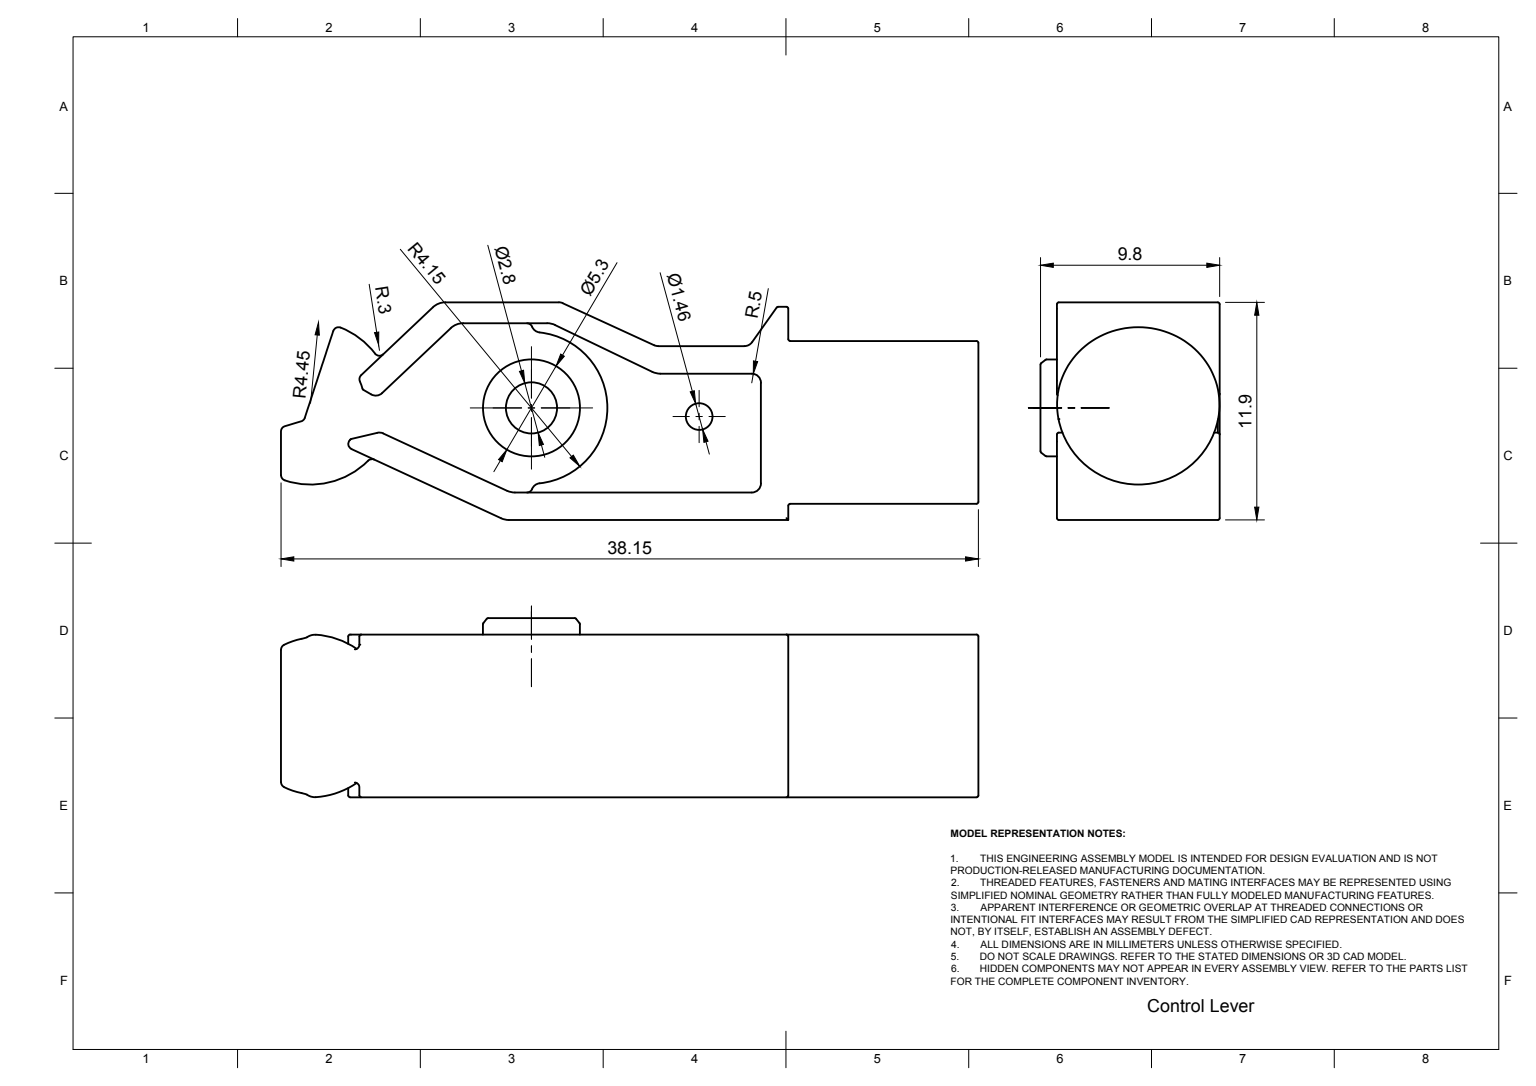
ISO-10303-21;
HEADER;
/* Generated by software containing ST-Developer
 * from STEP Tools, Inc. (www.steptools.com) 
 */

FILE_DESCRIPTION(
/* description */ ('STEP AP214'),
/* implementation_level */ '2;1');

FILE_NAME(
/* name */ 'Control Lever.step',
/* time_stamp */ '2026-10-06T00:19:40-07:00',
/* author */ (''),
/* organization */ (''),
/* preprocessor_version */ 'ST-DEVELOPER v20.2',
/* originating_system */ 'Autodesk Translation Framework v15.15.0.0',
/* authorisation */ '');

FILE_SCHEMA (('AUTOMOTIVE_DESIGN { 1 0 10303 214 3 1 1 }'));
ENDSEC;

DATA;
#10=MECHANICAL_DESIGN_GEOMETRIC_PRESENTATION_REPRESENTATION('',(#2068),#98302);
#51=(
BOUNDED_SURFACE()
B_SPLINE_SURFACE(2,2,((#79789,#79790,#79791),(#79792,#79793,#79794),(#79795,
#79796,#79797)),.UNSPECIFIED.,.F.,.F.,.F.)
B_SPLINE_SURFACE_WITH_KNOTS((3,3),(3,3),(-1.5707963267949,0.),(2.16840434497101E-15,
1.5707963267949),.UNSPECIFIED.)
GEOMETRIC_REPRESENTATION_ITEM()
RATIONAL_B_SPLINE_SURFACE(((1.,0.707106781186548,1.),(0.707106781186552,
0.500000000000004,0.707106781186552),(1.,0.707106781186548,1.)))
REPRESENTATION_ITEM('')
SURFACE()
);
#52=(
BOUNDED_SURFACE()
B_SPLINE_SURFACE(2,2,((#79805,#79806,#79807),(#79808,#79809,#79810),(#79811,
#79812,#79813)),.UNSPECIFIED.,.F.,.F.,.F.)
B_SPLINE_SURFACE_WITH_KNOTS((3,3),(3,3),(-1.5707963267949,0.),(-2.60208521396521E-15,
1.57079632679489),.UNSPECIFIED.)
GEOMETRIC_REPRESENTATION_ITEM()
RATIONAL_B_SPLINE_SURFACE(((1.,0.707106781186547,1.),(0.707106781186549,
0.500000000000001,0.707106781186549),(1.,0.707106781186547,1.)))
REPRESENTATION_ITEM('')
SURFACE()
);
#53=(
BOUNDED_SURFACE()
B_SPLINE_SURFACE(2,2,((#80188,#80189,#80190),(#80191,#80192,#80193),(#80194,
#80195,#80196)),.UNSPECIFIED.,.F.,.F.,.F.)
B_SPLINE_SURFACE_WITH_KNOTS((3,3),(3,3),(0.,1.4106605988315),(0.376263560334167,
1.46306115470143),.UNSPECIFIED.)
GEOMETRIC_REPRESENTATION_ITEM()
RATIONAL_B_SPLINE_SURFACE(((1.,0.855956286723383,1.),(0.761397465025631,
0.651722946883935,0.761397465025631),(1.,0.855956286723383,1.)))
REPRESENTATION_ITEM('')
SURFACE()
);
#54=(
BOUNDED_SURFACE()
B_SPLINE_SURFACE(2,2,((#80214,#80215,#80216),(#80217,#80218,#80219),(#80220,
#80221,#80222)),.UNSPECIFIED.,.F.,.F.,.F.)
B_SPLINE_SURFACE_WITH_KNOTS((3,3),(3,3),(0.,1.4106586369982),(-1.77013213181166E-11,
1.08679759433717),.UNSPECIFIED.)
GEOMETRIC_REPRESENTATION_ITEM()
RATIONAL_B_SPLINE_SURFACE(((1.,0.855956286726587,1.),(0.761398100939168,
0.651723491200565,0.761398100939168),(1.,0.855956286726587,1.)))
REPRESENTATION_ITEM('')
SURFACE()
);
#55=(
BOUNDED_SURFACE()
B_SPLINE_SURFACE(2,2,((#82289,#82290,#82291),(#82292,#82293,#82294),(#82295,
#82296,#82297)),.UNSPECIFIED.,.F.,.F.,.F.)
B_SPLINE_SURFACE_WITH_KNOTS((3,3),(3,3),(-1.5707963267949,0.),(-1.5707963267949,
-2.16840434497101E-15),.UNSPECIFIED.)
GEOMETRIC_REPRESENTATION_ITEM()
RATIONAL_B_SPLINE_SURFACE(((1.,0.707106781186548,1.),(0.707106781186552,
0.500000000000004,0.707106781186552),(1.,0.707106781186548,1.)))
REPRESENTATION_ITEM('')
SURFACE()
);
#56=(
BOUNDED_SURFACE()
B_SPLINE_SURFACE(2,2,((#82717,#82718,#82719),(#82720,#82721,#82722),(#82723,
#82724,#82725)),.UNSPECIFIED.,.F.,.F.,.F.)
B_SPLINE_SURFACE_WITH_KNOTS((3,3),(3,3),(-1.5707963267949,0.),(-1.57079632679489,
2.60208521396521E-15),.UNSPECIFIED.)
GEOMETRIC_REPRESENTATION_ITEM()
RATIONAL_B_SPLINE_SURFACE(((1.,0.707106781186547,1.),(0.707106781186549,
0.500000000000001,0.707106781186549),(1.,0.707106781186547,1.)))
REPRESENTATION_ITEM('')
SURFACE()
);
#57=(
BOUNDED_SURFACE()
B_SPLINE_SURFACE(2,2,((#82902,#82903,#82904),(#82905,#82906,#82907),(#82908,
#82909,#82910)),.UNSPECIFIED.,.F.,.F.,.F.)
B_SPLINE_SURFACE_WITH_KNOTS((3,3),(3,3),(0.,1.41065863634176),(-1.08679758944487,
1.77019687584094E-11),.UNSPECIFIED.)
GEOMETRIC_REPRESENTATION_ITEM()
RATIONAL_B_SPLINE_SURFACE(((1.,0.855956287991364,1.),(0.761398101151941,
0.651723492345688,0.761398101151941),(1.,0.855956287991364,1.)))
REPRESENTATION_ITEM('')
SURFACE()
);
#58=(
BOUNDED_SURFACE()
B_SPLINE_SURFACE(2,2,((#83156,#83157,#83158),(#83159,#83160,#83161),(#83162,
#83163,#83164)),.UNSPECIFIED.,.F.,.F.,.F.)
B_SPLINE_SURFACE_WITH_KNOTS((3,3),(3,3),(0.,1.41066059181116),(-1.46306115470144,
-0.376263565240401),.UNSPECIFIED.)
GEOMETRIC_REPRESENTATION_ITEM()
RATIONAL_B_SPLINE_SURFACE(((1.,0.855956287991761,1.),(0.761397467301222,
0.651722949797482,0.761397467301222),(1.,0.855956287991761,1.)))
REPRESENTATION_ITEM('')
SURFACE()
);
#138=TOROIDAL_SURFACE('',#35727,4.25458972174,0.3);
#139=TOROIDAL_SURFACE('',#35732,4.40145759978,0.3);
#140=TOROIDAL_SURFACE('',#35739,4.72461821943,0.3);
#141=TOROIDAL_SURFACE('',#35746,4.40145759978,0.3);
#142=TOROIDAL_SURFACE('',#35752,4.25458972174,0.3);
#143=TOROIDAL_SURFACE('',#35757,4.1423251838,0.3);
#144=TOROIDAL_SURFACE('',#35772,4.00032353732,0.3);
#145=TOROIDAL_SURFACE('',#35791,4.00032353732,0.3);
#146=TOROIDAL_SURFACE('',#35793,3.93623398426,0.3);
#147=TOROIDAL_SURFACE('',#35806,1.3,0.3);
#148=TOROIDAL_SURFACE('',#35819,4.45,0.3);
#149=TOROIDAL_SURFACE('',#35846,0.9,0.1);
#150=TOROIDAL_SURFACE('',#35851,0.6,0.1);
#151=TOROIDAL_SURFACE('',#35856,0.6,0.1);
#152=TOROIDAL_SURFACE('',#35874,3.85,0.3);
#153=TOROIDAL_SURFACE('',#35880,1.1,0.1);
#154=TOROIDAL_SURFACE('',#35901,4.15601973046,0.3);
#155=TOROIDAL_SURFACE('',#35912,0.7,0.3);
#156=TOROIDAL_SURFACE('',#35915,1.1,0.1);
#157=TOROIDAL_SURFACE('',#35927,0.8,0.3);
#158=TOROIDAL_SURFACE('',#35929,0.8,0.3);
#159=TOROIDAL_SURFACE('',#35933,0.9,0.1);
#160=TOROIDAL_SURFACE('',#35938,0.2,0.1);
#161=TOROIDAL_SURFACE('',#35941,3.05,0.1);
#162=TOROIDAL_SURFACE('',#35947,0.4,0.1);
#163=TOROIDAL_SURFACE('',#35951,1.1,0.1);
#164=TOROIDAL_SURFACE('',#35955,0.4,0.1);
#165=TOROIDAL_SURFACE('',#35960,3.05,0.1);
#166=TOROIDAL_SURFACE('',#35964,0.2,0.1);
#167=TOROIDAL_SURFACE('',#35969,0.9,0.1);
#168=TOROIDAL_SURFACE('',#35974,0.4,0.1);
#169=TOROIDAL_SURFACE('',#35979,0.6,0.1);
#170=TOROIDAL_SURFACE('',#35984,0.6,0.1);
#171=TOROIDAL_SURFACE('',#35995,0.2,0.1);
#172=TOROIDAL_SURFACE('',#36006,0.2,0.1);
#173=TOROIDAL_SURFACE('',#36010,2.95,0.3);
#174=TOROIDAL_SURFACE('',#36014,0.7,0.3);
#175=TOROIDAL_SURFACE('',#36016,2.65,0.3);
#176=TOROIDAL_SURFACE('',#36021,2.65,0.3);
#177=TOROIDAL_SURFACE('',#36027,2.65,0.3);
#178=TOROIDAL_SURFACE('',#36031,2.65,0.3);
#179=TOROIDAL_SURFACE('',#36042,0.8,0.3);
#180=TOROIDAL_SURFACE('',#36048,3.98150447852,0.3);
#181=TOROIDAL_SURFACE('',#36055,4.46095497424,0.3);
#182=TOROIDAL_SURFACE('',#36106,3.05,0.1);
#183=TOROIDAL_SURFACE('',#36112,4.15601973046,0.3);
#184=TOROIDAL_SURFACE('',#36135,0.9,0.1);
#185=TOROIDAL_SURFACE('',#36140,0.2,0.1);
#186=TOROIDAL_SURFACE('',#36143,0.2,0.1);
#187=TOROIDAL_SURFACE('',#36148,0.9,0.1);
#188=TOROIDAL_SURFACE('',#36153,0.4,0.1);
#189=TOROIDAL_SURFACE('',#36158,0.6,0.1);
#190=TOROIDAL_SURFACE('',#36163,0.6,0.1);
#191=TOROIDAL_SURFACE('',#36178,0.2,0.1);
#192=TOROIDAL_SURFACE('',#36193,0.2,0.1);
#193=TOROIDAL_SURFACE('',#36206,2.95,0.3);
#194=TOROIDAL_SURFACE('',#36212,0.7,0.3);
#195=TOROIDAL_SURFACE('',#36215,0.7,0.3);
#196=TOROIDAL_SURFACE('',#36220,0.8,0.3);
#197=TOROIDAL_SURFACE('',#36229,0.8,0.3);
#198=TOROIDAL_SURFACE('',#36233,0.8,0.3);
#199=TOROIDAL_SURFACE('',#36237,3.85,0.3);
#200=TOROIDAL_SURFACE('',#36240,2.36684105319,0.1);
#201=TOROIDAL_SURFACE('',#36253,0.4,0.1);
#202=TOROIDAL_SURFACE('',#36259,1.1,0.1);
#203=TOROIDAL_SURFACE('',#36268,3.98150447852,0.3);
#204=TOROIDAL_SURFACE('',#36272,2.55,0.1);
#205=TOROIDAL_SURFACE('',#36276,1.3,0.3);
#206=TOROIDAL_SURFACE('',#36292,1.1,0.1);
#207=TOROIDAL_SURFACE('',#36306,3.05,0.1);
#208=TOROIDAL_SURFACE('',#36312,0.4,0.1);
#209=TOROIDAL_SURFACE('',#36320,0.6,0.1);
#210=TOROIDAL_SURFACE('',#36325,0.6,0.1);
#211=TOROIDAL_SURFACE('',#36330,0.9,0.1);
#212=TOROIDAL_SURFACE('',#36335,1.1,0.1);
#213=TOROIDAL_SURFACE('',#36363,4.45,0.3);
#606=ELLIPSE('',#35728,0.35400824521659,0.325120639664921);
#607=ELLIPSE('',#35730,0.26079295230188,0.225428549013028);
#608=ELLIPSE('',#35733,0.298959427554072,0.296143919662364);
#609=ELLIPSE('',#35753,0.260785485861866,0.225415709617204);
#610=ELLIPSE('',#35755,0.354058541716697,0.325144371990916);
#611=ELLIPSE('',#35805,0.298848922732419,0.296905432652653);
#612=ELLIPSE('',#35824,0.298891660055286,0.297093982021653);
#613=ELLIPSE('',#35833,0.298979043963965,0.297433001748831);
#614=ELLIPSE('',#35835,0.298894659298114,0.297106043484314);
#615=ELLIPSE('',#35836,0.298977328382314,0.297429112568373);
#616=ELLIPSE('',#35932,0.14142135623731,0.1);
#617=ELLIPSE('',#36133,0.14142135623731,0.1);
#618=ELLIPSE('',#36348,0.298848922836507,0.296905432909967);
#619=ELLIPSE('',#36349,0.298979123737475,0.29743317011586);
#620=ELLIPSE('',#36360,0.298979307954305,0.297433587262778);
#621=ELLIPSE('',#36361,0.298894247034695,0.297105377501926);
#622=ELLIPSE('',#36365,0.298891932661897,0.29709461276469);
#623=ELLIPSE('',#36366,0.298848892860348,0.296905360884096);
#736=SPHERICAL_SURFACE('',#35769,0.3);
#737=SPHERICAL_SURFACE('',#35775,4.45);
#738=SPHERICAL_SURFACE('',#35788,0.3);
#739=SPHERICAL_SURFACE('',#35899,0.3);
#740=SPHERICAL_SURFACE('',#36036,0.3);
#741=SPHERICAL_SURFACE('',#36040,0.3);
#742=SPHERICAL_SURFACE('',#36047,0.3);
#743=SPHERICAL_SURFACE('',#36063,0.1);
#744=SPHERICAL_SURFACE('',#36068,0.1);
#745=SPHERICAL_SURFACE('',#36086,0.1);
#746=SPHERICAL_SURFACE('',#36089,0.1);
#747=SPHERICAL_SURFACE('',#36095,0.1);
#748=SPHERICAL_SURFACE('',#36098,0.1);
#749=SPHERICAL_SURFACE('',#36126,0.3);
#750=SPHERICAL_SURFACE('',#36199,0.1);
#751=SPHERICAL_SURFACE('',#36223,0.3);
#752=SPHERICAL_SURFACE('',#36227,0.3);
#753=SPHERICAL_SURFACE('',#36245,0.1);
#754=SPHERICAL_SURFACE('',#36246,0.1);
#755=SPHERICAL_SURFACE('',#36247,0.1);
#756=SPHERICAL_SURFACE('',#36248,0.1);
#757=SPHERICAL_SURFACE('',#36265,0.3);
#758=SPHERICAL_SURFACE('',#36308,0.1);
#1156=B_SPLINE_SURFACE_WITH_KNOTS('',5,5,((#79194,#79195,#79196,#79197,
#79198,#79199),(#79200,#79201,#79202,#79203,#79204,#79205),(#79206,#79207,
#79208,#79209,#79210,#79211),(#79212,#79213,#79214,#79215,#79216,#79217),
(#79218,#79219,#79220,#79221,#79222,#79223),(#79224,#79225,#79226,#79227,
#79228,#79229)),.UNSPECIFIED.,.F.,.F.,.F.,(6,6),(6,6),(1.91917304179,2.64214133457),
(0.,0.3),.UNSPECIFIED.);
#1157=B_SPLINE_SURFACE_WITH_KNOTS('',5,5,((#79714,#79715,#79716,#79717,
#79718,#79719),(#79720,#79721,#79722,#79723,#79724,#79725),(#79726,#79727,
#79728,#79729,#79730,#79731),(#79732,#79733,#79734,#79735,#79736,#79737),
(#79738,#79739,#79740,#79741,#79742,#79743),(#79744,#79745,#79746,#79747,
#79748,#79749)),.UNSPECIFIED.,.F.,.F.,.F.,(6,6),(6,6),(1.95117092983,2.67415250918),
(0.,0.3),.UNSPECIFIED.);
#1158=B_SPLINE_SURFACE_WITH_KNOTS('',5,5,((#79924,#79925,#79926,#79927,
#79928,#79929),(#79930,#79931,#79932,#79933,#79934,#79935),(#79936,#79937,
#79938,#79939,#79940,#79941),(#79942,#79943,#79944,#79945,#79946,#79947),
(#79948,#79949,#79950,#79951,#79952,#79953),(#79954,#79955,#79956,#79957,
#79958,#79959)),.UNSPECIFIED.,.F.,.F.,.F.,(6,6),(6,6),(1.62679171178,4.14575432942),
(0.,0.3),.UNSPECIFIED.);
#1159=B_SPLINE_SURFACE_WITH_KNOTS('',5,5,((#79981,#79982,#79983,#79984,
#79985,#79986),(#79987,#79988,#79989,#79990,#79991,#79992),(#79993,#79994,
#79995,#79996,#79997,#79998),(#79999,#80000,#80001,#80002,#80003,#80004),
(#80005,#80006,#80007,#80008,#80009,#80010),(#80011,#80012,#80013,#80014,
#80015,#80016)),.UNSPECIFIED.,.F.,.F.,.F.,(6,6),(6,6),(5.20521075808,6.00042817873),
(0.,0.3),.UNSPECIFIED.);
#1160=B_SPLINE_SURFACE_WITH_KNOTS('',5,5,((#80093,#80094,#80095,#80096,
#80097,#80098),(#80099,#80100,#80101,#80102,#80103,#80104),(#80105,#80106,
#80107,#80108,#80109,#80110),(#80111,#80112,#80113,#80114,#80115,#80116),
(#80117,#80118,#80119,#80120,#80121,#80122),(#80123,#80124,#80125,#80126,
#80127,#80128)),.UNSPECIFIED.,.F.,.F.,.F.,(6,6),(6,6),(5.20484021909,5.76063633602),
(0.,0.3),.UNSPECIFIED.);
#1161=B_SPLINE_SURFACE_WITH_KNOTS('',5,5,((#80139,#80140,#80141,#80142,
#80143,#80144),(#80145,#80146,#80147,#80148,#80149,#80150),(#80151,#80152,
#80153,#80154,#80155,#80156),(#80157,#80158,#80159,#80160,#80161,#80162),
(#80163,#80164,#80165,#80166,#80167,#80168),(#80169,#80170,#80171,#80172,
#80173,#80174)),.UNSPECIFIED.,.F.,.F.,.F.,(6,6),(6,6),(1.9878298196,2.53578324996),
(0.,0.3),.UNSPECIFIED.);
#1162=B_SPLINE_SURFACE_WITH_KNOTS('',5,5,((#80264,#80265,#80266,#80267,
#80268,#80269),(#80270,#80271,#80272,#80273,#80274,#80275),(#80276,#80277,
#80278,#80279,#80280,#80281),(#80282,#80283,#80284,#80285,#80286,#80287),
(#80288,#80289,#80290,#80291,#80292,#80293),(#80294,#80295,#80296,#80297,
#80298,#80299),(#80300,#80301,#80302,#80303,#80304,#80305),(#80306,#80307,
#80308,#80309,#80310,#80311),(#80312,#80313,#80314,#80315,#80316,#80317)),
 .UNSPECIFIED.,.F.,.F.,.F.,(6,3,6),(6,6),(3.54900880514,4.18701109461,4.71575303852),
(0.,0.3),.UNSPECIFIED.);
#1163=B_SPLINE_SURFACE_WITH_KNOTS('',5,5,((#80403,#80404,#80405,#80406,
#80407,#80408),(#80409,#80410,#80411,#80412,#80413,#80414),(#80415,#80416,
#80417,#80418,#80419,#80420),(#80421,#80422,#80423,#80424,#80425,#80426),
(#80427,#80428,#80429,#80430,#80431,#80432),(#80433,#80434,#80435,#80436,
#80437,#80438),(#80439,#80440,#80441,#80442,#80443,#80444),(#80445,#80446,
#80447,#80448,#80449,#80450),(#80451,#80452,#80453,#80454,#80455,#80456)),
 .UNSPECIFIED.,.F.,.F.,.F.,(6,3,6),(6,6),(3.54900880515,4.18701109461,4.71575303852),
(0.,0.3),.UNSPECIFIED.);
#1164=B_SPLINE_SURFACE_WITH_KNOTS('',5,5,((#80828,#80829,#80830,#80831,
#80832,#80833),(#80834,#80835,#80836,#80837,#80838,#80839),(#80840,#80841,
#80842,#80843,#80844,#80845),(#80846,#80847,#80848,#80849,#80850,#80851),
(#80852,#80853,#80854,#80855,#80856,#80857),(#80858,#80859,#80860,#80861,
#80862,#80863)),.UNSPECIFIED.,.F.,.F.,.F.,(6,6),(6,6),(3.53583307557,4.36798756241),
(0.,0.3),.UNSPECIFIED.);
#1165=B_SPLINE_SURFACE_WITH_KNOTS('',5,5,((#80907,#80908,#80909,#80910,
#80911,#80912,#80913,#80914,#80915),(#80916,#80917,#80918,#80919,#80920,
#80921,#80922,#80923,#80924),(#80925,#80926,#80927,#80928,#80929,#80930,
#80931,#80932,#80933),(#80934,#80935,#80936,#80937,#80938,#80939,#80940,
#80941,#80942),(#80943,#80944,#80945,#80946,#80947,#80948,#80949,#80950,
#80951),(#80952,#80953,#80954,#80955,#80956,#80957,#80958,#80959,#80960),
(#80961,#80962,#80963,#80964,#80965,#80966,#80967,#80968,#80969),(#80970,
#80971,#80972,#80973,#80974,#80975,#80976,#80977,#80978),(#80979,#80980,
#80981,#80982,#80983,#80984,#80985,#80986,#80987)),.UNSPECIFIED.,.F.,.F.,
 .F.,(6,3,6),(6,3,6),(1.97024157714,2.85861157082,3.64197819698),(0.,0.15,
0.3),.UNSPECIFIED.);
#1166=B_SPLINE_SURFACE_WITH_KNOTS('',5,5,((#81069,#81070,#81071,#81072,
#81073,#81074,#81075,#81076,#81077),(#81078,#81079,#81080,#81081,#81082,
#81083,#81084,#81085,#81086),(#81087,#81088,#81089,#81090,#81091,#81092,
#81093,#81094,#81095),(#81096,#81097,#81098,#81099,#81100,#81101,#81102,
#81103,#81104),(#81105,#81106,#81107,#81108,#81109,#81110,#81111,#81112,
#81113),(#81114,#81115,#81116,#81117,#81118,#81119,#81120,#81121,#81122),
(#81123,#81124,#81125,#81126,#81127,#81128,#81129,#81130,#81131),(#81132,
#81133,#81134,#81135,#81136,#81137,#81138,#81139,#81140),(#81141,#81142,
#81143,#81144,#81145,#81146,#81147,#81148,#81149)),.UNSPECIFIED.,.F.,.F.,
 .F.,(6,3,6),(6,3,6),(1.91124469448,2.8398573808,3.58302582769),(0.,0.15,
0.3),.UNSPECIFIED.);
#1167=B_SPLINE_SURFACE_WITH_KNOTS('',5,5,((#81243,#81244,#81245,#81246,
#81247,#81248),(#81249,#81250,#81251,#81252,#81253,#81254),(#81255,#81256,
#81257,#81258,#81259,#81260),(#81261,#81262,#81263,#81264,#81265,#81266),
(#81267,#81268,#81269,#81270,#81271,#81272),(#81273,#81274,#81275,#81276,
#81277,#81278),(#81279,#81280,#81281,#81282,#81283,#81284),(#81285,#81286,
#81287,#81288,#81289,#81290),(#81291,#81292,#81293,#81294,#81295,#81296)),
 .UNSPECIFIED.,.F.,.F.,.F.,(6,3,6),(6,6),(0.109166698395,1.13023412606,
2.1197288877),(0.,0.3),.UNSPECIFIED.);
#1168=B_SPLINE_SURFACE_WITH_KNOTS('',5,5,((#81385,#81386,#81387,#81388,
#81389,#81390,#81391,#81392,#81393),(#81394,#81395,#81396,#81397,#81398,
#81399,#81400,#81401,#81402),(#81403,#81404,#81405,#81406,#81407,#81408,
#81409,#81410,#81411),(#81412,#81413,#81414,#81415,#81416,#81417,#81418,
#81419,#81420),(#81421,#81422,#81423,#81424,#81425,#81426,#81427,#81428,
#81429),(#81430,#81431,#81432,#81433,#81434,#81435,#81436,#81437,#81438),
(#81439,#81440,#81441,#81442,#81443,#81444,#81445,#81446,#81447),(#81448,
#81449,#81450,#81451,#81452,#81453,#81454,#81455,#81456),(#81457,#81458,
#81459,#81460,#81461,#81462,#81463,#81464,#81465)),.UNSPECIFIED.,.F.,.F.,
 .F.,(6,3,6),(6,3,6),(2.21471914028,2.64235434316,3.16496476901),(0.,0.15,
0.3),.UNSPECIFIED.);
#1169=B_SPLINE_SURFACE_WITH_KNOTS('',5,5,((#81523,#81524,#81525,#81526,
#81527,#81528,#81529,#81530,#81531),(#81532,#81533,#81534,#81535,#81536,
#81537,#81538,#81539,#81540),(#81541,#81542,#81543,#81544,#81545,#81546,
#81547,#81548,#81549),(#81550,#81551,#81552,#81553,#81554,#81555,#81556,
#81557,#81558),(#81559,#81560,#81561,#81562,#81563,#81564,#81565,#81566,
#81567),(#81568,#81569,#81570,#81571,#81572,#81573,#81574,#81575,#81576),
(#81577,#81578,#81579,#81580,#81581,#81582,#81583,#81584,#81585),(#81586,
#81587,#81588,#81589,#81590,#81591,#81592,#81593,#81594),(#81595,#81596,
#81597,#81598,#81599,#81600,#81601,#81602,#81603)),.UNSPECIFIED.,.F.,.F.,
 .F.,(6,3,6),(6,3,6),(2.20468600976,2.64437519712,3.15494946669),(0.,0.15,
0.3),.UNSPECIFIED.);
#1170=B_SPLINE_SURFACE_WITH_KNOTS('',5,5,((#81743,#81744,#81745,#81746,
#81747,#81748,#81749,#81750,#81751),(#81752,#81753,#81754,#81755,#81756,
#81757,#81758,#81759,#81760),(#81761,#81762,#81763,#81764,#81765,#81766,
#81767,#81768,#81769),(#81770,#81771,#81772,#81773,#81774,#81775,#81776,
#81777,#81778),(#81779,#81780,#81781,#81782,#81783,#81784,#81785,#81786,
#81787),(#81788,#81789,#81790,#81791,#81792,#81793,#81794,#81795,#81796)),
 .UNSPECIFIED.,.F.,.F.,.F.,(6,6),(6,3,6),(1.4421658125425,1.77233951315641),
(-0.000123951336412412,0.15,0.3),.UNSPECIFIED.);
#1171=B_SPLINE_SURFACE_WITH_KNOTS('',5,5,((#81842,#81843,#81844,#81845,
#81846,#81847),(#81848,#81849,#81850,#81851,#81852,#81853),(#81854,#81855,
#81856,#81857,#81858,#81859),(#81860,#81861,#81862,#81863,#81864,#81865),
(#81866,#81867,#81868,#81869,#81870,#81871),(#81872,#81873,#81874,#81875,
#81876,#81877)),.UNSPECIFIED.,.F.,.F.,.F.,(6,6),(6,6),(1.49467475321184,
1.75483909752735),(-4.40481773546895E-5,0.3),.UNSPECIFIED.);
#1172=B_SPLINE_SURFACE_WITH_KNOTS('',5,5,((#81898,#81899,#81900,#81901,
#81902,#81903,#81904,#81905,#81906),(#81907,#81908,#81909,#81910,#81911,
#81912,#81913,#81914,#81915),(#81916,#81917,#81918,#81919,#81920,#81921,
#81922,#81923,#81924),(#81925,#81926,#81927,#81928,#81929,#81930,#81931,
#81932,#81933),(#81934,#81935,#81936,#81937,#81938,#81939,#81940,#81941,
#81942),(#81943,#81944,#81945,#81946,#81947,#81948,#81949,#81950,#81951)),
 .UNSPECIFIED.,.F.,.F.,.F.,(6,6),(6,3,6),(1.40783636987619,1.73804585327402),
(-0.000127187184019683,0.15,0.3),.UNSPECIFIED.);
#1173=B_SPLINE_SURFACE_WITH_KNOTS('',5,5,((#81966,#81967,#81968,#81969,
#81970,#81971),(#81972,#81973,#81974,#81975,#81976,#81977),(#81978,#81979,
#81980,#81981,#81982,#81983),(#81984,#81985,#81986,#81987,#81988,#81989),
(#81990,#81991,#81992,#81993,#81994,#81995),(#81996,#81997,#81998,#81999,
#82000,#82001)),.UNSPECIFIED.,.F.,.F.,.F.,(6,6),(6,6),(1.54690812238987,
1.80703488607013),(-4.43625301270991E-5,0.3),.UNSPECIFIED.);
#1174=B_SPLINE_SURFACE_WITH_KNOTS('',5,5,((#82309,#82310,#82311,#82312,
#82313,#82314),(#82315,#82316,#82317,#82318,#82319,#82320),(#82321,#82322,
#82323,#82324,#82325,#82326),(#82327,#82328,#82329,#82330,#82331,#82332),
(#82333,#82334,#82335,#82336,#82337,#82338),(#82339,#82340,#82341,#82342,
#82343,#82344),(#82345,#82346,#82347,#82348,#82349,#82350),(#82351,#82352,
#82353,#82354,#82355,#82356),(#82357,#82358,#82359,#82360,#82361,#82362)),
 .UNSPECIFIED.,.F.,.F.,.F.,(6,3,6),(6,6),(3.01269951131,3.90600477275,5.02326603963),
(0.,0.3),.UNSPECIFIED.);
#1175=B_SPLINE_SURFACE_WITH_KNOTS('',5,5,((#82489,#82490,#82491,#82492,
#82493,#82494),(#82495,#82496,#82497,#82498,#82499,#82500),(#82501,#82502,
#82503,#82504,#82505,#82506),(#82507,#82508,#82509,#82510,#82511,#82512),
(#82513,#82514,#82515,#82516,#82517,#82518),(#82519,#82520,#82521,#82522,
#82523,#82524)),.UNSPECIFIED.,.F.,.F.,.F.,(6,6),(6,6),(6.50394744106137,
7.33762762903),(-0.00162956260388768,0.301629563228629),.UNSPECIFIED.);
#1176=B_SPLINE_SURFACE_WITH_KNOTS('',5,5,((#82733,#82734,#82735,#82736,
#82737,#82738),(#82739,#82740,#82741,#82742,#82743,#82744),(#82745,#82746,
#82747,#82748,#82749,#82750),(#82751,#82752,#82753,#82754,#82755,#82756),
(#82757,#82758,#82759,#82760,#82761,#82762),(#82763,#82764,#82765,#82766,
#82767,#82768)),.UNSPECIFIED.,.F.,.F.,.F.,(6,6),(6,6),(5.20521075808,6.00042817873),
(0.,0.3),.UNSPECIFIED.);
#1177=B_SPLINE_SURFACE_WITH_KNOTS('',5,5,((#82781,#82782,#82783,#82784,
#82785,#82786),(#82787,#82788,#82789,#82790,#82791,#82792),(#82793,#82794,
#82795,#82796,#82797,#82798),(#82799,#82800,#82801,#82802,#82803,#82804),
(#82805,#82806,#82807,#82808,#82809,#82810),(#82811,#82812,#82813,#82814,
#82815,#82816),(#82817,#82818,#82819,#82820,#82821,#82822),(#82823,#82824,
#82825,#82826,#82827,#82828),(#82829,#82830,#82831,#82832,#82833,#82834)),
 .UNSPECIFIED.,.F.,.F.,.F.,(6,3,6),(6,6),(3.54900880514,4.18701109461,4.71575303852),
(0.,0.3),.UNSPECIFIED.);
#1178=B_SPLINE_SURFACE_WITH_KNOTS('',5,5,((#82991,#82992,#82993,#82994,
#82995,#82996),(#82997,#82998,#82999,#83000,#83001,#83002),(#83003,#83004,
#83005,#83006,#83007,#83008),(#83009,#83010,#83011,#83012,#83013,#83014),
(#83015,#83016,#83017,#83018,#83019,#83020),(#83021,#83022,#83023,#83024,
#83025,#83026)),.UNSPECIFIED.,.F.,.F.,.F.,(6,6),(6,6),(5.20484021909,5.76063633602),
(0.,0.3),.UNSPECIFIED.);
#1179=B_SPLINE_SURFACE_WITH_KNOTS('',5,5,((#83038,#83039,#83040,#83041,
#83042,#83043),(#83044,#83045,#83046,#83047,#83048,#83049),(#83050,#83051,
#83052,#83053,#83054,#83055),(#83056,#83057,#83058,#83059,#83060,#83061),
(#83062,#83063,#83064,#83065,#83066,#83067),(#83068,#83069,#83070,#83071,
#83072,#83073),(#83074,#83075,#83076,#83077,#83078,#83079),(#83080,#83081,
#83082,#83083,#83084,#83085),(#83086,#83087,#83088,#83089,#83090,#83091)),
 .UNSPECIFIED.,.F.,.F.,.F.,(6,3,6),(6,6),(3.54900880515,4.18701109461,4.71575303852),
(0.,0.3),.UNSPECIFIED.);
#1180=B_SPLINE_SURFACE_WITH_KNOTS('',5,5,((#83204,#83205,#83206,#83207,
#83208,#83209),(#83210,#83211,#83212,#83213,#83214,#83215),(#83216,#83217,
#83218,#83219,#83220,#83221),(#83222,#83223,#83224,#83225,#83226,#83227),
(#83228,#83229,#83230,#83231,#83232,#83233),(#83234,#83235,#83236,#83237,
#83238,#83239)),.UNSPECIFIED.,.F.,.F.,.F.,(6,6),(6,6),(1.9878298196,2.53578324996),
(0.,0.3),.UNSPECIFIED.);
#1181=B_SPLINE_SURFACE_WITH_KNOTS('',5,5,((#83241,#83242,#83243,#83244,
#83245,#83246),(#83247,#83248,#83249,#83250,#83251,#83252),(#83253,#83254,
#83255,#83256,#83257,#83258),(#83259,#83260,#83261,#83262,#83263,#83264),
(#83265,#83266,#83267,#83268,#83269,#83270),(#83271,#83272,#83273,#83274,
#83275,#83276)),.UNSPECIFIED.,.F.,.F.,.F.,(6,6),(6,6),(1.62679171178,4.14575432942),
(0.,0.3),.UNSPECIFIED.);
#1295=FACE_BOUND('',#6322,.T.);
#1296=FACE_BOUND('',#6330,.T.);
#1297=FACE_BOUND('',#6375,.T.);
#1298=FACE_BOUND('',#6481,.T.);
#1299=FACE_BOUND('',#6516,.T.);
#1300=FACE_BOUND('',#6551,.T.);
#1763=B_SPLINE_CURVE_WITH_KNOTS('',5,(#78627,#78628,#78629,#78630,#78631,
#78632),.UNSPECIFIED.,.F.,.F.,(6,6),(0.226923016970762,1.),
 .UNSPECIFIED.);
#1764=B_SPLINE_CURVE_WITH_KNOTS('',3,(#78640,#78641,#78642,#78643,#78644,
#78645),.UNSPECIFIED.,.F.,.F.,(4,2,4),(0.226811293541348,0.613405646770674,
1.),.UNSPECIFIED.);
#1765=B_SPLINE_CURVE_WITH_KNOTS('',3,(#78678,#78679,#78680,#78681,#78682,
#78683),.UNSPECIFIED.,.F.,.F.,(4,2,4),(0.197042714657638,0.598521357328819,
1.),.UNSPECIFIED.);
#1766=B_SPLINE_CURVE_WITH_KNOTS('',3,(#78696,#78697,#78698,#78699,#78700,
#78701),.UNSPECIFIED.,.F.,.F.,(4,2,4),(0.226811293549919,0.61340564677496,
1.),.UNSPECIFIED.);
#1767=B_SPLINE_CURVE_WITH_KNOTS('',5,(#78705,#78706,#78707,#78708,#78709,
#78710),.UNSPECIFIED.,.F.,.F.,(6,6),(0.226923156363992,1.),
 .UNSPECIFIED.);
#1768=B_SPLINE_CURVE_WITH_KNOTS('',5,(#78719,#78720,#78721,#78722,#78723,
#78724),.UNSPECIFIED.,.F.,.F.,(6,6),(0.,1.),.UNSPECIFIED.);
#1769=B_SPLINE_CURVE_WITH_KNOTS('',3,(#78728,#78729,#78730,#78731,#78732,
#78733,#78734,#78735,#78736,#78737,#78738,#78739,#78740,#78741,#78742,#78743,
#78744,#78745,#78746,#78747,#78748,#78749,#78750,#78751,#78752,#78753,#78754,
#78755,#78756,#78757,#78758,#78759,#78760,#78761,#78762,#78763,#78764,#78765,
#78766,#78767,#78768,#78769,#78770,#78771,#78772,#78773,#78774,#78775,#78776,
#78777,#78778,#78779,#78780,#78781,#78782,#78783,#78784,#78785,#78786,#78787,
#78788,#78789,#78790,#78791,#78792,#78793,#78794,#78795,#78796,#78797,#78798,
#78799,#78800,#78801,#78802,#78803,#78804,#78805,#78806,#78807,#78808,#78809,
#78810,#78811,#78812,#78813,#78814,#78815,#78816,#78817,#78818,#78819,#78820,
#78821,#78822,#78823,#78824,#78825,#78826,#78827,#78828,#78829,#78830,#78831,
#78832,#78833,#78834,#78835,#78836,#78837,#78838,#78839,#78840,#78841,#78842,
#78843,#78844,#78845,#78846,#78847,#78848,#78849,#78850,#78851,#78852,#78853,
#78854,#78855,#78856,#78857,#78858,#78859,#78860,#78861,#78862,#78863,#78864,
#78865,#78866,#78867,#78868,#78869,#78870,#78871,#78872,#78873,#78874,#78875,
#78876,#78877,#78878,#78879,#78880,#78881,#78882,#78883,#78884,#78885,#78886,
#78887,#78888,#78889,#78890,#78891,#78892,#78893,#78894,#78895,#78896,#78897,
#78898,#78899,#78900,#78901,#78902,#78903,#78904,#78905,#78906,#78907,#78908,
#78909,#78910,#78911,#78912,#78913,#78914,#78915,#78916,#78917,#78918,#78919,
#78920,#78921,#78922,#78923,#78924,#78925,#78926,#78927,#78928,#78929,#78930,
#78931,#78932,#78933,#78934,#78935,#78936,#78937,#78938,#78939,#78940,#78941,
#78942,#78943,#78944,#78945,#78946,#78947),.UNSPECIFIED.,.F.,.F.,(4,3,3,
3,3,3,3,3,3,3,3,3,3,3,3,3,3,3,3,3,3,3,3,3,3,3,3,3,3,3,3,3,3,3,3,3,3,3,3,
3,3,3,3,3,3,3,3,3,3,3,3,3,3,3,3,3,3,3,3,3,3,3,3,3,3,3,3,3,3,3,3,3,3,4),
(0.0868385867057379,0.0937499999999956,0.109374999999995,0.117187499999994,
0.121093749999994,0.123046874999994,0.124023437499994,0.124999999999994,
0.145934913493643,0.167462598467453,0.187499999999996,0.209872497695248,
0.218749999999997,0.234374999999997,0.242187499999998,0.246093749999998,
0.248046874999998,0.249023437499998,0.249999999999998,0.272528330630081,
0.29564318505803,0.312499999999998,0.336432597942232,0.343749999999998,
0.359374999999998,0.367187499999998,0.371093749999998,0.373046874999998,
0.374851354279564,0.374999999999998,0.398493781362424,0.406249999999999,
0.421874999999999,0.429687499999999,0.433593749999999,0.436607414249363,
0.437499999999999,0.461739947182365,0.468749999999999,0.484374999999999,
0.492187499999999,0.497333394583601,0.499999999999998,0.525206949984025,
0.551256701035308,0.562499999999999,0.591346920143275,0.593749999999999,
0.609375,0.6171875,0.622302819166279,0.625,0.65625,0.6875,0.716247216753145,
0.71875,0.734375,0.7421875,0.747756676868899,0.75,0.778803250902111,0.78125,
0.798733322246778,0.8125,0.840832577832501,0.84375,0.859375,0.868597898855189,
0.875,0.903754289572031,0.93251341058128,0.961094429961356,0.989185606847336,
1.),.UNSPECIFIED.);
#1770=B_SPLINE_CURVE_WITH_KNOTS('',3,(#78949,#78950,#78951,#78952,#78953,
#78954,#78955,#78956,#78957,#78958,#78959,#78960,#78961,#78962,#78963,#78964,
#78965,#78966,#78967,#78968,#78969,#78970,#78971,#78972,#78973,#78974,#78975,
#78976,#78977,#78978,#78979,#78980,#78981,#78982,#78983,#78984,#78985,#78986,
#78987,#78988,#78989,#78990,#78991),.UNSPECIFIED.,.F.,.F.,(4,3,3,3,3,3,
3,3,3,3,3,3,3,3,4),(0.,0.00951856234533963,0.0190261223058877,0.0285057566012048,
0.0312499999999986,0.0406555969248241,0.0468749999999981,0.0546874999999978,
0.0585937499999976,0.0605468749999976,0.0615234374999975,0.0624213299799009,
0.0624999999999974,0.0778317290989469,0.0868385867057379),.UNSPECIFIED.);
#1771=B_SPLINE_CURVE_WITH_KNOTS('',3,(#79000,#79001,#79002,#79003,#79004,
#79005,#79006,#79007,#79008,#79009,#79010,#79011,#79012,#79013,#79014,#79015,
#79016,#79017,#79018,#79019,#79020,#79021,#79022,#79023,#79024,#79025,#79026,
#79027,#79028,#79029,#79030,#79031,#79032,#79033,#79034,#79035,#79036,#79037,
#79038,#79039,#79040,#79041,#79042,#79043,#79044,#79045,#79046,#79047,#79048,
#79049,#79050,#79051,#79052,#79053,#79054,#79055,#79056,#79057,#79058,#79059,
#79060,#79061,#79062,#79063,#79064,#79065,#79066),.UNSPECIFIED.,.F.,.F.,
(4,3,3,3,3,3,3,3,3,3,3,3,3,3,3,3,3,3,3,3,3,3,4),(0.,0.0967186461262831,
0.12500000000004,0.18750000000006,0.21875000000007,0.234375000000064,0.243656743286663,
0.250000000000058,0.304783310397428,0.358759691292195,0.375000000000016,
0.42752541592923,0.437500000000005,0.468750000000006,0.483401950931687,
0.498680111726324,0.500000000000007,0.585314944032889,0.673616873479213,
0.766999996706054,0.86351900109437,0.96497775590487,1.),.UNSPECIFIED.);
#1772=B_SPLINE_CURVE_WITH_KNOTS('',3,(#79069,#79070,#79071,#79072,#79073,
#79074,#79075,#79076,#79077,#79078,#79079,#79080,#79081,#79082,#79083,#79084,
#79085,#79086,#79087,#79088,#79089,#79090,#79091,#79092,#79093,#79094,#79095,
#79096,#79097,#79098,#79099,#79100,#79101,#79102,#79103,#79104,#79105,#79106,
#79107,#79108,#79109,#79110,#79111,#79112,#79113,#79114,#79115,#79116,#79117,
#79118,#79119,#79120,#79121,#79122,#79123,#79124,#79125,#79126,#79127,#79128,
#79129,#79130,#79131,#79132,#79133,#79134,#79135),.UNSPECIFIED.,.F.,.F.,
(4,3,3,3,3,3,3,3,3,3,3,3,3,3,3,3,3,3,3,3,3,3,4),(0.,0.100757444409959,0.196147984514473,
0.249999999999972,0.340191959854596,0.374999999999954,0.437499999999945,
0.468749999999941,0.484374999999938,0.498793165549547,0.499999999999936,
0.550373236664276,0.602950842746076,0.624999999999946,0.678928159561804,
0.687499999999961,0.718749999999969,0.734374999999973,0.742187499999975,
0.749999999999977,0.841743474586641,0.938196398372317,1.),.UNSPECIFIED.);
#1773=B_SPLINE_CURVE_WITH_KNOTS('',3,(#79143,#79144,#79145,#79146,#79147,
#79148,#79149,#79150,#79151,#79152,#79153,#79154,#79155,#79156,#79157,#79158,
#79159,#79160,#79161,#79162,#79163,#79164),.UNSPECIFIED.,.F.,.F.,(4,3,3,
3,3,3,3,4),(1.91917304179,2.05149792398005,2.18491877151797,2.22039294838,
2.3639360580223,2.50932327973008,2.52698484563,2.64214133457),
 .UNSPECIFIED.);
#1774=B_SPLINE_CURVE_WITH_KNOTS('',3,(#79166,#79167,#79168,#79169,#79170,
#79171,#79172,#79173,#79174,#79175,#79176,#79177,#79178,#79179,#79180,#79181,
#79182,#79183,#79184),.UNSPECIFIED.,.F.,.F.,(4,3,3,3,3,3,4),(1.95117092983,
2.10540845651,2.25964598319,2.39637208287195,2.53179243110294,2.56487158268,
2.67415250918),.UNSPECIFIED.);
#1775=B_SPLINE_CURVE_WITH_KNOTS('',3,(#79230,#79231,#79232,#79233,#79234,
#79235,#79236,#79237,#79238,#79239,#79240,#79241,#79242,#79243,#79244,#79245,
#79246,#79247,#79248,#79249,#79250,#79251),.UNSPECIFIED.,.F.,.F.,(4,3,3,
3,3,3,3,4),(1.91917304179,2.02579232441727,2.13535045929516,2.24802429461472,
2.36515236413743,2.48418559772032,2.60408580572557,2.64214133457),
 .UNSPECIFIED.);
#1776=B_SPLINE_CURVE_WITH_KNOTS('',3,(#79255,#79256,#79257,#79258,#79259,
#79260,#79261,#79262,#79263,#79264,#79265,#79266,#79267,#79268,#79269,#79270,
#79271,#79272,#79273,#79274,#79275,#79276,#79277,#79278,#79279,#79280,#79281,
#79282,#79283,#79284,#79285,#79286,#79287,#79288,#79289,#79290,#79291,#79292,
#79293,#79294,#79295,#79296,#79297,#79298,#79299,#79300,#79301,#79302,#79303,
#79304,#79305,#79306,#79307,#79308,#79309,#79310,#79311,#79312,#79313,#79314,
#79315,#79316,#79317,#79318,#79319,#79320,#79321,#79322,#79323,#79324,#79325,
#79326,#79327,#79328,#79329,#79330,#79331,#79332,#79333,#79334,#79335,#79336,
#79337,#79338,#79339,#79340,#79341,#79342,#79343,#79344,#79345,#79346,#79347,
#79348,#79349,#79350,#79351),.UNSPECIFIED.,.F.,.F.,(4,3,3,3,3,3,3,3,3,3,
3,3,3,3,3,3,3,3,3,3,3,3,3,3,3,3,3,3,3,3,3,3,4),(4.0025111321083E-13,0.0632489107248744,
0.125000000000003,0.187500000000005,0.218750000000006,0.235672573927374,
0.250000000000007,0.3073632326897,0.363175963289869,0.37500000000001,0.429360664035595,
0.437500000000012,0.468750000000012,0.484375000000012,0.492187500000013,
0.497903776612221,0.500000000000013,0.554907532207408,0.608404879582191,
0.625000000000013,0.676344675408734,0.687500000000013,0.718750000000014,
0.734375000000014,0.742187500000014,0.746093750000014,0.749653402950428,
0.750000000000014,0.808127914628195,0.864545740498736,0.920016589838173,
0.974147928007887,0.99999998552153),.UNSPECIFIED.);
#1777=B_SPLINE_CURVE_WITH_KNOTS('',3,(#79354,#79355,#79356,#79357,#79358,
#79359,#79360,#79361,#79362,#79363,#79364,#79365,#79366,#79367,#79368,#79369,
#79370,#79371,#79372,#79373,#79374,#79375),.UNSPECIFIED.,.F.,.F.,(4,3,3,
3,3,3,3,4),(1.95117092983,2.07121338925534,2.1903352130963,2.31128953711722,
2.42369300779211,2.53345239947667,2.6396571157376,2.67415250918),
 .UNSPECIFIED.);
#1778=B_SPLINE_CURVE_WITH_KNOTS('',5,(#79383,#79384,#79385,#79386,#79387,
#79388,#79389,#79390,#79391),.UNSPECIFIED.,.F.,.F.,(6,3,6),(0.,0.444536926591004,
1.),.UNSPECIFIED.);
#1779=B_SPLINE_CURVE_WITH_KNOTS('',5,(#79394,#79395,#79396,#79397,#79398,
#79399,#79400,#79401,#79402,#79403,#79404,#79405),.UNSPECIFIED.,.F.,.F.,
(6,3,3,6),(-1.80699050239119,-1.67012369382,-1.56537299057,-1.54695248492),
 .UNSPECIFIED.);
#1780=B_SPLINE_CURVE_WITH_KNOTS('',3,(#79407,#79408,#79409,#79410,#79411,
#79412,#79413,#79414,#79415,#79416,#79417,#79418,#79419,#79420,#79421,#79422,
#79423,#79424,#79425,#79426,#79427,#79428),.UNSPECIFIED.,.F.,.F.,(4,3,3,
3,3,3,3,4),(-4.36798756241,-4.169936044415,-3.99462490463767,-3.97188452642,
-3.81611914244834,-3.6712886258062,-3.62984805881,-3.53583307557),
 .UNSPECIFIED.);
#1781=B_SPLINE_CURVE_WITH_KNOTS('',3,(#79433,#79434,#79435,#79436,#79437,
#79438,#79439,#79440,#79441,#79442,#79443,#79444,#79445,#79446,#79447,#79448,
#79449,#79450,#79451,#79452,#79453,#79454,#79455,#79456,#79457,#79458,#79459,
#79460,#79461,#79462,#79463,#79464,#79465,#79466,#79467,#79468,#79469,#79470,
#79471,#79472,#79473,#79474,#79475),.UNSPECIFIED.,.F.,.F.,(4,3,3,3,3,3,
3,3,3,3,3,3,3,3,4),(-2.1197288877,-1.98841331521492,-1.86159678165,-1.7188993737364,
-1.60356346906,-1.44037681505088,-1.3668875221,-1.17788035732586,-1.13023412606,
-0.922050724180072,-0.709993980015713,-0.657118805891,-0.442216022332552,
-0.328557428358,-0.109166698395),.UNSPECIFIED.);
#1782=B_SPLINE_CURVE_WITH_KNOTS('',3,(#79477,#79478,#79479,#79480,#79481,
#79482,#79483,#79484,#79485,#79486,#79487,#79488,#79489,#79490,#79491,#79492,
#79493,#79494,#79495,#79496,#79497,#79498,#79499,#79500,#79501),
 .UNSPECIFIED.,.F.,.F.,(4,3,3,3,3,3,3,3,4),(-1.73791866609,-1.69805976489305,
-1.65573758388662,-1.61550378495,-1.56701234941871,-1.51549851525847,-1.49803365755,
-1.45023151716658,-1.40796354572),.UNSPECIFIED.);
#1783=B_SPLINE_CURVE_WITH_KNOTS('',3,(#79504,#79505,#79506,#79507,#79508,
#79509,#79510,#79511,#79512,#79513,#79514,#79515,#79516,#79517,#79518,#79519,
#79520,#79521,#79522,#79523,#79524,#79525,#79526,#79527,#79528,#79529,#79530,
#79531,#79532,#79533,#79534,#79535,#79536,#79537,#79538,#79539,#79540,#79541,
#79542,#79543,#79544,#79545,#79546),.UNSPECIFIED.,.F.,.F.,(4,3,3,3,3,3,
3,3,3,3,3,3,3,3,4),(-3.16496476901,-3.05739501013341,-2.95490927595688,
-2.89022619818,-2.80130651793357,-2.71899621993714,-2.64235434316,-2.57577600227824,
-2.53314284706,-2.46341560037499,-2.42388273879,-2.35998782232,-2.29609290585,
-2.23666406729655,-2.21471914028),.UNSPECIFIED.);
#1784=B_SPLINE_CURVE_WITH_KNOTS('',3,(#79548,#79549,#79550,#79551,#79552,
#79553,#79554,#79555,#79556,#79557,#79558,#79559,#79560,#79561,#79562,#79563,
#79564,#79565,#79566,#79567,#79568,#79569,#79570,#79571,#79572,#79573,#79574,
#79575,#79576,#79577,#79578,#79579,#79580,#79581,#79582,#79583,#79584,#79585,
#79586,#79587),.UNSPECIFIED.,.F.,.F.,(4,3,3,3,3,3,3,3,3,3,3,3,3,4),(-3.15494946668974,
-3.09429422325597,-3.03469546375,-2.97101336920453,-2.90283799032044,-2.84788436267,
-2.77508951699777,-2.70623933891542,-2.64437519712,-2.56234040630418,-2.47134155465,
-2.36779504868473,-2.29839214685,-2.20468603571421),.UNSPECIFIED.);
#1785=B_SPLINE_CURVE_WITH_KNOTS('',3,(#79590,#79591,#79592,#79593,#79594,
#79595,#79596,#79597,#79598,#79599,#79600,#79601,#79602,#79603,#79604,#79605,
#79606,#79607,#79608,#79609,#79610,#79611,#79612,#79613,#79614,#79615,#79616,
#79617),.UNSPECIFIED.,.F.,.F.,(4,3,3,3,3,3,3,3,3,4),(-1.77221556182,-1.72541256452829,
-1.67470799810622,-1.63241886503,-1.58516494184952,-1.55011502341,-1.50856575067229,
-1.49939588111,-1.45848471590269,-1.44228974252),.UNSPECIFIED.);
#1786=B_SPLINE_CURVE_WITH_KNOTS('',3,(#79619,#79620,#79621,#79622,#79623,
#79624,#79625,#79626,#79627,#79628,#79629,#79630,#79631,#79632,#79633,#79634,
#79635,#79636,#79637,#79638,#79639,#79640,#79641,#79642,#79643,#79644,#79645,
#79646,#79647,#79648,#79649,#79650,#79651,#79652,#79653,#79654,#79655,#79656,
#79657,#79658),.UNSPECIFIED.,.F.,.F.,(4,3,3,3,3,3,3,3,3,3,3,3,3,4),(-5.02326603963,
-4.80637580757057,-4.59184582783107,-4.46470265851,-4.25520068526698,-4.05094564988226,
-3.90600477275,-3.72858936815271,-3.56430826698,-3.41556843081671,-3.27772290795148,
-3.22245900472,-3.09341777853601,-3.01269951131),.UNSPECIFIED.);
#1787=B_SPLINE_CURVE_WITH_KNOTS('',3,(#79663,#79664,#79665,#79666,#79667,
#79668,#79669,#79670,#79671,#79672,#79673,#79674,#79675,#79676,#79677,#79678,
#79679,#79680,#79681,#79682,#79683,#79684),.UNSPECIFIED.,.F.,.F.,(4,3,3,
3,3,3,3,4),(-7.33762762903,-7.19451398421356,-7.08790984155,-6.92735535556756,
-6.82008855637394,-6.62897001935503,-6.58881135386,-6.50557700429),
 .UNSPECIFIED.);
#1788=B_SPLINE_CURVE_WITH_KNOTS('',5,(#79686,#79687,#79688,#79689,#79690,
#79691,#79692,#79693,#79694,#79695,#79696,#79697),.UNSPECIFIED.,.F.,.F.,
(6,3,3,6),(-1.75479504935,-1.62859651807,-1.50635582191,-1.4947188012),
 .UNSPECIFIED.);
#1789=B_SPLINE_CURVE_WITH_KNOTS('',5,(#79700,#79701,#79702,#79703,#79704,
#79705,#79706,#79707,#79708),.UNSPECIFIED.,.F.,.F.,(6,3,6),(3.35057951372198E-8,
0.468594524318655,1.),.UNSPECIFIED.);
#1790=B_SPLINE_CURVE_WITH_KNOTS('',5,(#79823,#79824,#79825,#79826,#79827,
#79828,#79829,#79830,#79831),.UNSPECIFIED.,.F.,.F.,(6,3,6),(-6.00042817873,
-5.42884095166,-5.20521075808),.UNSPECIFIED.);
#1791=B_SPLINE_CURVE_WITH_KNOTS('',3,(#79833,#79834,#79835,#79836,#79837,
#79838,#79839,#79840,#79841,#79842,#79843,#79844,#79845,#79846,#79847,#79848,
#79849,#79850,#79851,#79852,#79853,#79854,#79855,#79856,#79857),
 .UNSPECIFIED.,.F.,.F.,(4,3,3,3,3,3,3,3,4),(0.,0.125,0.249051326604059,
0.37312891753387,0.497226955279358,0.622920216459519,0.747043580627599,
0.873521790313799,1.),.UNSPECIFIED.);
#1792=B_SPLINE_CURVE_WITH_KNOTS('',5,(#79859,#79860,#79861,#79862,#79863,
#79864,#79865,#79866,#79867),.UNSPECIFIED.,.F.,.F.,(6,3,6),(1.9878298196,
2.20723764364,2.53578324996),.UNSPECIFIED.);
#1793=B_SPLINE_CURVE_WITH_KNOTS('',5,(#79869,#79870,#79871,#79872,#79873,
#79874),.UNSPECIFIED.,.F.,.F.,(6,6),(5.20484021909,5.76063633602),
 .UNSPECIFIED.);
#1794=B_SPLINE_CURVE_WITH_KNOTS('',3,(#79886,#79887,#79888,#79889,#79890,
#79891,#79892,#79893,#79894,#79895,#79896,#79897,#79898,#79899,#79900,#79901,
#79902,#79903,#79904,#79905,#79906,#79907,#79908,#79909,#79910,#79911,#79912,
#79913,#79914,#79915,#79916,#79917,#79918,#79919,#79920,#79921,#79922),
 .UNSPECIFIED.,.F.,.F.,(4,3,3,3,3,3,3,3,3,3,3,3,4),(1.62679171178,1.80119189921,
2.06549727040562,2.33022193180684,2.59511005010776,2.8601162004504,2.9864917,
3.25107716364615,3.51563595035349,3.56612301471,3.83086251970706,4.09597227277403,
4.14575432942),.UNSPECIFIED.);
#1795=B_SPLINE_CURVE_WITH_KNOTS('',3,(#80019,#80020,#80021,#80022,#80023,
#80024,#80025,#80026,#80027,#80028),.UNSPECIFIED.,.F.,.F.,(4,3,3,4),(-6.00042817873,
-5.73764962787167,-5.47143019297584,-5.20521075808),.UNSPECIFIED.);
#1796=B_SPLINE_CURVE_WITH_KNOTS('',3,(#80031,#80032,#80033,#80034,#80035,
#80036,#80037,#80038,#80039,#80040,#80041,#80042,#80043,#80044,#80045,#80046,
#80047,#80048,#80049,#80050,#80051,#80052,#80053,#80054,#80055,#80056,#80057,
#80058,#80059,#80060,#80061,#80062,#80063,#80064,#80065,#80066,#80067,#80068,
#80069,#80070,#80071,#80072,#80073,#80074,#80075,#80076,#80077,#80078,#80079,
#80080,#80081,#80082,#80083,#80084,#80085),.UNSPECIFIED.,.F.,.F.,(4,3,3,
3,3,3,3,3,3,3,3,3,3,3,3,3,3,3,4),(-4.71575303852,-4.65907697863314,-4.59837909975905,
-4.56620180037,-4.49782940088838,-4.45572366868,-4.37891278786157,-4.34130806771,
-4.27463577302459,-4.21375904184622,-4.18701109461,-4.10530819905221,-4.019523415627,
-3.96784558239,-3.87773712401142,-3.78337627560873,-3.75420974096,-3.65160927305,
-3.54900880514),.UNSPECIFIED.);
#1797=B_SPLINE_CURVE_WITH_KNOTS('',5,(#80132,#80133,#80134,#80135,#80136,
#80137),.UNSPECIFIED.,.F.,.F.,(6,6),(5.20484021909,5.76063633602),
 .UNSPECIFIED.);
#1798=B_SPLINE_CURVE_WITH_KNOTS('',3,(#80175,#80176,#80177,#80178,#80179,
#80180,#80181,#80182,#80183,#80184,#80185,#80186,#80187),.UNSPECIFIED.,
 .F.,.F.,(4,3,3,3,4),(0.,0.253975090744685,0.502216732464109,0.751108366232054,
1.),.UNSPECIFIED.);
#1799=B_SPLINE_CURVE_WITH_KNOTS('',5,(#80199,#80200,#80201,#80202,#80203,
#80204,#80205,#80206,#80207),.UNSPECIFIED.,.F.,.F.,(6,3,6),(0.,0.546822749333166,
1.),.UNSPECIFIED.);
#1800=B_SPLINE_CURVE_WITH_KNOTS('',5,(#80225,#80226,#80227,#80228,#80229,
#80230,#80231,#80232,#80233),.UNSPECIFIED.,.F.,.F.,(6,3,6),(0.,0.45317725066295,
1.),.UNSPECIFIED.);
#1801=B_SPLINE_CURVE_WITH_KNOTS('',3,(#80348,#80349,#80350,#80351,#80352,
#80353,#80354,#80355,#80356,#80357,#80358,#80359,#80360,#80361,#80362,#80363,
#80364,#80365,#80366,#80367,#80368,#80369,#80370,#80371,#80372,#80373,#80374,
#80375,#80376,#80377,#80378,#80379,#80380,#80381,#80382,#80383,#80384,#80385,
#80386,#80387,#80388,#80389,#80390,#80391,#80392,#80393,#80394,#80395,#80396,
#80397,#80398,#80399,#80400,#80401,#80402),.UNSPECIFIED.,.F.,.F.,(4,3,3,
3,3,3,3,3,3,3,3,3,3,3,3,3,3,3,4),(3.54900880515,3.651609273055,3.75420974096,
3.84893307386556,3.93929532064981,3.96784558239,4.05430391724671,4.13645477350633,
4.18701109461,4.24753706288369,4.31344142163189,4.34130806771,4.41811894852724,
4.45572366868,4.52409606816139,4.56620180037,4.62755792701915,4.68459440694729,
4.71575303852),.UNSPECIFIED.);
#1802=B_SPLINE_CURVE_WITH_KNOTS('',5,(#80754,#80755,#80756,#80757,#80758,
#80759),.UNSPECIFIED.,.F.,.F.,(6,6),(3.1859449136978E-8,1.),
 .UNSPECIFIED.);
#1803=B_SPLINE_CURVE_WITH_KNOTS('',3,(#80765,#80766,#80767,#80768,#80769,
#80770,#80771,#80772,#80773,#80774),.UNSPECIFIED.,.F.,.F.,(4,2,2,2,4),(0.,
0.25,0.5,0.75,1.),.UNSPECIFIED.);
#1804=B_SPLINE_CURVE_WITH_KNOTS('',3,(#80792,#80793,#80794,#80795,#80796,
#80797,#80798,#80799,#80800,#80801,#80802,#80803,#80804,#80805,#80806,#80807,
#80808,#80809,#80810,#80811,#80812,#80813,#80814,#80815,#80816,#80817,#80818,
#80819,#80820,#80821,#80822),.UNSPECIFIED.,.F.,.F.,(4,3,3,3,3,3,3,3,3,3,
4),(0.,0.103486941292664,0.209722140116913,0.317273808041208,0.426249484256839,
0.5,0.609150430624086,0.71686238797799,0.823269317845894,0.927288353897733,
1.),.UNSPECIFIED.);
#1805=B_SPLINE_CURVE_WITH_KNOTS('',3,(#80864,#80865,#80866,#80867,#80868,
#80869,#80870,#80871,#80872,#80873,#80874,#80875,#80876),.UNSPECIFIED.,
 .F.,.F.,(4,3,3,3,4),(0.,0.283655470482566,0.567100173465966,0.871696373072702,
1.),.UNSPECIFIED.);
#1806=B_SPLINE_CURVE_WITH_KNOTS('',3,(#80988,#80989,#80990,#80991,#80992,
#80993,#80994,#80995,#80996,#80997,#80998,#80999,#81000,#81001,#81002,#81003,
#81004,#81005,#81006,#81007,#81008,#81009,#81010,#81011,#81012,#81013,#81014,
#81015,#81016,#81017,#81018,#81019,#81020,#81021,#81022,#81023,#81024,#81025,
#81026,#81027,#81028,#81029,#81030,#81031,#81032,#81033,#81034,#81035,#81036,
#81037,#81038,#81039,#81040,#81041,#81042,#81043,#81044,#81045,#81046,#81047,
#81048,#81049,#81050,#81051,#81052,#81053,#81054,#81055,#81056,#81057,#81058,
#81059,#81060,#81061,#81062,#81063,#81064,#81065,#81066),.UNSPECIFIED.,
 .F.,.F.,(4,3,3,3,3,3,3,3,3,3,3,3,3,3,3,3,3,3,3,3,3,3,3,3,3,3,4),(0.,0.0787260457931564,
0.124999999999993,0.187499999999992,0.218749999999992,0.247757967308853,
0.249999999999991,0.331434298157057,0.37499999999999,0.449421300548547,
0.466731041768843,0.483365520884418,0.485303339327099,0.495778997034871,
0.499999999999993,0.548146868097096,0.624999999999991,0.687499999999989,
0.718749999999989,0.734374999999988,0.742936082500893,0.749999999999988,
0.816779350141409,0.883437797437894,0.937634632232333,0.984782267543852,
1.),.UNSPECIFIED.);
#1807=B_SPLINE_CURVE_WITH_KNOTS('',3,(#81150,#81151,#81152,#81153,#81154,
#81155,#81156,#81157,#81158,#81159,#81160,#81161,#81162,#81163,#81164,#81165,
#81166,#81167,#81168,#81169,#81170,#81171,#81172,#81173,#81174,#81175,#81176,
#81177,#81178,#81179,#81180,#81181,#81182,#81183,#81184,#81185,#81186,#81187,
#81188,#81189,#81190,#81191,#81192,#81193,#81194,#81195,#81196,#81197,#81198,
#81199,#81200,#81201,#81202,#81203,#81204,#81205,#81206,#81207,#81208,#81209,
#81210,#81211,#81212,#81213,#81214,#81215,#81216,#81217,#81218,#81219,#81220,
#81221,#81222,#81223,#81224,#81225,#81226,#81227,#81228,#81229,#81230,#81231,
#81232,#81233,#81234,#81235,#81236,#81237),.UNSPECIFIED.,.F.,.F.,(4,3,3,
3,3,3,3,3,3,3,3,3,3,3,3,3,3,3,3,3,3,3,3,3,3,3,3,3,3,4),(0.,0.0468087724836094,
0.100006845757394,0.135651264268524,0.192825632134262,0.221412816067131,
0.228559612050348,0.233919709037761,0.235289363314821,0.243650512143623,
0.25,0.31592266226525,0.374999999999993,0.425566231049382,0.43749999999999,
0.451681239474872,0.468749999999989,0.484374999999988,0.493507364861486,
0.499999999999987,0.578683814801776,0.624999999999991,0.687499999999992,
0.718749999999993,0.734374999999993,0.745475655325922,0.749999999999993,
0.861453741249095,0.944849601132576,1.),.UNSPECIFIED.);
#1808=B_SPLINE_CURVE_WITH_KNOTS('',3,(#81297,#81298,#81299,#81300,#81301,
#81302,#81303,#81304,#81305,#81306,#81307,#81308,#81309,#81310,#81311,#81312,
#81313,#81314,#81315,#81316,#81317,#81318,#81319,#81320,#81321,#81322,#81323,
#81324,#81325,#81326,#81327,#81328,#81329,#81330,#81331,#81332,#81333,#81334,
#81335,#81336,#81337,#81338,#81339,#81340,#81341,#81342,#81343,#81344,#81345,
#81346,#81347,#81348,#81349,#81350,#81351,#81352,#81353,#81354,#81355,#81356,
#81357,#81358,#81359,#81360,#81361,#81362,#81363,#81364,#81365,#81366,#81367,
#81368,#81369,#81370,#81371,#81372,#81373,#81374,#81375,#81376,#81377,#81378),
 .UNSPECIFIED.,.F.,.F.,(4,3,3,3,3,3,3,3,3,3,3,3,3,3,3,3,3,3,3,3,3,3,3,3,
3,3,3,4),(0.,0.101529500922143,0.222413752673,0.249999999999876,0.362127564372828,
0.374999999999812,0.437499999999778,0.46874999999976,0.484374999999751,
0.48892738670375,0.492135627913471,0.492858316487225,0.493479773407748,
0.499999999999745,0.601963594423371,0.624999999999756,0.687499999999762,
0.718749999999763,0.734374999999762,0.74218749999976,0.746093749999758,
0.749999999999756,0.795770799058943,0.841887284320127,0.887967824962089,
0.933349893659305,0.976313037422695,1.),.UNSPECIFIED.);
#1809=B_SPLINE_CURVE_WITH_KNOTS('',3,(#81466,#81467,#81468,#81469,#81470,
#81471,#81472,#81473,#81474,#81475,#81476,#81477,#81478,#81479,#81480,#81481,
#81482,#81483,#81484,#81485,#81486,#81487,#81488,#81489,#81490,#81491,#81492,
#81493,#81494,#81495,#81496,#81497,#81498,#81499,#81500,#81501,#81502,#81503,
#81504,#81505,#81506,#81507,#81508,#81509,#81510,#81511,#81512,#81513,#81514,
#81515,#81516,#81517,#81518,#81519,#81520),.UNSPECIFIED.,.F.,.F.,(4,3,3,
3,3,3,3,3,3,3,3,3,3,3,3,3,3,3,4),(0.,0.120637102514753,0.250000000000005,
0.375000000000008,0.437500000000011,0.46400815730569,0.468497525776301,
0.470967635615609,0.487729750531094,0.494705110367547,0.497908251856533,
0.499991186139283,0.501597039562557,0.543532629222724,0.626157938461672,
0.747341134508375,0.859198878060181,0.960140090645202,1.),.UNSPECIFIED.);
#1810=B_SPLINE_CURVE_WITH_KNOTS('',3,(#81604,#81605,#81606,#81607,#81608,
#81609,#81610,#81611,#81612,#81613,#81614,#81615,#81616,#81617,#81618,#81619,
#81620,#81621,#81622,#81623,#81624,#81625,#81626,#81627,#81628,#81629,#81630,
#81631,#81632,#81633,#81634,#81635,#81636,#81637,#81638,#81639,#81640,#81641,
#81642,#81643,#81644,#81645,#81646),.UNSPECIFIED.,.F.,.F.,(4,3,3,3,3,3,
3,3,3,3,3,3,3,3,4),(0.,0.0966694249688917,0.231867346864773,0.250000000000024,
0.352344865255222,0.375000000000035,0.437500000000042,0.468750000000045,
0.483362225881677,0.500000000000047,0.545177325600272,0.705546343994153,
0.856284891331945,0.975254970201329,1.),.UNSPECIFIED.);
#1811=B_SPLINE_CURVE_WITH_KNOTS('',3,(#81797,#81798,#81799,#81800,#81801,
#81802,#81803,#81804,#81805,#81806,#81807,#81808,#81809),.UNSPECIFIED.,
 .F.,.F.,(4,3,3,3,4),(0.,0.290643058527184,0.585647964061105,0.887654578917741,
1.),.UNSPECIFIED.);
#1812=B_SPLINE_CURVE_WITH_KNOTS('',3,(#81878,#81879,#81880,#81881,#81882,
#81883,#81884,#81885,#81886,#81887),.UNSPECIFIED.,.F.,.F.,(4,3,3,4),(0.,
0.388137409541929,0.768803426065497,1.),.UNSPECIFIED.);
#1813=B_SPLINE_CURVE_WITH_KNOTS('',3,(#81952,#81953,#81954,#81955,#81956,
#81957,#81958,#81959,#81960,#81961,#81962,#81963,#81964),.UNSPECIFIED.,
 .F.,.F.,(4,3,3,3,4),(0.,0.301170390997793,0.597353856341166,0.886897365258997,
1.),.UNSPECIFIED.);
#1814=B_SPLINE_CURVE_WITH_KNOTS('',3,(#82002,#82003,#82004,#82005,#82006,
#82007,#82008,#82009,#82010,#82011),.UNSPECIFIED.,.F.,.F.,(4,3,3,4),(0.,
0.379616953105207,0.766838018123526,0.999999998064869),.UNSPECIFIED.);
#1815=B_SPLINE_CURVE_WITH_KNOTS('',3,(#82165,#82166,#82167,#82168,#82169,
#82170,#82171,#82172,#82173,#82174,#82175,#82176,#82177,#82178,#82179,#82180,
#82181,#82182,#82183,#82184,#82185,#82186,#82187,#82188,#82189,#82190,#82191,
#82192,#82193,#82194,#82195),.UNSPECIFIED.,.F.,.F.,(4,3,3,3,3,3,3,3,3,3,
4),(0.,0.0997880523616104,0.200062662981434,0.301948937113961,0.405212424694865,
0.51037062471613,0.61810126360354,0.731592938427962,0.849728512114637,0.976002843446623,
1.),.UNSPECIFIED.);
#1816=B_SPLINE_CURVE_WITH_KNOTS('',3,(#82363,#82364,#82365,#82366,#82367,
#82368,#82369,#82370,#82371,#82372,#82373,#82374,#82375,#82376,#82377,#82378,
#82379,#82380,#82381,#82382,#82383,#82384,#82385,#82386,#82387,#82388,#82389,
#82390,#82391,#82392,#82393,#82394,#82395,#82396,#82397,#82398,#82399,#82400,
#82401,#82402,#82403,#82404,#82405,#82406,#82407,#82408,#82409,#82410,#82411,
#82412,#82413,#82414,#82415,#82416,#82417,#82418,#82419,#82420,#82421,#82422,
#82423,#82424,#82425,#82426,#82427,#82428,#82429,#82430,#82431,#82432,#82433,
#82434,#82435),.UNSPECIFIED.,.F.,.F.,(4,3,3,3,3,3,3,3,3,3,3,3,3,3,3,3,3,
3,3,3,3,3,3,3,4),(0.,0.0437264140634012,0.089989771863013,0.12499999999996,
0.170646942111976,0.187499999999941,0.218749999999933,0.234374999999931,
0.242187499999928,0.246093749999931,0.249999999999934,0.324140195987469,
0.374999999999962,0.437499999999977,0.468749999999983,0.484374999999987,
0.492187499999989,0.499419384271932,0.499999999999991,0.546155699914753,
0.638263904679061,0.757052346717483,0.864898370340035,0.957922231030437,
1.),.UNSPECIFIED.);
#1817=B_SPLINE_CURVE_WITH_KNOTS('',3,(#82525,#82526,#82527,#82528,#82529,
#82530,#82531,#82532,#82533,#82534,#82535,#82536,#82537),.UNSPECIFIED.,
 .F.,.F.,(4,3,3,3,4),(0.,0.32216108780556,0.609771124076306,0.905431279270806,
1.),.UNSPECIFIED.);
#1818=B_SPLINE_CURVE_WITH_KNOTS('',3,(#82548,#82549,#82550,#82551,#82552,
#82553,#82554,#82555,#82556,#82557,#82558,#82559,#82560,#82561,#82562,#82563,
#82564,#82565,#82566,#82567,#82568,#82569,#82570,#82571,#82572,#82573,#82574,
#82575,#82576,#82577,#82578,#82579,#82580,#82581,#82582,#82583,#82584,#82585,
#82586,#82587,#82588,#82589,#82590,#82591,#82592,#82593,#82594,#82595,#82596,
#82597,#82598,#82599,#82600,#82601,#82602),.UNSPECIFIED.,.F.,.F.,(4,3,3,
3,3,3,3,3,3,3,3,3,3,3,3,3,3,3,4),(-4.71575303852,-4.65907697863314,-4.59837909975905,
-4.56620180037,-4.49782940088838,-4.45572366868,-4.37891278786157,-4.34130806771,
-4.27463577302459,-4.21375904184622,-4.18701109461,-4.10530819905221,-4.019523415627,
-3.96784558239,-3.87773712401142,-3.78337627560873,-3.75420974096,-3.65160927305,
-3.54900880514),.UNSPECIFIED.);
#1819=B_SPLINE_CURVE_WITH_KNOTS('',3,(#82604,#82605,#82606,#82607,#82608,
#82609,#82610,#82611,#82612,#82613),.UNSPECIFIED.,.F.,.F.,(4,3,3,4),(-6.00042817873,
-5.73764962787167,-5.47143019297584,-5.20521075808),.UNSPECIFIED.);
#1820=B_SPLINE_CURVE_WITH_KNOTS('',3,(#82649,#82650,#82651,#82652,#82653,
#82654,#82655,#82656,#82657,#82658,#82659,#82660,#82661,#82662,#82663,#82664),
 .UNSPECIFIED.,.F.,.F.,(4,3,3,3,3,4),(1.9878298196,2.12810444562736,2.20723764364,
2.34744480889074,2.48762106236855,2.53578324996),.UNSPECIFIED.);
#1821=B_SPLINE_CURVE_WITH_KNOTS('',3,(#82670,#82671,#82672,#82673,#82674,
#82675,#82676,#82677,#82678,#82679,#82680,#82681,#82682,#82683,#82684,#82685,
#82686,#82687,#82688,#82689,#82690,#82691,#82692,#82693,#82694,#82695,#82696,
#82697,#82698,#82699,#82700,#82701,#82702,#82703,#82704,#82705,#82706),
 .UNSPECIFIED.,.F.,.F.,(4,3,3,3,3,3,3,3,3,3,3,3,4),(1.62679171178,1.80119189921,
2.06549727040562,2.33022193180684,2.59511005010776,2.8601162004504,2.9864917,
3.25107716364615,3.51563595035349,3.56612301471,3.83086251970706,4.09597227277403,
4.14575432942),.UNSPECIFIED.);
#1822=B_SPLINE_CURVE_WITH_KNOTS('',3,(#82771,#82772,#82773,#82774,#82775,
#82776,#82777,#82778,#82779,#82780),.UNSPECIFIED.,.F.,.F.,(4,3,3,4),(0.,
0.393559372360371,0.800977653566811,1.),.UNSPECIFIED.);
#1823=B_SPLINE_CURVE_WITH_KNOTS('',3,(#82835,#82836,#82837,#82838,#82839,
#82840,#82841,#82842,#82843,#82844,#82845,#82846,#82847,#82848,#82849,#82850,
#82851,#82852,#82853,#82854,#82855,#82856,#82857,#82858,#82859,#82860,#82861,
#82862,#82863,#82864,#82865,#82866,#82867,#82868,#82869,#82870,#82871,#82872,
#82873,#82874,#82875,#82876,#82877,#82878,#82879,#82880,#82881,#82882,#82883,
#82884,#82885,#82886,#82887,#82888,#82889,#82890,#82891,#82892,#82893,#82894,
#82895,#82896,#82897,#82898,#82899,#82900,#82901),.UNSPECIFIED.,.F.,.F.,
(4,3,3,3,3,3,3,3,3,3,3,3,3,3,3,3,3,3,3,3,3,3,4),(0.,0.0466542567303633,
0.100279857526539,0.162566268563517,0.222223321736243,0.250000000000032,
0.32224695109353,0.371748221688835,0.420281745240556,0.462936832422792,
0.481468416211426,0.484289083525892,0.485665060839194,0.493820456455645,
0.500000000000061,0.582690514763901,0.661722188633312,0.737674786625859,
0.75000000000003,0.825845181320885,0.900982137734557,0.97270193986251,1.),
 .UNSPECIFIED.);
#1824=B_SPLINE_CURVE_WITH_KNOTS('',5,(#82930,#82931,#82932,#82933,#82934,
#82935),.UNSPECIFIED.,.F.,.F.,(6,6),(5.20484021909,5.76063633602),
 .UNSPECIFIED.);
#1825=B_SPLINE_CURVE_WITH_KNOTS('',3,(#82936,#82937,#82938,#82939,#82940,
#82941,#82942,#82943,#82944,#82945,#82946,#82947,#82948,#82949,#82950,#82951,
#82952,#82953,#82954,#82955,#82956,#82957,#82958,#82959,#82960,#82961,#82962,
#82963,#82964,#82965,#82966,#82967,#82968,#82969,#82970,#82971,#82972,#82973,
#82974,#82975,#82976,#82977,#82978,#82979,#82980,#82981,#82982,#82983,#82984,
#82985,#82986,#82987,#82988,#82989,#82990),.UNSPECIFIED.,.F.,.F.,(4,3,3,
3,3,3,3,3,3,3,3,3,3,3,3,3,3,3,4),(3.54900880515,3.651609273055,3.75420974096,
3.84893307386556,3.93929532064981,3.96784558239,4.05430391724671,4.13645477350633,
4.18701109461,4.24753706288369,4.31344142163189,4.34130806771,4.41811894852724,
4.45572366868,4.52409606816139,4.56620180037,4.62755792701915,4.68459440694729,
4.71575303852),.UNSPECIFIED.);
#1826=B_SPLINE_CURVE_WITH_KNOTS('',3,(#83031,#83032,#83033,#83034,#83035,
#83036,#83037),.UNSPECIFIED.,.F.,.F.,(4,3,4),(5.20484021909,5.51152466079559,
5.76063633567283),.UNSPECIFIED.);
#1827=B_SPLINE_CURVE_WITH_KNOTS('',3,(#83092,#83093,#83094,#83095,#83096,
#83097,#83098,#83099,#83100,#83101,#83102,#83103,#83104,#83105,#83106,#83107,
#83108,#83109,#83110,#83111,#83112,#83113,#83114,#83115,#83116,#83117,#83118,
#83119,#83120,#83121,#83122,#83123,#83124,#83125,#83126,#83127,#83128,#83129,
#83130,#83131,#83132,#83133,#83134,#83135,#83136,#83137,#83138,#83139,#83140,
#83141,#83142,#83143,#83144,#83145,#83146,#83147,#83148,#83149,#83150,#83151,
#83152,#83153,#83154,#83155),.UNSPECIFIED.,.F.,.F.,(4,3,3,3,3,3,3,3,3,3,
3,3,3,3,3,3,3,3,3,3,3,4),(0.,0.0726878348096301,0.147617440689613,0.22357937320159,
0.250000000000044,0.325585219584544,0.375000000000065,0.437500000000074,
0.468750000000078,0.484375000000076,0.493410050348708,0.500000000000073,
0.537063812349334,0.579892736074948,0.63030009007674,0.696058572840903,
0.750000000000037,0.808743423167996,0.871226719986258,0.928440251933461,
0.975705935423915,1.),.UNSPECIFIED.);
#1828=B_SPLINE_CURVE_WITH_KNOTS('',5,(#83168,#83169,#83170,#83171,#83172,
#83173,#83174,#83175,#83176),.UNSPECIFIED.,.F.,.F.,(6,3,6),(1.9878298196,
2.20723764364,2.53578324996),.UNSPECIFIED.);
#1829=B_SPLINE_CURVE_WITH_KNOTS('',3,(#83178,#83179,#83180,#83181,#83182,
#83183,#83184,#83185,#83186,#83187,#83188,#83189,#83190,#83191,#83192,#83193,
#83194,#83195,#83196,#83197,#83198,#83199,#83200,#83201,#83202),
 .UNSPECIFIED.,.F.,.F.,(4,3,3,3,3,3,3,3,4),(0.,0.125,0.250543946517898,
0.377358570830386,0.5,0.626576440687726,0.752623525909811,0.876311762954906,
1.),.UNSPECIFIED.);
#2048=SHAPE_REPRESENTATION_RELATIONSHIP('SRR','None',#98345,#2058);
#2058=ADVANCED_BREP_SHAPE_REPRESENTATION('',(#2077),#98297);
#2068=STYLED_ITEM('',(#98399),#2077);
#2077=MANIFOLD_SOLID_BREP('Body1',#34174);
#2280=PLANE('',#35761);
#2281=PLANE('',#35764);
#2282=PLANE('',#35768);
#2283=PLANE('',#35794);
#2284=PLANE('',#35798);
#2285=PLANE('',#35823);
#2286=PLANE('',#35827);
#2287=PLANE('',#35830);
#2288=PLANE('',#35834);
#2289=PLANE('',#35870);
#2290=PLANE('',#35883);
#2291=PLANE('',#35905);
#2292=PLANE('',#35914);
#2293=PLANE('',#36051);
#2294=PLANE('',#36052);
#2295=PLANE('',#36059);
#2296=PLANE('',#36065);
#2297=PLANE('',#36067);
#2298=PLANE('',#36073);
#2299=PLANE('',#36076);
#2300=PLANE('',#36079);
#2301=PLANE('',#36082);
#2302=PLANE('',#36085);
#2303=PLANE('',#36088);
#2304=PLANE('',#36091);
#2305=PLANE('',#36094);
#2306=PLANE('',#36097);
#2307=PLANE('',#36100);
#2308=PLANE('',#36103);
#2309=PLANE('',#36116);
#2310=PLANE('',#36197);
#2311=PLANE('',#36205);
#2312=PLANE('',#36239);
#2313=PLANE('',#36271);
#2314=PLANE('',#36275);
#2315=PLANE('',#36299);
#2316=PLANE('',#36315);
#2317=PLANE('',#36317);
#2318=PLANE('',#36338);
#2319=PLANE('',#36340);
#2320=PLANE('',#36342);
#2321=PLANE('',#36359);
#2322=PLANE('',#36368);
#2776=CYLINDRICAL_SURFACE('',#35763,0.300000000000002);
#2777=CYLINDRICAL_SURFACE('',#35767,0.300000000000002);
#2778=CYLINDRICAL_SURFACE('',#35796,0.730765926094);
#2779=CYLINDRICAL_SURFACE('',#35803,0.3);
#2780=CYLINDRICAL_SURFACE('',#35809,0.3);
#2781=CYLINDRICAL_SURFACE('',#35813,0.3);
#2782=CYLINDRICAL_SURFACE('',#35817,0.3);
#2783=CYLINDRICAL_SURFACE('',#35825,1.);
#2784=CYLINDRICAL_SURFACE('',#35828,0.5);
#2785=CYLINDRICAL_SURFACE('',#35831,0.5);
#2786=CYLINDRICAL_SURFACE('',#35838,4.15);
#2787=CYLINDRICAL_SURFACE('',#35841,0.1);
#2788=CYLINDRICAL_SURFACE('',#35844,1.);
#2789=CYLINDRICAL_SURFACE('',#35849,0.0999999999999998);
#2790=CYLINDRICAL_SURFACE('',#35854,0.0999999999999998);
#2791=CYLINDRICAL_SURFACE('',#35860,0.3);
#2792=CYLINDRICAL_SURFACE('',#35862,0.3);
#2793=CYLINDRICAL_SURFACE('',#35865,1.);
#2794=CYLINDRICAL_SURFACE('',#35868,0.1);
#2795=CYLINDRICAL_SURFACE('',#35872,0.5);
#2796=CYLINDRICAL_SURFACE('',#35878,0.5);
#2797=CYLINDRICAL_SURFACE('',#35917,0.3);
#2798=CYLINDRICAL_SURFACE('',#35920,0.3);
#2799=CYLINDRICAL_SURFACE('',#35922,1.);
#2800=CYLINDRICAL_SURFACE('',#35925,0.1);
#2801=CYLINDRICAL_SURFACE('',#35930,0.1);
#2802=CYLINDRICAL_SURFACE('',#35936,0.0999999999999995);
#2803=CYLINDRICAL_SURFACE('',#35944,0.0999999999999999);
#2804=CYLINDRICAL_SURFACE('',#35950,0.1);
#2805=CYLINDRICAL_SURFACE('',#35953,0.0999999999999989);
#2806=CYLINDRICAL_SURFACE('',#35958,0.0999999999999999);
#2807=CYLINDRICAL_SURFACE('',#35967,0.1);
#2808=CYLINDRICAL_SURFACE('',#35972,0.1);
#2809=CYLINDRICAL_SURFACE('',#35977,0.1);
#2810=CYLINDRICAL_SURFACE('',#35982,0.1);
#2811=CYLINDRICAL_SURFACE('',#35987,0.1);
#2812=CYLINDRICAL_SURFACE('',#35989,0.1);
#2813=CYLINDRICAL_SURFACE('',#35992,0.1);
#2814=CYLINDRICAL_SURFACE('',#35998,0.1);
#2815=CYLINDRICAL_SURFACE('',#36000,0.1);
#2816=CYLINDRICAL_SURFACE('',#36003,0.1);
#2817=CYLINDRICAL_SURFACE('',#36009,0.1);
#2818=CYLINDRICAL_SURFACE('',#36020,2.95);
#2819=CYLINDRICAL_SURFACE('',#36025,2.95);
#2820=CYLINDRICAL_SURFACE('',#36030,2.95);
#2821=CYLINDRICAL_SURFACE('',#36034,2.95);
#2822=CYLINDRICAL_SURFACE('',#36039,0.299999999999999);
#2823=CYLINDRICAL_SURFACE('',#36045,0.3);
#2824=CYLINDRICAL_SURFACE('',#36046,0.5);
#2825=CYLINDRICAL_SURFACE('',#36053,1.);
#2826=CYLINDRICAL_SURFACE('',#36060,0.3);
#2827=CYLINDRICAL_SURFACE('',#36062,0.3);
#2828=CYLINDRICAL_SURFACE('',#36066,0.5);
#2829=CYLINDRICAL_SURFACE('',#36070,0.299999999999999);
#2830=CYLINDRICAL_SURFACE('',#36071,0.299999999999999);
#2831=CYLINDRICAL_SURFACE('',#36074,1.);
#2832=CYLINDRICAL_SURFACE('',#36077,0.5);
#2833=CYLINDRICAL_SURFACE('',#36080,0.5);
#2834=CYLINDRICAL_SURFACE('',#36083,0.5);
#2835=CYLINDRICAL_SURFACE('',#36092,0.1);
#2836=CYLINDRICAL_SURFACE('',#36101,0.1);
#2837=CYLINDRICAL_SURFACE('',#36104,2.65);
#2838=CYLINDRICAL_SURFACE('',#36110,0.100000000000001);
#2839=CYLINDRICAL_SURFACE('',#36124,0.0999999999999995);
#2840=CYLINDRICAL_SURFACE('',#36130,0.100000000000001);
#2841=CYLINDRICAL_SURFACE('',#36131,0.0999999999999995);
#2842=CYLINDRICAL_SURFACE('',#36132,0.1);
#2843=CYLINDRICAL_SURFACE('',#36138,0.0999999999999995);
#2844=CYLINDRICAL_SURFACE('',#36146,0.1);
#2845=CYLINDRICAL_SURFACE('',#36151,0.1);
#2846=CYLINDRICAL_SURFACE('',#36156,0.1);
#2847=CYLINDRICAL_SURFACE('',#36161,0.1);
#2848=CYLINDRICAL_SURFACE('',#36166,0.1);
#2849=CYLINDRICAL_SURFACE('',#36168,0.1);
#2850=CYLINDRICAL_SURFACE('',#36170,0.1);
#2851=CYLINDRICAL_SURFACE('',#36173,0.1);
#2852=CYLINDRICAL_SURFACE('',#36175,0.1);
#2853=CYLINDRICAL_SURFACE('',#36181,0.1);
#2854=CYLINDRICAL_SURFACE('',#36183,0.0999999999999994);
#2855=CYLINDRICAL_SURFACE('',#36185,0.1);
#2856=CYLINDRICAL_SURFACE('',#36188,0.1);
#2857=CYLINDRICAL_SURFACE('',#36190,0.1);
#2858=CYLINDRICAL_SURFACE('',#36196,0.1);
#2859=CYLINDRICAL_SURFACE('',#36209,0.3);
#2860=CYLINDRICAL_SURFACE('',#36219,0.3);
#2861=CYLINDRICAL_SURFACE('',#36226,0.299999999999999);
#2862=CYLINDRICAL_SURFACE('',#36232,0.3);
#2863=CYLINDRICAL_SURFACE('',#36249,1.4);
#2864=CYLINDRICAL_SURFACE('',#36251,0.0999999999999999);
#2865=CYLINDRICAL_SURFACE('',#36257,0.0999999999999989);
#2866=CYLINDRICAL_SURFACE('',#36263,0.1);
#2867=CYLINDRICAL_SURFACE('',#36267,1.);
#2868=CYLINDRICAL_SURFACE('',#36281,0.3);
#2869=CYLINDRICAL_SURFACE('',#36287,0.3);
#2870=CYLINDRICAL_SURFACE('',#36288,0.5);
#2871=CYLINDRICAL_SURFACE('',#36289,2.65);
#2872=CYLINDRICAL_SURFACE('',#36290,0.3);
#2873=CYLINDRICAL_SURFACE('',#36297,0.1);
#2874=CYLINDRICAL_SURFACE('',#36310,0.0999999999999999);
#2875=CYLINDRICAL_SURFACE('',#36314,0.5);
#2876=CYLINDRICAL_SURFACE('',#36316,1.);
#2877=CYLINDRICAL_SURFACE('',#36318,0.1);
#2878=CYLINDRICAL_SURFACE('',#36323,0.0999999999999998);
#2879=CYLINDRICAL_SURFACE('',#36328,0.0999999999999998);
#2880=CYLINDRICAL_SURFACE('',#36333,0.1);
#2881=CYLINDRICAL_SURFACE('',#36337,1.);
#2882=CYLINDRICAL_SURFACE('',#36339,1.);
#2883=CYLINDRICAL_SURFACE('',#36341,0.5);
#2884=CYLINDRICAL_SURFACE('',#36343,0.5);
#2885=CYLINDRICAL_SURFACE('',#36347,0.3);
#2886=CYLINDRICAL_SURFACE('',#36352,0.5);
#2887=CYLINDRICAL_SURFACE('',#36353,4.15);
#2888=CYLINDRICAL_SURFACE('',#36355,0.5);
#2889=CYLINDRICAL_SURFACE('',#36357,0.3);
#2890=CYLINDRICAL_SURFACE('',#36367,0.3);
#4126=FACE_OUTER_BOUND('',#6307,.T.);
#4127=FACE_OUTER_BOUND('',#6308,.T.);
#4128=FACE_OUTER_BOUND('',#6309,.T.);
#4129=FACE_OUTER_BOUND('',#6310,.T.);
#4130=FACE_OUTER_BOUND('',#6311,.T.);
#4131=FACE_OUTER_BOUND('',#6312,.T.);
#4132=FACE_OUTER_BOUND('',#6313,.T.);
#4133=FACE_OUTER_BOUND('',#6314,.T.);
#4134=FACE_OUTER_BOUND('',#6315,.T.);
#4135=FACE_OUTER_BOUND('',#6316,.T.);
#4136=FACE_OUTER_BOUND('',#6317,.T.);
#4137=FACE_OUTER_BOUND('',#6318,.T.);
#4138=FACE_OUTER_BOUND('',#6319,.T.);
#4139=FACE_OUTER_BOUND('',#6320,.T.);
#4140=FACE_OUTER_BOUND('',#6321,.T.);
#4141=FACE_OUTER_BOUND('',#6323,.T.);
#4142=FACE_OUTER_BOUND('',#6324,.T.);
#4143=FACE_OUTER_BOUND('',#6325,.T.);
#4144=FACE_OUTER_BOUND('',#6326,.T.);
#4145=FACE_OUTER_BOUND('',#6327,.T.);
#4146=FACE_OUTER_BOUND('',#6328,.T.);
#4147=FACE_OUTER_BOUND('',#6329,.T.);
#4148=FACE_OUTER_BOUND('',#6331,.T.);
#4149=FACE_OUTER_BOUND('',#6332,.T.);
#4150=FACE_OUTER_BOUND('',#6333,.T.);
#4151=FACE_OUTER_BOUND('',#6334,.T.);
#4152=FACE_OUTER_BOUND('',#6335,.T.);
#4153=FACE_OUTER_BOUND('',#6336,.T.);
#4154=FACE_OUTER_BOUND('',#6337,.T.);
#4155=FACE_OUTER_BOUND('',#6338,.T.);
#4156=FACE_OUTER_BOUND('',#6339,.T.);
#4157=FACE_OUTER_BOUND('',#6340,.T.);
#4158=FACE_OUTER_BOUND('',#6341,.T.);
#4159=FACE_OUTER_BOUND('',#6342,.T.);
#4160=FACE_OUTER_BOUND('',#6343,.T.);
#4161=FACE_OUTER_BOUND('',#6344,.T.);
#4162=FACE_OUTER_BOUND('',#6345,.T.);
#4163=FACE_OUTER_BOUND('',#6346,.T.);
#4164=FACE_OUTER_BOUND('',#6347,.T.);
#4165=FACE_OUTER_BOUND('',#6348,.T.);
#4166=FACE_OUTER_BOUND('',#6349,.T.);
#4167=FACE_OUTER_BOUND('',#6350,.T.);
#4168=FACE_OUTER_BOUND('',#6351,.T.);
#4169=FACE_OUTER_BOUND('',#6352,.T.);
#4170=FACE_OUTER_BOUND('',#6353,.T.);
#4171=FACE_OUTER_BOUND('',#6354,.T.);
#4172=FACE_OUTER_BOUND('',#6355,.T.);
#4173=FACE_OUTER_BOUND('',#6356,.T.);
#4174=FACE_OUTER_BOUND('',#6357,.T.);
#4175=FACE_OUTER_BOUND('',#6358,.T.);
#4176=FACE_OUTER_BOUND('',#6359,.T.);
#4177=FACE_OUTER_BOUND('',#6360,.T.);
#4178=FACE_OUTER_BOUND('',#6361,.T.);
#4179=FACE_OUTER_BOUND('',#6362,.T.);
#4180=FACE_OUTER_BOUND('',#6363,.T.);
#4181=FACE_OUTER_BOUND('',#6364,.T.);
#4182=FACE_OUTER_BOUND('',#6365,.T.);
#4183=FACE_OUTER_BOUND('',#6366,.T.);
#4184=FACE_OUTER_BOUND('',#6367,.T.);
#4185=FACE_OUTER_BOUND('',#6368,.T.);
#4186=FACE_OUTER_BOUND('',#6369,.T.);
#4187=FACE_OUTER_BOUND('',#6370,.T.);
#4188=FACE_OUTER_BOUND('',#6371,.T.);
#4189=FACE_OUTER_BOUND('',#6372,.T.);
#4190=FACE_OUTER_BOUND('',#6373,.T.);
#4191=FACE_OUTER_BOUND('',#6374,.T.);
#4192=FACE_OUTER_BOUND('',#6376,.T.);
#4193=FACE_OUTER_BOUND('',#6377,.T.);
#4194=FACE_OUTER_BOUND('',#6378,.T.);
#4195=FACE_OUTER_BOUND('',#6379,.T.);
#4196=FACE_OUTER_BOUND('',#6380,.T.);
#4197=FACE_OUTER_BOUND('',#6381,.T.);
#4198=FACE_OUTER_BOUND('',#6382,.T.);
#4199=FACE_OUTER_BOUND('',#6383,.T.);
#4200=FACE_OUTER_BOUND('',#6384,.T.);
#4201=FACE_OUTER_BOUND('',#6385,.T.);
#4202=FACE_OUTER_BOUND('',#6386,.T.);
#4203=FACE_OUTER_BOUND('',#6387,.T.);
#4204=FACE_OUTER_BOUND('',#6388,.T.);
#4205=FACE_OUTER_BOUND('',#6389,.T.);
#4206=FACE_OUTER_BOUND('',#6390,.T.);
#4207=FACE_OUTER_BOUND('',#6391,.T.);
#4208=FACE_OUTER_BOUND('',#6392,.T.);
#4209=FACE_OUTER_BOUND('',#6393,.T.);
#4210=FACE_OUTER_BOUND('',#6394,.T.);
#4211=FACE_OUTER_BOUND('',#6395,.T.);
#4212=FACE_OUTER_BOUND('',#6396,.T.);
#4213=FACE_OUTER_BOUND('',#6397,.T.);
#4214=FACE_OUTER_BOUND('',#6398,.T.);
#4215=FACE_OUTER_BOUND('',#6399,.T.);
#4216=FACE_OUTER_BOUND('',#6400,.T.);
#4217=FACE_OUTER_BOUND('',#6401,.T.);
#4218=FACE_OUTER_BOUND('',#6402,.T.);
#4219=FACE_OUTER_BOUND('',#6403,.T.);
#4220=FACE_OUTER_BOUND('',#6404,.T.);
#4221=FACE_OUTER_BOUND('',#6405,.T.);
#4222=FACE_OUTER_BOUND('',#6406,.T.);
#4223=FACE_OUTER_BOUND('',#6407,.T.);
#4224=FACE_OUTER_BOUND('',#6408,.T.);
#4225=FACE_OUTER_BOUND('',#6409,.T.);
#4226=FACE_OUTER_BOUND('',#6410,.T.);
#4227=FACE_OUTER_BOUND('',#6411,.T.);
#4228=FACE_OUTER_BOUND('',#6412,.T.);
#4229=FACE_OUTER_BOUND('',#6413,.T.);
#4230=FACE_OUTER_BOUND('',#6414,.T.);
#4231=FACE_OUTER_BOUND('',#6415,.T.);
#4232=FACE_OUTER_BOUND('',#6416,.T.);
#4233=FACE_OUTER_BOUND('',#6417,.T.);
#4234=FACE_OUTER_BOUND('',#6418,.T.);
#4235=FACE_OUTER_BOUND('',#6419,.T.);
#4236=FACE_OUTER_BOUND('',#6420,.T.);
#4237=FACE_OUTER_BOUND('',#6421,.T.);
#4238=FACE_OUTER_BOUND('',#6422,.T.);
#4239=FACE_OUTER_BOUND('',#6423,.T.);
#4240=FACE_OUTER_BOUND('',#6424,.T.);
#4241=FACE_OUTER_BOUND('',#6425,.T.);
#4242=FACE_OUTER_BOUND('',#6426,.T.);
#4243=FACE_OUTER_BOUND('',#6427,.T.);
#4244=FACE_OUTER_BOUND('',#6428,.T.);
#4245=FACE_OUTER_BOUND('',#6429,.T.);
#4246=FACE_OUTER_BOUND('',#6430,.T.);
#4247=FACE_OUTER_BOUND('',#6431,.T.);
#4248=FACE_OUTER_BOUND('',#6432,.T.);
#4249=FACE_OUTER_BOUND('',#6433,.T.);
#4250=FACE_OUTER_BOUND('',#6434,.T.);
#4251=FACE_OUTER_BOUND('',#6435,.T.);
#4252=FACE_OUTER_BOUND('',#6436,.T.);
#4253=FACE_OUTER_BOUND('',#6437,.T.);
#4254=FACE_OUTER_BOUND('',#6438,.T.);
#4255=FACE_OUTER_BOUND('',#6439,.T.);
#4256=FACE_OUTER_BOUND('',#6440,.T.);
#4257=FACE_OUTER_BOUND('',#6441,.T.);
#4258=FACE_OUTER_BOUND('',#6442,.T.);
#4259=FACE_OUTER_BOUND('',#6443,.T.);
#4260=FACE_OUTER_BOUND('',#6444,.T.);
#4261=FACE_OUTER_BOUND('',#6445,.T.);
#4262=FACE_OUTER_BOUND('',#6446,.T.);
#4263=FACE_OUTER_BOUND('',#6447,.T.);
#4264=FACE_OUTER_BOUND('',#6448,.T.);
#4265=FACE_OUTER_BOUND('',#6449,.T.);
#4266=FACE_OUTER_BOUND('',#6450,.T.);
#4267=FACE_OUTER_BOUND('',#6451,.T.);
#4268=FACE_OUTER_BOUND('',#6452,.T.);
#4269=FACE_OUTER_BOUND('',#6453,.T.);
#4270=FACE_OUTER_BOUND('',#6454,.T.);
#4271=FACE_OUTER_BOUND('',#6455,.T.);
#4272=FACE_OUTER_BOUND('',#6456,.T.);
#4273=FACE_OUTER_BOUND('',#6457,.T.);
#4274=FACE_OUTER_BOUND('',#6458,.T.);
#4275=FACE_OUTER_BOUND('',#6459,.T.);
#4276=FACE_OUTER_BOUND('',#6460,.T.);
#4277=FACE_OUTER_BOUND('',#6461,.T.);
#4278=FACE_OUTER_BOUND('',#6462,.T.);
#4279=FACE_OUTER_BOUND('',#6463,.T.);
#4280=FACE_OUTER_BOUND('',#6464,.T.);
#4281=FACE_OUTER_BOUND('',#6465,.T.);
#4282=FACE_OUTER_BOUND('',#6466,.T.);
#4283=FACE_OUTER_BOUND('',#6467,.T.);
#4284=FACE_OUTER_BOUND('',#6468,.T.);
#4285=FACE_OUTER_BOUND('',#6469,.T.);
#4286=FACE_OUTER_BOUND('',#6470,.T.);
#4287=FACE_OUTER_BOUND('',#6471,.T.);
#4288=FACE_OUTER_BOUND('',#6472,.T.);
#4289=FACE_OUTER_BOUND('',#6473,.T.);
#4290=FACE_OUTER_BOUND('',#6474,.T.);
#4291=FACE_OUTER_BOUND('',#6475,.T.);
#4292=FACE_OUTER_BOUND('',#6476,.T.);
#4293=FACE_OUTER_BOUND('',#6477,.T.);
#4294=FACE_OUTER_BOUND('',#6478,.T.);
#4295=FACE_OUTER_BOUND('',#6479,.T.);
#4296=FACE_OUTER_BOUND('',#6480,.T.);
#4297=FACE_OUTER_BOUND('',#6482,.T.);
#4298=FACE_OUTER_BOUND('',#6483,.T.);
#4299=FACE_OUTER_BOUND('',#6484,.T.);
#4300=FACE_OUTER_BOUND('',#6485,.T.);
#4301=FACE_OUTER_BOUND('',#6486,.T.);
#4302=FACE_OUTER_BOUND('',#6487,.T.);
#4303=FACE_OUTER_BOUND('',#6488,.T.);
#4304=FACE_OUTER_BOUND('',#6489,.T.);
#4305=FACE_OUTER_BOUND('',#6490,.T.);
#4306=FACE_OUTER_BOUND('',#6491,.T.);
#4307=FACE_OUTER_BOUND('',#6492,.T.);
#4308=FACE_OUTER_BOUND('',#6493,.T.);
#4309=FACE_OUTER_BOUND('',#6494,.T.);
#4310=FACE_OUTER_BOUND('',#6495,.T.);
#4311=FACE_OUTER_BOUND('',#6496,.T.);
#4312=FACE_OUTER_BOUND('',#6497,.T.);
#4313=FACE_OUTER_BOUND('',#6498,.T.);
#4314=FACE_OUTER_BOUND('',#6499,.T.);
#4315=FACE_OUTER_BOUND('',#6500,.T.);
#4316=FACE_OUTER_BOUND('',#6501,.T.);
#4317=FACE_OUTER_BOUND('',#6502,.T.);
#4318=FACE_OUTER_BOUND('',#6503,.T.);
#4319=FACE_OUTER_BOUND('',#6504,.T.);
#4320=FACE_OUTER_BOUND('',#6505,.T.);
#4321=FACE_OUTER_BOUND('',#6506,.T.);
#4322=FACE_OUTER_BOUND('',#6507,.T.);
#4323=FACE_OUTER_BOUND('',#6508,.T.);
#4324=FACE_OUTER_BOUND('',#6509,.T.);
#4325=FACE_OUTER_BOUND('',#6510,.T.);
#4326=FACE_OUTER_BOUND('',#6511,.T.);
#4327=FACE_OUTER_BOUND('',#6512,.T.);
#4328=FACE_OUTER_BOUND('',#6513,.T.);
#4329=FACE_OUTER_BOUND('',#6514,.T.);
#4330=FACE_OUTER_BOUND('',#6515,.T.);
#4331=FACE_OUTER_BOUND('',#6517,.T.);
#4332=FACE_OUTER_BOUND('',#6518,.T.);
#4333=FACE_OUTER_BOUND('',#6519,.T.);
#4334=FACE_OUTER_BOUND('',#6520,.T.);
#4335=FACE_OUTER_BOUND('',#6521,.T.);
#4336=FACE_OUTER_BOUND('',#6522,.T.);
#4337=FACE_OUTER_BOUND('',#6523,.T.);
#4338=FACE_OUTER_BOUND('',#6524,.T.);
#4339=FACE_OUTER_BOUND('',#6525,.T.);
#4340=FACE_OUTER_BOUND('',#6526,.T.);
#4341=FACE_OUTER_BOUND('',#6527,.T.);
#4342=FACE_OUTER_BOUND('',#6528,.T.);
#4343=FACE_OUTER_BOUND('',#6529,.T.);
#4344=FACE_OUTER_BOUND('',#6530,.T.);
#4345=FACE_OUTER_BOUND('',#6531,.T.);
#4346=FACE_OUTER_BOUND('',#6532,.T.);
#4347=FACE_OUTER_BOUND('',#6533,.T.);
#4348=FACE_OUTER_BOUND('',#6534,.T.);
#4349=FACE_OUTER_BOUND('',#6535,.T.);
#4350=FACE_OUTER_BOUND('',#6536,.T.);
#4351=FACE_OUTER_BOUND('',#6537,.T.);
#4352=FACE_OUTER_BOUND('',#6538,.T.);
#4353=FACE_OUTER_BOUND('',#6539,.T.);
#4354=FACE_OUTER_BOUND('',#6540,.T.);
#4355=FACE_OUTER_BOUND('',#6541,.T.);
#4356=FACE_OUTER_BOUND('',#6542,.T.);
#4357=FACE_OUTER_BOUND('',#6543,.T.);
#4358=FACE_OUTER_BOUND('',#6544,.T.);
#4359=FACE_OUTER_BOUND('',#6545,.T.);
#4360=FACE_OUTER_BOUND('',#6546,.T.);
#4361=FACE_OUTER_BOUND('',#6547,.T.);
#4362=FACE_OUTER_BOUND('',#6548,.T.);
#4363=FACE_OUTER_BOUND('',#6549,.T.);
#4364=FACE_OUTER_BOUND('',#6550,.T.);
#4365=FACE_OUTER_BOUND('',#6552,.T.);
#4366=FACE_OUTER_BOUND('',#6553,.T.);
#4367=FACE_OUTER_BOUND('',#6554,.T.);
#4368=FACE_OUTER_BOUND('',#6555,.T.);
#4369=FACE_OUTER_BOUND('',#6556,.T.);
#4370=FACE_OUTER_BOUND('',#6557,.T.);
#4371=FACE_OUTER_BOUND('',#6558,.T.);
#4372=FACE_OUTER_BOUND('',#6559,.T.);
#4373=FACE_OUTER_BOUND('',#6560,.T.);
#4374=FACE_OUTER_BOUND('',#6561,.T.);
#4375=FACE_OUTER_BOUND('',#6562,.T.);
#4376=FACE_OUTER_BOUND('',#6563,.T.);
#4377=FACE_OUTER_BOUND('',#6564,.T.);
#4378=FACE_OUTER_BOUND('',#6565,.T.);
#4379=FACE_OUTER_BOUND('',#6566,.T.);
#4380=FACE_OUTER_BOUND('',#6567,.T.);
#4381=FACE_OUTER_BOUND('',#6568,.T.);
#4382=FACE_OUTER_BOUND('',#6569,.T.);
#4383=FACE_OUTER_BOUND('',#6570,.T.);
#4384=FACE_OUTER_BOUND('',#6571,.T.);
#4385=FACE_OUTER_BOUND('',#6572,.T.);
#4386=FACE_OUTER_BOUND('',#6573,.T.);
#4387=FACE_OUTER_BOUND('',#6574,.T.);
#4388=FACE_OUTER_BOUND('',#6575,.T.);
#4389=FACE_OUTER_BOUND('',#6576,.T.);
#4390=FACE_OUTER_BOUND('',#6577,.T.);
#4391=FACE_OUTER_BOUND('',#6578,.T.);
#4392=FACE_OUTER_BOUND('',#6579,.T.);
#4393=FACE_OUTER_BOUND('',#6580,.T.);
#4394=FACE_OUTER_BOUND('',#6581,.T.);
#4395=FACE_OUTER_BOUND('',#6582,.T.);
#4396=FACE_OUTER_BOUND('',#6583,.T.);
#4397=FACE_OUTER_BOUND('',#6584,.T.);
#4398=FACE_OUTER_BOUND('',#6585,.T.);
#4399=FACE_OUTER_BOUND('',#6586,.T.);
#4400=FACE_OUTER_BOUND('',#6587,.T.);
#4401=FACE_OUTER_BOUND('',#6588,.T.);
#4402=FACE_OUTER_BOUND('',#6589,.T.);
#4403=FACE_OUTER_BOUND('',#6590,.T.);
#4404=FACE_OUTER_BOUND('',#6591,.T.);
#4405=FACE_OUTER_BOUND('',#6592,.T.);
#4406=FACE_OUTER_BOUND('',#6593,.T.);
#4407=FACE_OUTER_BOUND('',#6594,.T.);
#4408=FACE_OUTER_BOUND('',#6595,.T.);
#4409=FACE_OUTER_BOUND('',#6596,.T.);
#4410=FACE_OUTER_BOUND('',#6597,.T.);
#4411=FACE_OUTER_BOUND('',#6598,.T.);
#4412=FACE_OUTER_BOUND('',#6599,.T.);
#4413=FACE_OUTER_BOUND('',#6600,.T.);
#4414=FACE_OUTER_BOUND('',#6601,.T.);
#4415=FACE_OUTER_BOUND('',#6602,.T.);
#4416=FACE_OUTER_BOUND('',#6603,.T.);
#4417=FACE_OUTER_BOUND('',#6604,.T.);
#6307=EDGE_LOOP('',(#26017,#26018,#26019,#26020,#26021,#26022));
#6308=EDGE_LOOP('',(#26023,#26024,#26025,#26026,#26027,#26028));
#6309=EDGE_LOOP('',(#26029,#26030,#26031,#26032,#26033,#26034));
#6310=EDGE_LOOP('',(#26035,#26036,#26037,#26038,#26039,#26040));
#6311=EDGE_LOOP('',(#26041,#26042,#26043,#26044,#26045,#26046));
#6312=EDGE_LOOP('',(#26047,#26048,#26049,#26050,#26051,#26052));
#6313=EDGE_LOOP('',(#26053,#26054));
#6314=EDGE_LOOP('',(#26055,#26056,#26057,#26058));
#6315=EDGE_LOOP('',(#26059,#26060,#26061,#26062));
#6316=EDGE_LOOP('',(#26063,#26064,#26065,#26066));
#6317=EDGE_LOOP('',(#26067,#26068));
#6318=EDGE_LOOP('',(#26069,#26070,#26071));
#6319=EDGE_LOOP('',(#26072,#26073,#26074,#26075));
#6320=EDGE_LOOP('',(#26076,#26077,#26078,#26079));
#6321=EDGE_LOOP('',(#26080,#26081,#26082,#26083,#26084,#26085,#26086,#26087,
#26088,#26089,#26090));
#6322=EDGE_LOOP('',(#26091,#26092,#26093,#26094,#26095,#26096,#26097,#26098,
#26099,#26100,#26101,#26102,#26103,#26104,#26105,#26106,#26107,#26108,#26109,
#26110,#26111,#26112,#26113,#26114,#26115,#26116));
#6323=EDGE_LOOP('',(#26117,#26118,#26119));
#6324=EDGE_LOOP('',(#26120,#26121,#26122,#26123));
#6325=EDGE_LOOP('',(#26124,#26125,#26126,#26127));
#6326=EDGE_LOOP('',(#26128,#26129,#26130,#26131,#26132));
#6327=EDGE_LOOP('',(#26133));
#6328=EDGE_LOOP('',(#26134,#26135,#26136,#26137));
#6329=EDGE_LOOP('',(#26138,#26139,#26140,#26141,#26142,#26143,#26144,#26145));
#6330=EDGE_LOOP('',(#26146));
#6331=EDGE_LOOP('',(#26147,#26148,#26149,#26150));
#6332=EDGE_LOOP('',(#26151,#26152,#26153,#26154));
#6333=EDGE_LOOP('',(#26155,#26156,#26157,#26158));
#6334=EDGE_LOOP('',(#26159,#26160,#26161,#26162));
#6335=EDGE_LOOP('',(#26163,#26164,#26165,#26166));
#6336=EDGE_LOOP('',(#26167,#26168,#26169,#26170));
#6337=EDGE_LOOP('',(#26171,#26172,#26173,#26174));
#6338=EDGE_LOOP('',(#26175,#26176,#26177,#26178,#26179,#26180,#26181,#26182));
#6339=EDGE_LOOP('',(#26183,#26184,#26185,#26186,#26187));
#6340=EDGE_LOOP('',(#26188,#26189,#26190,#26191));
#6341=EDGE_LOOP('',(#26192,#26193,#26194,#26195));
#6342=EDGE_LOOP('',(#26196,#26197,#26198,#26199));
#6343=EDGE_LOOP('',(#26200,#26201,#26202,#26203));
#6344=EDGE_LOOP('',(#26204,#26205,#26206,#26207));
#6345=EDGE_LOOP('',(#26208,#26209,#26210,#26211));
#6346=EDGE_LOOP('',(#26212,#26213,#26214,#26215));
#6347=EDGE_LOOP('',(#26216,#26217,#26218,#26219,#26220,#26221,#26222,#26223));
#6348=EDGE_LOOP('',(#26224,#26225,#26226,#26227));
#6349=EDGE_LOOP('',(#26228,#26229,#26230,#26231));
#6350=EDGE_LOOP('',(#26232,#26233,#26234));
#6351=EDGE_LOOP('',(#26235,#26236,#26237,#26238));
#6352=EDGE_LOOP('',(#26239,#26240,#26241));
#6353=EDGE_LOOP('',(#26242,#26243,#26244,#26245));
#6354=EDGE_LOOP('',(#26246,#26247,#26248,#26249));
#6355=EDGE_LOOP('',(#26250,#26251,#26252,#26253));
#6356=EDGE_LOOP('',(#26254,#26255,#26256,#26257));
#6357=EDGE_LOOP('',(#26258,#26259,#26260,#26261));
#6358=EDGE_LOOP('',(#26262,#26263,#26264,#26265));
#6359=EDGE_LOOP('',(#26266,#26267,#26268,#26269));
#6360=EDGE_LOOP('',(#26270,#26271,#26272,#26273));
#6361=EDGE_LOOP('',(#26274,#26275,#26276,#26277));
#6362=EDGE_LOOP('',(#26278,#26279,#26280,#26281));
#6363=EDGE_LOOP('',(#26282,#26283,#26284,#26285));
#6364=EDGE_LOOP('',(#26286,#26287,#26288,#26289));
#6365=EDGE_LOOP('',(#26290,#26291,#26292,#26293,#26294,#26295,#26296));
#6366=EDGE_LOOP('',(#26297,#26298,#26299,#26300));
#6367=EDGE_LOOP('',(#26301,#26302,#26303,#26304));
#6368=EDGE_LOOP('',(#26305,#26306,#26307,#26308));
#6369=EDGE_LOOP('',(#26309,#26310,#26311,#26312));
#6370=EDGE_LOOP('',(#26313,#26314,#26315,#26316));
#6371=EDGE_LOOP('',(#26317,#26318,#26319,#26320,#26321,#26322,#26323,#26324,
#26325,#26326,#26327,#26328,#26329,#26330,#26331,#26332,#26333,#26334,#26335,
#26336,#26337,#26338,#26339,#26340,#26341,#26342,#26343,#26344,#26345,#26346,
#26347,#26348,#26349,#26350,#26351,#26352,#26353,#26354,#26355,#26356,#26357));
#6372=EDGE_LOOP('',(#26358,#26359,#26360));
#6373=EDGE_LOOP('',(#26361,#26362,#26363,#26364));
#6374=EDGE_LOOP('',(#26365,#26366,#26367,#26368,#26369,#26370,#26371,#26372,
#26373,#26374,#26375));
#6375=EDGE_LOOP('',(#26376));
#6376=EDGE_LOOP('',(#26377,#26378,#26379,#26380));
#6377=EDGE_LOOP('',(#26381,#26382,#26383,#26384));
#6378=EDGE_LOOP('',(#26385,#26386,#26387,#26388));
#6379=EDGE_LOOP('',(#26389,#26390,#26391,#26392));
#6380=EDGE_LOOP('',(#26393,#26394,#26395,#26396));
#6381=EDGE_LOOP('',(#26397,#26398,#26399,#26400));
#6382=EDGE_LOOP('',(#26401,#26402,#26403,#26404));
#6383=EDGE_LOOP('',(#26405,#26406,#26407,#26408));
#6384=EDGE_LOOP('',(#26409,#26410,#26411,#26412));
#6385=EDGE_LOOP('',(#26413,#26414,#26415,#26416));
#6386=EDGE_LOOP('',(#26417,#26418,#26419,#26420));
#6387=EDGE_LOOP('',(#26421,#26422,#26423,#26424));
#6388=EDGE_LOOP('',(#26425,#26426,#26427,#26428));
#6389=EDGE_LOOP('',(#26429,#26430,#26431,#26432));
#6390=EDGE_LOOP('',(#26433,#26434,#26435,#26436));
#6391=EDGE_LOOP('',(#26437,#26438,#26439,#26440));
#6392=EDGE_LOOP('',(#26441,#26442,#26443,#26444));
#6393=EDGE_LOOP('',(#26445,#26446,#26447,#26448));
#6394=EDGE_LOOP('',(#26449,#26450,#26451,#26452));
#6395=EDGE_LOOP('',(#26453,#26454,#26455,#26456));
#6396=EDGE_LOOP('',(#26457,#26458,#26459,#26460));
#6397=EDGE_LOOP('',(#26461,#26462,#26463,#26464));
#6398=EDGE_LOOP('',(#26465,#26466,#26467,#26468));
#6399=EDGE_LOOP('',(#26469,#26470,#26471,#26472));
#6400=EDGE_LOOP('',(#26473,#26474,#26475,#26476));
#6401=EDGE_LOOP('',(#26477,#26478,#26479,#26480));
#6402=EDGE_LOOP('',(#26481,#26482,#26483,#26484));
#6403=EDGE_LOOP('',(#26485,#26486,#26487,#26488));
#6404=EDGE_LOOP('',(#26489,#26490,#26491,#26492));
#6405=EDGE_LOOP('',(#26493,#26494,#26495,#26496));
#6406=EDGE_LOOP('',(#26497,#26498,#26499,#26500));
#6407=EDGE_LOOP('',(#26501,#26502,#26503,#26504));
#6408=EDGE_LOOP('',(#26505,#26506,#26507,#26508));
#6409=EDGE_LOOP('',(#26509,#26510,#26511,#26512));
#6410=EDGE_LOOP('',(#26513,#26514,#26515,#26516));
#6411=EDGE_LOOP('',(#26517,#26518,#26519,#26520));
#6412=EDGE_LOOP('',(#26521,#26522,#26523,#26524));
#6413=EDGE_LOOP('',(#26525,#26526,#26527,#26528));
#6414=EDGE_LOOP('',(#26529,#26530,#26531,#26532));
#6415=EDGE_LOOP('',(#26533,#26534,#26535,#26536));
#6416=EDGE_LOOP('',(#26537,#26538,#26539,#26540,#26541));
#6417=EDGE_LOOP('',(#26542,#26543,#26544,#26545));
#6418=EDGE_LOOP('',(#26546,#26547,#26548,#26549));
#6419=EDGE_LOOP('',(#26550,#26551,#26552,#26553));
#6420=EDGE_LOOP('',(#26554,#26555,#26556,#26557));
#6421=EDGE_LOOP('',(#26558,#26559,#26560,#26561));
#6422=EDGE_LOOP('',(#26562,#26563,#26564,#26565));
#6423=EDGE_LOOP('',(#26566,#26567,#26568,#26569));
#6424=EDGE_LOOP('',(#26570,#26571,#26572,#26573));
#6425=EDGE_LOOP('',(#26574,#26575,#26576,#26577));
#6426=EDGE_LOOP('',(#26578,#26579,#26580));
#6427=EDGE_LOOP('',(#26581,#26582,#26583,#26584));
#6428=EDGE_LOOP('',(#26585,#26586,#26587));
#6429=EDGE_LOOP('',(#26588,#26589,#26590,#26591));
#6430=EDGE_LOOP('',(#26592,#26593,#26594,#26595));
#6431=EDGE_LOOP('',(#26596,#26597,#26598,#26599,#26600));
#6432=EDGE_LOOP('',(#26601,#26602,#26603,#26604,#26605));
#6433=EDGE_LOOP('',(#26606,#26607,#26608));
#6434=EDGE_LOOP('',(#26609,#26610,#26611,#26612));
#6435=EDGE_LOOP('',(#26613,#26614,#26615,#26616,#26617));
#6436=EDGE_LOOP('',(#26618,#26619,#26620,#26621));
#6437=EDGE_LOOP('',(#26622,#26623,#26624,#26625));
#6438=EDGE_LOOP('',(#26626,#26627,#26628,#26629));
#6439=EDGE_LOOP('',(#26630,#26631,#26632,#26633,#26634,#26635));
#6440=EDGE_LOOP('',(#26636,#26637,#26638,#26639));
#6441=EDGE_LOOP('',(#26640,#26641,#26642,#26643));
#6442=EDGE_LOOP('',(#26644,#26645,#26646,#26647));
#6443=EDGE_LOOP('',(#26648,#26649,#26650,#26651));
#6444=EDGE_LOOP('',(#26652,#26653,#26654));
#6445=EDGE_LOOP('',(#26655,#26656,#26657,#26658));
#6446=EDGE_LOOP('',(#26659,#26660,#26661,#26662,#26663));
#6447=EDGE_LOOP('',(#26664,#26665,#26666,#26667));
#6448=EDGE_LOOP('',(#26668,#26669,#26670,#26671));
#6449=EDGE_LOOP('',(#26672,#26673,#26674));
#6450=EDGE_LOOP('',(#26675,#26676,#26677,#26678,#26679));
#6451=EDGE_LOOP('',(#26680,#26681,#26682,#26683));
#6452=EDGE_LOOP('',(#26684,#26685,#26686,#26687,#26688));
#6453=EDGE_LOOP('',(#26689,#26690,#26691,#26692));
#6454=EDGE_LOOP('',(#26693,#26694,#26695,#26696,#26697,#26698));
#6455=EDGE_LOOP('',(#26699,#26700,#26701,#26702));
#6456=EDGE_LOOP('',(#26703,#26704,#26705,#26706));
#6457=EDGE_LOOP('',(#26707,#26708,#26709,#26710));
#6458=EDGE_LOOP('',(#26711,#26712,#26713,#26714));
#6459=EDGE_LOOP('',(#26715,#26716,#26717,#26718));
#6460=EDGE_LOOP('',(#26719,#26720,#26721,#26722));
#6461=EDGE_LOOP('',(#26723,#26724,#26725,#26726));
#6462=EDGE_LOOP('',(#26727,#26728,#26729,#26730));
#6463=EDGE_LOOP('',(#26731,#26732,#26733));
#6464=EDGE_LOOP('',(#26734,#26735,#26736,#26737));
#6465=EDGE_LOOP('',(#26738,#26739,#26740));
#6466=EDGE_LOOP('',(#26741,#26742,#26743,#26744));
#6467=EDGE_LOOP('',(#26745,#26746,#26747,#26748));
#6468=EDGE_LOOP('',(#26749,#26750,#26751,#26752));
#6469=EDGE_LOOP('',(#26753,#26754,#26755));
#6470=EDGE_LOOP('',(#26756,#26757,#26758,#26759));
#6471=EDGE_LOOP('',(#26760,#26761,#26762));
#6472=EDGE_LOOP('',(#26763,#26764,#26765,#26766));
#6473=EDGE_LOOP('',(#26767,#26768,#26769,#26770));
#6474=EDGE_LOOP('',(#26771,#26772,#26773,#26774));
#6475=EDGE_LOOP('',(#26775,#26776,#26777,#26778,#26779));
#6476=EDGE_LOOP('',(#26780,#26781,#26782,#26783));
#6477=EDGE_LOOP('',(#26784,#26785,#26786,#26787,#26788));
#6478=EDGE_LOOP('',(#26789,#26790,#26791,#26792));
#6479=EDGE_LOOP('',(#26793,#26794,#26795,#26796));
#6480=EDGE_LOOP('',(#26797,#26798,#26799,#26800,#26801,#26802,#26803,#26804,
#26805,#26806,#26807));
#6481=EDGE_LOOP('',(#26808));
#6482=EDGE_LOOP('',(#26809,#26810,#26811,#26812,#26813));
#6483=EDGE_LOOP('',(#26814,#26815,#26816,#26817));
#6484=EDGE_LOOP('',(#26818,#26819,#26820));
#6485=EDGE_LOOP('',(#26821,#26822,#26823,#26824,#26825));
#6486=EDGE_LOOP('',(#26826,#26827,#26828,#26829));
#6487=EDGE_LOOP('',(#26830,#26831,#26832,#26833,#26834));
#6488=EDGE_LOOP('',(#26835,#26836,#26837,#26838));
#6489=EDGE_LOOP('',(#26839,#26840,#26841,#26842));
#6490=EDGE_LOOP('',(#26843,#26844,#26845,#26846));
#6491=EDGE_LOOP('',(#26847,#26848,#26849,#26850));
#6492=EDGE_LOOP('',(#26851,#26852,#26853,#26854));
#6493=EDGE_LOOP('',(#26855,#26856,#26857,#26858));
#6494=EDGE_LOOP('',(#26859,#26860,#26861,#26862));
#6495=EDGE_LOOP('',(#26863,#26864,#26865,#26866));
#6496=EDGE_LOOP('',(#26867,#26868,#26869,#26870));
#6497=EDGE_LOOP('',(#26871,#26872,#26873,#26874));
#6498=EDGE_LOOP('',(#26875,#26876,#26877,#26878));
#6499=EDGE_LOOP('',(#26879,#26880,#26881,#26882));
#6500=EDGE_LOOP('',(#26883,#26884,#26885,#26886));
#6501=EDGE_LOOP('',(#26887,#26888,#26889,#26890));
#6502=EDGE_LOOP('',(#26891,#26892,#26893,#26894));
#6503=EDGE_LOOP('',(#26895,#26896,#26897,#26898));
#6504=EDGE_LOOP('',(#26899,#26900,#26901,#26902));
#6505=EDGE_LOOP('',(#26903,#26904,#26905,#26906));
#6506=EDGE_LOOP('',(#26907,#26908,#26909,#26910));
#6507=EDGE_LOOP('',(#26911,#26912,#26913,#26914));
#6508=EDGE_LOOP('',(#26915,#26916,#26917,#26918));
#6509=EDGE_LOOP('',(#26919,#26920,#26921,#26922));
#6510=EDGE_LOOP('',(#26923,#26924,#26925,#26926));
#6511=EDGE_LOOP('',(#26927,#26928,#26929,#26930));
#6512=EDGE_LOOP('',(#26931,#26932,#26933,#26934));
#6513=EDGE_LOOP('',(#26935,#26936,#26937,#26938));
#6514=EDGE_LOOP('',(#26939,#26940,#26941,#26942));
#6515=EDGE_LOOP('',(#26943));
#6516=EDGE_LOOP('',(#26944));
#6517=EDGE_LOOP('',(#26945,#26946,#26947));
#6518=EDGE_LOOP('',(#26948,#26949,#26950,#26951,#26952));
#6519=EDGE_LOOP('',(#26953,#26954,#26955,#26956));
#6520=EDGE_LOOP('',(#26957,#26958,#26959,#26960));
#6521=EDGE_LOOP('',(#26961,#26962,#26963,#26964));
#6522=EDGE_LOOP('',(#26965,#26966,#26967,#26968));
#6523=EDGE_LOOP('',(#26969,#26970,#26971,#26972));
#6524=EDGE_LOOP('',(#26973,#26974,#26975,#26976));
#6525=EDGE_LOOP('',(#26977,#26978,#26979,#26980));
#6526=EDGE_LOOP('',(#26981,#26982,#26983));
#6527=EDGE_LOOP('',(#26984,#26985,#26986,#26987));
#6528=EDGE_LOOP('',(#26988,#26989,#26990));
#6529=EDGE_LOOP('',(#26991,#26992,#26993,#26994));
#6530=EDGE_LOOP('',(#26995,#26996,#26997,#26998));
#6531=EDGE_LOOP('',(#26999,#27000,#27001,#27002));
#6532=EDGE_LOOP('',(#27003,#27004,#27005,#27006));
#6533=EDGE_LOOP('',(#27007,#27008,#27009,#27010));
#6534=EDGE_LOOP('',(#27011,#27012,#27013,#27014,#27015,#27016,#27017));
#6535=EDGE_LOOP('',(#27018,#27019,#27020));
#6536=EDGE_LOOP('',(#27021,#27022,#27023));
#6537=EDGE_LOOP('',(#27024,#27025,#27026));
#6538=EDGE_LOOP('',(#27027,#27028,#27029));
#6539=EDGE_LOOP('',(#27030,#27031,#27032,#27033));
#6540=EDGE_LOOP('',(#27034,#27035,#27036,#27037));
#6541=EDGE_LOOP('',(#27038,#27039,#27040,#27041));
#6542=EDGE_LOOP('',(#27042,#27043,#27044,#27045));
#6543=EDGE_LOOP('',(#27046,#27047,#27048,#27049));
#6544=EDGE_LOOP('',(#27050,#27051,#27052,#27053));
#6545=EDGE_LOOP('',(#27054,#27055,#27056));
#6546=EDGE_LOOP('',(#27057,#27058,#27059,#27060));
#6547=EDGE_LOOP('',(#27061,#27062,#27063,#27064));
#6548=EDGE_LOOP('',(#27065,#27066,#27067,#27068,#27069));
#6549=EDGE_LOOP('',(#27070,#27071,#27072,#27073));
#6550=EDGE_LOOP('',(#27074,#27075,#27076));
#6551=EDGE_LOOP('',(#27077));
#6552=EDGE_LOOP('',(#27078,#27079,#27080,#27081));
#6553=EDGE_LOOP('',(#27082,#27083,#27084,#27085));
#6554=EDGE_LOOP('',(#27086,#27087,#27088,#27089));
#6555=EDGE_LOOP('',(#27090,#27091,#27092,#27093));
#6556=EDGE_LOOP('',(#27094,#27095,#27096,#27097,#27098));
#6557=EDGE_LOOP('',(#27099,#27100,#27101,#27102));
#6558=EDGE_LOOP('',(#27103,#27104,#27105,#27106));
#6559=EDGE_LOOP('',(#27107,#27108,#27109,#27110));
#6560=EDGE_LOOP('',(#27111,#27112,#27113,#27114));
#6561=EDGE_LOOP('',(#27115,#27116,#27117,#27118));
#6562=EDGE_LOOP('',(#27119,#27120,#27121,#27122,#27123,#27124,#27125,#27126,
#27127,#27128,#27129,#27130,#27131,#27132,#27133,#27134,#27135,#27136,#27137,
#27138,#27139,#27140,#27141,#27142,#27143,#27144,#27145,#27146,#27147,#27148,
#27149,#27150,#27151,#27152,#27153,#27154,#27155,#27156,#27157,#27158,#27159));
#6563=EDGE_LOOP('',(#27160,#27161,#27162,#27163));
#6564=EDGE_LOOP('',(#27164,#27165,#27166));
#6565=EDGE_LOOP('',(#27167,#27168,#27169,#27170));
#6566=EDGE_LOOP('',(#27171,#27172,#27173,#27174));
#6567=EDGE_LOOP('',(#27175,#27176,#27177,#27178,#27179));
#6568=EDGE_LOOP('',(#27180,#27181,#27182,#27183,#27184));
#6569=EDGE_LOOP('',(#27185,#27186,#27187,#27188));
#6570=EDGE_LOOP('',(#27189,#27190,#27191,#27192));
#6571=EDGE_LOOP('',(#27193,#27194,#27195,#27196,#27197,#27198,#27199,#27200));
#6572=EDGE_LOOP('',(#27201,#27202,#27203,#27204));
#6573=EDGE_LOOP('',(#27205,#27206,#27207,#27208));
#6574=EDGE_LOOP('',(#27209,#27210,#27211,#27212));
#6575=EDGE_LOOP('',(#27213,#27214,#27215,#27216));
#6576=EDGE_LOOP('',(#27217,#27218,#27219,#27220));
#6577=EDGE_LOOP('',(#27221,#27222,#27223,#27224));
#6578=EDGE_LOOP('',(#27225,#27226,#27227,#27228));
#6579=EDGE_LOOP('',(#27229,#27230,#27231,#27232));
#6580=EDGE_LOOP('',(#27233,#27234,#27235,#27236));
#6581=EDGE_LOOP('',(#27237,#27238,#27239,#27240,#27241));
#6582=EDGE_LOOP('',(#27242,#27243,#27244,#27245));
#6583=EDGE_LOOP('',(#27246,#27247,#27248,#27249));
#6584=EDGE_LOOP('',(#27250,#27251,#27252,#27253));
#6585=EDGE_LOOP('',(#27254,#27255,#27256,#27257));
#6586=EDGE_LOOP('',(#27258,#27259,#27260,#27261));
#6587=EDGE_LOOP('',(#27262,#27263,#27264,#27265));
#6588=EDGE_LOOP('',(#27266,#27267,#27268,#27269));
#6589=EDGE_LOOP('',(#27270,#27271,#27272,#27273));
#6590=EDGE_LOOP('',(#27274,#27275,#27276,#27277));
#6591=EDGE_LOOP('',(#27278,#27279,#27280));
#6592=EDGE_LOOP('',(#27281,#27282,#27283,#27284));
#6593=EDGE_LOOP('',(#27285,#27286,#27287,#27288));
#6594=EDGE_LOOP('',(#27289,#27290,#27291,#27292));
#6595=EDGE_LOOP('',(#27293,#27294,#27295,#27296));
#6596=EDGE_LOOP('',(#27297,#27298,#27299,#27300,#27301,#27302,#27303));
#6597=EDGE_LOOP('',(#27304,#27305,#27306,#27307));
#6598=EDGE_LOOP('',(#27308,#27309,#27310,#27311));
#6599=EDGE_LOOP('',(#27312,#27313,#27314));
#6600=EDGE_LOOP('',(#27315,#27316,#27317,#27318,#27319,#27320,#27321,#27322));
#6601=EDGE_LOOP('',(#27323,#27324,#27325,#27326));
#6602=EDGE_LOOP('',(#27327,#27328,#27329,#27330));
#6603=EDGE_LOOP('',(#27331,#27332,#27333,#27334));
#6604=EDGE_LOOP('',(#27335,#27336,#27337,#27338,#27339,#27340,#27341,#27342));
#8446=LINE('',#78996,#10286);
#8447=LINE('',#79068,#10287);
#8448=LINE('',#79139,#10288);
#8449=LINE('',#79165,#10289);
#8450=LINE('',#79756,#10290);
#8451=LINE('',#79763,#10291);
#8452=LINE('',#79767,#10292);
#8453=LINE('',#79771,#10293);
#8454=LINE('',#79774,#10294);
#8455=LINE('',#79779,#10295);
#8456=LINE('',#79788,#10296);
#8457=LINE('',#79804,#10297);
#8458=LINE('',#79820,#10298);
#8459=LINE('',#79883,#10299);
#8460=LINE('',#79885,#10300);
#8461=LINE('',#79923,#10301);
#8462=LINE('',#79963,#10302);
#8463=LINE('',#79967,#10303);
#8464=LINE('',#79968,#10304);
#8465=LINE('',#79972,#10305);
#8466=LINE('',#79975,#10306);
#8467=LINE('',#79976,#10307);
#8468=LINE('',#79980,#10308);
#8469=LINE('',#80087,#10309);
#8470=LINE('',#80089,#10310);
#8471=LINE('',#80091,#10311);
#8472=LINE('',#80092,#10312);
#8473=LINE('',#80212,#10313);
#8474=LINE('',#80213,#10314);
#8475=LINE('',#80238,#10315);
#8476=LINE('',#80243,#10316);
#8477=LINE('',#80251,#10317);
#8478=LINE('',#80259,#10318);
#8479=LINE('',#80322,#10319);
#8480=LINE('',#80326,#10320);
#8481=LINE('',#80334,#10321);
#8482=LINE('',#80338,#10322);
#8483=LINE('',#80341,#10323);
#8484=LINE('',#80343,#10324);
#8485=LINE('',#80345,#10325);
#8486=LINE('',#80347,#10326);
#8487=LINE('',#80460,#10327);
#8488=LINE('',#80477,#10328);
#8489=LINE('',#80481,#10329);
#8490=LINE('',#80483,#10330);
#8491=LINE('',#80485,#10331);
#8492=LINE('',#80489,#10332);
#8493=LINE('',#80491,#10333);
#8494=LINE('',#80493,#10334);
#8495=LINE('',#80497,#10335);
#8496=LINE('',#80501,#10336);
#8497=LINE('',#80505,#10337);
#8498=LINE('',#80509,#10338);
#8499=LINE('',#80515,#10339);
#8500=LINE('',#80519,#10340);
#8501=LINE('',#80522,#10341);
#8502=LINE('',#80526,#10342);
#8503=LINE('',#80530,#10343);
#8504=LINE('',#80536,#10344);
#8505=LINE('',#80539,#10345);
#8506=LINE('',#80552,#10346);
#8507=LINE('',#80558,#10347);
#8508=LINE('',#80561,#10348);
#8509=LINE('',#80568,#10349);
#8510=LINE('',#80570,#10350);
#8511=LINE('',#80571,#10351);
#8512=LINE('',#80583,#10352);
#8513=LINE('',#80594,#10353);
#8514=LINE('',#80603,#10354);
#8515=LINE('',#80617,#10355);
#8516=LINE('',#80627,#10356);
#8517=LINE('',#80635,#10357);
#8518=LINE('',#80649,#10358);
#8519=LINE('',#80657,#10359);
#8520=LINE('',#80665,#10360);
#8521=LINE('',#80673,#10361);
#8522=LINE('',#80681,#10362);
#8523=LINE('',#80687,#10363);
#8524=LINE('',#80693,#10364);
#8525=LINE('',#80701,#10365);
#8526=LINE('',#80707,#10366);
#8527=LINE('',#80713,#10367);
#8528=LINE('',#80719,#10368);
#8529=LINE('',#80735,#10369);
#8530=LINE('',#80736,#10370);
#8531=LINE('',#80745,#10371);
#8532=LINE('',#80748,#10372);
#8533=LINE('',#80761,#10373);
#8534=LINE('',#80762,#10374);
#8535=LINE('',#80780,#10375);
#8536=LINE('',#80783,#10376);
#8537=LINE('',#80789,#10377);
#8538=LINE('',#80878,#10378);
#8539=LINE('',#80885,#10379);
#8540=LINE('',#80888,#10380);
#8541=LINE('',#80890,#10381);
#8542=LINE('',#80891,#10382);
#8543=LINE('',#80894,#10383);
#8544=LINE('',#80904,#10384);
#8545=LINE('',#80905,#10385);
#8546=LINE('',#80906,#10386);
#8547=LINE('',#81242,#10387);
#8548=LINE('',#81380,#10388);
#8549=LINE('',#81382,#10389);
#8550=LINE('',#81522,#10390);
#8551=LINE('',#81649,#10391);
#8552=LINE('',#81653,#10392);
#8553=LINE('',#81654,#10393);
#8554=LINE('',#81657,#10394);
#8555=LINE('',#81661,#10395);
#8556=LINE('',#81662,#10396);
#8557=LINE('',#81665,#10397);
#8558=LINE('',#81669,#10398);
#8559=LINE('',#81670,#10399);
#8560=LINE('',#81673,#10400);
#8561=LINE('',#81677,#10401);
#8562=LINE('',#81678,#10402);
#8563=LINE('',#81681,#10403);
#8564=LINE('',#81685,#10404);
#8565=LINE('',#81686,#10405);
#8566=LINE('',#81691,#10406);
#8567=LINE('',#81693,#10407);
#8568=LINE('',#81694,#10408);
#8569=LINE('',#81699,#10409);
#8570=LINE('',#81701,#10410);
#8571=LINE('',#81702,#10411);
#8572=LINE('',#81705,#10412);
#8573=LINE('',#81709,#10413);
#8574=LINE('',#81710,#10414);
#8575=LINE('',#81715,#10415);
#8576=LINE('',#81717,#10416);
#8577=LINE('',#81718,#10417);
#8578=LINE('',#81723,#10418);
#8579=LINE('',#81725,#10419);
#8580=LINE('',#81726,#10420);
#8581=LINE('',#81729,#10421);
#8582=LINE('',#81732,#10422);
#8583=LINE('',#81736,#10423);
#8584=LINE('',#81813,#10424);
#8585=LINE('',#81822,#10425);
#8586=LINE('',#81826,#10426);
#8587=LINE('',#81834,#10427);
#8588=LINE('',#81838,#10428);
#8589=LINE('',#81890,#10429);
#8590=LINE('',#82018,#10430);
#8591=LINE('',#82026,#10431);
#8592=LINE('',#82038,#10432);
#8593=LINE('',#82046,#10433);
#8594=LINE('',#82054,#10434);
#8595=LINE('',#82062,#10435);
#8596=LINE('',#82070,#10436);
#8597=LINE('',#82076,#10437);
#8598=LINE('',#82083,#10438);
#8599=LINE('',#82092,#10439);
#8600=LINE('',#82098,#10440);
#8601=LINE('',#82105,#10441);
#8602=LINE('',#82112,#10442);
#8603=LINE('',#82122,#10443);
#8604=LINE('',#82128,#10444);
#8605=LINE('',#82129,#10445);
#8606=LINE('',#82138,#10446);
#8607=LINE('',#82151,#10447);
#8608=LINE('',#82161,#10448);
#8609=LINE('',#82201,#10449);
#8610=LINE('',#82212,#10450);
#8611=LINE('',#82213,#10451);
#8612=LINE('',#82229,#10452);
#8613=LINE('',#82232,#10453);
#8614=LINE('',#82242,#10454);
#8615=LINE('',#82244,#10455);
#8616=LINE('',#82254,#10456);
#8617=LINE('',#82256,#10457);
#8618=LINE('',#82261,#10458);
#8619=LINE('',#82262,#10459);
#8620=LINE('',#82268,#10460);
#8621=LINE('',#82285,#10461);
#8622=LINE('',#82288,#10462);
#8623=LINE('',#82307,#10463);
#8624=LINE('',#82308,#10464);
#8625=LINE('',#82438,#10465);
#8626=LINE('',#82441,#10466);
#8627=LINE('',#82444,#10467);
#8628=LINE('',#82456,#10468);
#8629=LINE('',#82458,#10469);
#8630=LINE('',#82464,#10470);
#8631=LINE('',#82467,#10471);
#8632=LINE('',#82471,#10472);
#8633=LINE('',#82475,#10473);
#8634=LINE('',#82479,#10474);
#8635=LINE('',#82539,#10475);
#8636=LINE('',#82541,#10476);
#8637=LINE('',#82543,#10477);
#8638=LINE('',#82546,#10478);
#8639=LINE('',#82615,#10479);
#8640=LINE('',#82616,#10480);
#8641=LINE('',#82625,#10481);
#8642=LINE('',#82633,#10482);
#8643=LINE('',#82641,#10483);
#8644=LINE('',#82647,#10484);
#8645=LINE('',#82665,#10485);
#8646=LINE('',#82667,#10486);
#8647=LINE('',#82669,#10487);
#8648=LINE('',#82708,#10488);
#8649=LINE('',#82710,#10489);
#8650=LINE('',#82712,#10490);
#8651=LINE('',#82714,#10491);
#8652=LINE('',#82732,#10492);
#8653=LINE('',#82915,#10493);
#8654=LINE('',#82918,#10494);
#8655=LINE('',#82922,#10495);
#8656=LINE('',#82926,#10496);
#8657=LINE('',#83279,#10497);
#10286=VECTOR('',#42369,1000.);
#10287=VECTOR('',#42374,1000.);
#10288=VECTOR('',#42377,1000.);
#10289=VECTOR('',#42384,1000.);
#10290=VECTOR('',#42443,0.730765926094);
#10291=VECTOR('',#42450,1000.);
#10292=VECTOR('',#42453,1000.);
#10293=VECTOR('',#42456,1000.);
#10294=VECTOR('',#42459,1000.);
#10295=VECTOR('',#42464,1000.);
#10296=VECTOR('',#42477,1000.);
#10297=VECTOR('',#42486,1000.);
#10298=VECTOR('',#42495,1000.);
#10299=VECTOR('',#42506,1000.);
#10300=VECTOR('',#42507,1000.);
#10301=VECTOR('',#42508,1000.);
#10302=VECTOR('',#42513,1000.);
#10303=VECTOR('',#42518,1000.);
#10304=VECTOR('',#42519,1000.);
#10305=VECTOR('',#42524,1000.);
#10306=VECTOR('',#42527,1000.);
#10307=VECTOR('',#42528,1000.);
#10308=VECTOR('',#42533,1000.);
#10309=VECTOR('',#42538,1000.);
#10310=VECTOR('',#42539,1000.);
#10311=VECTOR('',#42540,1000.);
#10312=VECTOR('',#42541,1000.);
#10313=VECTOR('',#42552,1000.);
#10314=VECTOR('',#42553,1000.);
#10315=VECTOR('',#42560,1000.);
#10316=VECTOR('',#42567,1000.);
#10317=VECTOR('',#42578,1000.);
#10318=VECTOR('',#42589,1000.);
#10319=VECTOR('',#42602,1000.);
#10320=VECTOR('',#42605,1000.);
#10321=VECTOR('',#42616,1000.);
#10322=VECTOR('',#42621,1000.);
#10323=VECTOR('',#42624,1000.);
#10324=VECTOR('',#42625,1000.);
#10325=VECTOR('',#42626,1000.);
#10326=VECTOR('',#42627,1000.);
#10327=VECTOR('',#42632,1000.);
#10328=VECTOR('',#42655,1000.);
#10329=VECTOR('',#42658,1000.);
#10330=VECTOR('',#42659,1000.);
#10331=VECTOR('',#42660,1000.);
#10332=VECTOR('',#42663,1000.);
#10333=VECTOR('',#42664,1000.);
#10334=VECTOR('',#42665,1000.);
#10335=VECTOR('',#42668,1000.);
#10336=VECTOR('',#42671,1000.);
#10337=VECTOR('',#42674,1000.);
#10338=VECTOR('',#42677,1000.);
#10339=VECTOR('',#42682,1000.);
#10340=VECTOR('',#42685,1000.);
#10341=VECTOR('',#42688,1000.);
#10342=VECTOR('',#42691,1000.);
#10343=VECTOR('',#42694,1000.);
#10344=VECTOR('',#42699,1000.);
#10345=VECTOR('',#42702,1000.);
#10346=VECTOR('',#42719,1000.);
#10347=VECTOR('',#42726,1000.);
#10348=VECTOR('',#42729,1000.);
#10349=VECTOR('',#42738,1000.);
#10350=VECTOR('',#42739,1000.);
#10351=VECTOR('',#42740,1000.);
#10352=VECTOR('',#42759,1000.);
#10353=VECTOR('',#42776,1000.);
#10354=VECTOR('',#42789,1000.);
#10355=VECTOR('',#42808,1000.);
#10356=VECTOR('',#42825,1000.);
#10357=VECTOR('',#42836,1000.);
#10358=VECTOR('',#42855,1000.);
#10359=VECTOR('',#42866,1000.);
#10360=VECTOR('',#42877,1000.);
#10361=VECTOR('',#42888,1000.);
#10362=VECTOR('',#42899,1000.);
#10363=VECTOR('',#42906,1000.);
#10364=VECTOR('',#42913,1000.);
#10365=VECTOR('',#42924,1000.);
#10366=VECTOR('',#42931,1000.);
#10367=VECTOR('',#42938,1000.);
#10368=VECTOR('',#42947,1000.);
#10369=VECTOR('',#42970,1000.);
#10370=VECTOR('',#42971,1000.);
#10371=VECTOR('',#42982,1000.);
#10372=VECTOR('',#42985,1000.);
#10373=VECTOR('',#42994,1000.);
#10374=VECTOR('',#42995,1000.);
#10375=VECTOR('',#43004,1000.);
#10376=VECTOR('',#43007,1000.);
#10377=VECTOR('',#43016,1000.);
#10378=VECTOR('',#43031,1000.);
#10379=VECTOR('',#43042,1000.);
#10380=VECTOR('',#43045,1000.);
#10381=VECTOR('',#43046,1000.);
#10382=VECTOR('',#43047,1000.);
#10383=VECTOR('',#43050,1000.);
#10384=VECTOR('',#43063,1000.);
#10385=VECTOR('',#43064,1000.);
#10386=VECTOR('',#43065,1000.);
#10387=VECTOR('',#43078,1000.);
#10388=VECTOR('',#43081,1000.);
#10389=VECTOR('',#43084,1000.);
#10390=VECTOR('',#43091,1000.);
#10391=VECTOR('',#43094,1000.);
#10392=VECTOR('',#43099,1000.);
#10393=VECTOR('',#43100,1000.);
#10394=VECTOR('',#43103,1000.);
#10395=VECTOR('',#43108,1000.);
#10396=VECTOR('',#43109,1000.);
#10397=VECTOR('',#43112,1000.);
#10398=VECTOR('',#43117,1000.);
#10399=VECTOR('',#43118,1000.);
#10400=VECTOR('',#43121,1000.);
#10401=VECTOR('',#43126,1000.);
#10402=VECTOR('',#43127,1000.);
#10403=VECTOR('',#43130,1000.);
#10404=VECTOR('',#43135,1000.);
#10405=VECTOR('',#43136,1000.);
#10406=VECTOR('',#43143,1000.);
#10407=VECTOR('',#43144,1000.);
#10408=VECTOR('',#43145,1000.);
#10409=VECTOR('',#43152,1000.);
#10410=VECTOR('',#43153,1000.);
#10411=VECTOR('',#43154,1000.);
#10412=VECTOR('',#43157,1000.);
#10413=VECTOR('',#43162,1000.);
#10414=VECTOR('',#43163,1000.);
#10415=VECTOR('',#43170,1000.);
#10416=VECTOR('',#43171,1000.);
#10417=VECTOR('',#43172,1000.);
#10418=VECTOR('',#43179,1000.);
#10419=VECTOR('',#43180,1000.);
#10420=VECTOR('',#43181,1000.);
#10421=VECTOR('',#43184,1000.);
#10422=VECTOR('',#43189,1000.);
#10423=VECTOR('',#43194,2.65);
#10424=VECTOR('',#43207,1000.);
#10425=VECTOR('',#43218,1000.);
#10426=VECTOR('',#43221,1000.);
#10427=VECTOR('',#43228,1000.);
#10428=VECTOR('',#43231,1000.);
#10429=VECTOR('',#43238,1000.);
#10430=VECTOR('',#43259,1000.);
#10431=VECTOR('',#43270,1000.);
#10432=VECTOR('',#43287,1000.);
#10433=VECTOR('',#43298,1000.);
#10434=VECTOR('',#43309,1000.);
#10435=VECTOR('',#43320,1000.);
#10436=VECTOR('',#43331,1000.);
#10437=VECTOR('',#43340,1000.);
#10438=VECTOR('',#43351,1000.);
#10439=VECTOR('',#43364,1000.);
#10440=VECTOR('',#43373,1000.);
#10441=VECTOR('',#43384,1000.);
#10442=VECTOR('',#43395,1000.);
#10443=VECTOR('',#43408,0.781285626506968);
#10444=VECTOR('',#43415,1000.);
#10445=VECTOR('',#43416,1000.);
#10446=VECTOR('',#43427,1000.);
#10447=VECTOR('',#43446,1000.);
#10448=VECTOR('',#43461,1000.);
#10449=VECTOR('',#43474,1000.);
#10450=VECTOR('',#43489,1000.);
#10451=VECTOR('',#43490,1000.);
#10452=VECTOR('',#43513,1.4);
#10453=VECTOR('',#43516,1000.);
#10454=VECTOR('',#43529,1000.);
#10455=VECTOR('',#43530,1000.);
#10456=VECTOR('',#43543,1000.);
#10457=VECTOR('',#43544,1000.);
#10458=VECTOR('',#43553,1000.);
#10459=VECTOR('',#43554,1000.);
#10460=VECTOR('',#43563,1000.);
#10461=VECTOR('',#43584,1000.);
#10462=VECTOR('',#43587,1000.);
#10463=VECTOR('',#43598,1000.);
#10464=VECTOR('',#43599,1000.);
#10465=VECTOR('',#43604,2.65);
#10466=VECTOR('',#43607,1000.);
#10467=VECTOR('',#43610,1000.);
#10468=VECTOR('',#43623,1000.);
#10469=VECTOR('',#43624,1000.);
#10470=VECTOR('',#43631,1000.);
#10471=VECTOR('',#43634,1000.);
#10472=VECTOR('',#43637,1000.);
#10473=VECTOR('',#43640,1000.);
#10474=VECTOR('',#43643,1000.);
#10475=VECTOR('',#43664,1000.);
#10476=VECTOR('',#43667,1000.);
#10477=VECTOR('',#43670,1000.);
#10478=VECTOR('',#43673,1000.);
#10479=VECTOR('',#43674,1000.);
#10480=VECTOR('',#43675,1000.);
#10481=VECTOR('',#43688,1000.);
#10482=VECTOR('',#43699,1000.);
#10483=VECTOR('',#43710,1000.);
#10484=VECTOR('',#43719,1000.);
#10485=VECTOR('',#43720,1000.);
#10486=VECTOR('',#43723,1000.);
#10487=VECTOR('',#43724,1000.);
#10488=VECTOR('',#43727,1000.);
#10489=VECTOR('',#43730,1000.);
#10490=VECTOR('',#43733,1000.);
#10491=VECTOR('',#43736,1000.);
#10492=VECTOR('',#43749,1000.);
#10493=VECTOR('',#43758,1000.);
#10494=VECTOR('',#43761,1000.);
#10495=VECTOR('',#43766,1000.);
#10496=VECTOR('',#43771,1000.);
#10497=VECTOR('',#43792,1000.);
#12037=CIRCLE('',#35729,3.98587879194);
#12038=CIRCLE('',#35731,4.25458972003406);
#12039=CIRCLE('',#35734,0.299547728742047);
#12040=CIRCLE('',#35735,4.12347080401);
#12041=CIRCLE('',#35736,0.3);
#12042=CIRCLE('',#35737,0.3);
#12043=CIRCLE('',#35738,4.40314384042832);
#12044=CIRCLE('',#35740,0.300000000000001);
#12045=CIRCLE('',#35741,0.300000000000001);
#12046=CIRCLE('',#35742,4.72461821943);
#12047=CIRCLE('',#35743,0.300000000000001);
#12048=CIRCLE('',#35744,0.300000000000001);
#12049=CIRCLE('',#35745,4.42622127925);
#12050=CIRCLE('',#35747,0.300126293190847);
#12051=CIRCLE('',#35748,4.40312534809379);
#12052=CIRCLE('',#35749,0.299998398909284);
#12053=CIRCLE('',#35750,0.299965609274366);
#12054=CIRCLE('',#35751,4.12347080401);
#12055=CIRCLE('',#35754,4.25458975164979);
#12056=CIRCLE('',#35756,3.98587879194);
#12057=CIRCLE('',#35758,4.1423251838);
#12058=CIRCLE('',#35759,4.44177037781);
#12059=CIRCLE('',#35760,0.300000000000024);
#12060=CIRCLE('',#35762,3.93623398426);
#12061=CIRCLE('',#35765,4.00032353732);
#12062=CIRCLE('',#35766,4.00032353732);
#12063=CIRCLE('',#35770,0.3);
#12064=CIRCLE('',#35771,0.3);
#12065=CIRCLE('',#35773,0.299999999999949);
#12066=CIRCLE('',#35774,4.28950984611483);
#12067=CIRCLE('',#35776,4.28950741312049);
#12068=CIRCLE('',#35777,4.45);
#12069=CIRCLE('',#35778,4.22078101927);
#12070=CIRCLE('',#35779,4.17921044955);
#12071=CIRCLE('',#35780,2.48263157895);
#12072=CIRCLE('',#35781,3.8935342738);
#12073=CIRCLE('',#35782,3.73004103777);
#12074=CIRCLE('',#35783,2.48263157895);
#12075=CIRCLE('',#35784,2.48263157895);
#12076=CIRCLE('',#35785,3.73004103777);
#12077=CIRCLE('',#35786,3.8935342738);
#12078=CIRCLE('',#35787,2.48263157895);
#12079=CIRCLE('',#35789,0.3);
#12080=CIRCLE('',#35790,0.3);
#12081=CIRCLE('',#35792,0.300000000000001);
#12082=CIRCLE('',#35795,0.730765926094);
#12083=CIRCLE('',#35797,0.730765926094);
#12084=CIRCLE('',#35799,4.45);
#12085=CIRCLE('',#35800,0.2);
#12086=CIRCLE('',#35801,0.2);
#12087=CIRCLE('',#35802,1.3);
#12088=CIRCLE('',#35804,0.3);
#12089=CIRCLE('',#35807,0.3);
#12090=CIRCLE('',#35808,1.);
#12091=CIRCLE('',#35810,0.3);
#12092=CIRCLE('',#35811,0.3);
#12093=CIRCLE('',#35812,0.5);
#12094=CIRCLE('',#35814,0.3);
#12095=CIRCLE('',#35815,0.3);
#12096=CIRCLE('',#35816,0.5);
#12097=CIRCLE('',#35818,0.3);
#12098=CIRCLE('',#35820,0.3);
#12099=CIRCLE('',#35821,4.15);
#12100=CIRCLE('',#35822,0.3);
#12101=CIRCLE('',#35826,1.);
#12102=CIRCLE('',#35829,0.5);
#12103=CIRCLE('',#35832,0.5);
#12104=CIRCLE('',#35837,0.5);
#12105=CIRCLE('',#35839,4.15);
#12106=CIRCLE('',#35840,0.5);
#12107=CIRCLE('',#35842,0.1);
#12108=CIRCLE('',#35843,0.1);
#12109=CIRCLE('',#35845,1.);
#12110=CIRCLE('',#35847,0.1);
#12111=CIRCLE('',#35848,0.9);
#12112=CIRCLE('',#35850,0.1);
#12113=CIRCLE('',#35852,0.1);
#12114=CIRCLE('',#35853,0.6);
#12115=CIRCLE('',#35855,0.1);
#12116=CIRCLE('',#35857,0.1);
#12117=CIRCLE('',#35858,0.6);
#12118=CIRCLE('',#35859,0.300088662990782);
#12119=CIRCLE('',#35861,0.3);
#12120=CIRCLE('',#35863,0.3);
#12121=CIRCLE('',#35864,0.3);
#12122=CIRCLE('',#35866,0.999999999999999);
#12123=CIRCLE('',#35867,0.999999999999999);
#12124=CIRCLE('',#35869,0.1);
#12125=CIRCLE('',#35871,0.300088662500368);
#12126=CIRCLE('',#35873,0.5);
#12127=CIRCLE('',#35875,3.85);
#12128=CIRCLE('',#35876,0.3);
#12129=CIRCLE('',#35877,0.3);
#12130=CIRCLE('',#35879,0.5);
#12131=CIRCLE('',#35881,1.1);
#12132=CIRCLE('',#35882,0.1);
#12133=CIRCLE('',#35884,0.2);
#12134=CIRCLE('',#35885,0.2);
#12135=CIRCLE('',#35886,0.6);
#12136=CIRCLE('',#35887,0.6);
#12137=CIRCLE('',#35888,0.4);
#12138=CIRCLE('',#35889,0.9);
#12139=CIRCLE('',#35890,0.199999999999999);
#12140=CIRCLE('',#35891,3.05);
#12141=CIRCLE('',#35892,0.400000000000001);
#12142=CIRCLE('',#35893,1.1);
#12143=CIRCLE('',#35894,1.1);
#12144=CIRCLE('',#35895,0.400000000000001);
#12145=CIRCLE('',#35896,3.05);
#12146=CIRCLE('',#35897,0.199999999999999);
#12147=CIRCLE('',#35898,0.9);
#12148=CIRCLE('',#35900,0.3);
#12149=CIRCLE('',#35902,0.3);
#12150=CIRCLE('',#35903,4.15601973046);
#12151=CIRCLE('',#35904,0.3);
#12152=CIRCLE('',#35906,0.799999999999999);
#12153=CIRCLE('',#35907,0.699999999999999);
#12154=CIRCLE('',#35908,0.8);
#12155=CIRCLE('',#35909,0.8);
#12156=CIRCLE('',#35910,0.699999999999999);
#12157=CIRCLE('',#35911,2.95);
#12158=CIRCLE('',#35913,0.3);
#12159=CIRCLE('',#35916,0.1);
#12160=CIRCLE('',#35918,0.3);
#12161=CIRCLE('',#35919,0.3);
#12162=CIRCLE('',#35921,0.3);
#12163=CIRCLE('',#35923,1.);
#12164=CIRCLE('',#35924,1.);
#12165=CIRCLE('',#35926,0.1);
#12166=CIRCLE('',#35928,0.3);
#12167=CIRCLE('',#35931,0.1);
#12168=CIRCLE('',#35934,0.1);
#12169=CIRCLE('',#35935,1.);
#12170=CIRCLE('',#35937,0.1);
#12171=CIRCLE('',#35939,0.1);
#12172=CIRCLE('',#35940,0.300000000000002);
#12173=CIRCLE('',#35942,0.1);
#12174=CIRCLE('',#35943,2.95);
#12175=CIRCLE('',#35945,0.1);
#12176=CIRCLE('',#35946,0.1);
#12177=CIRCLE('',#35948,0.1);
#12178=CIRCLE('',#35949,0.5);
#12179=CIRCLE('',#35952,0.1);
#12180=CIRCLE('',#35954,0.1);
#12181=CIRCLE('',#35956,0.1);
#12182=CIRCLE('',#35957,0.5);
#12183=CIRCLE('',#35959,0.1);
#12184=CIRCLE('',#35961,0.1);
#12185=CIRCLE('',#35962,0.1);
#12186=CIRCLE('',#35963,2.95);
#12187=CIRCLE('',#35965,0.1);
#12188=CIRCLE('',#35966,0.300000000000002);
#12189=CIRCLE('',#35968,0.1);
#12190=CIRCLE('',#35970,0.1);
#12191=CIRCLE('',#35971,1.);
#12192=CIRCLE('',#35973,0.1);
#12193=CIRCLE('',#35975,0.1);
#12194=CIRCLE('',#35976,0.5);
#12195=CIRCLE('',#35978,0.1);
#12196=CIRCLE('',#35980,0.1);
#12197=CIRCLE('',#35981,0.5);
#12198=CIRCLE('',#35983,0.1);
#12199=CIRCLE('',#35985,0.1);
#12200=CIRCLE('',#35986,0.5);
#12201=CIRCLE('',#35988,0.1);
#12202=CIRCLE('',#35990,0.1);
#12203=CIRCLE('',#35991,0.1);
#12204=CIRCLE('',#35993,0.1);
#12205=CIRCLE('',#35994,0.1);
#12206=CIRCLE('',#35996,0.1);
#12207=CIRCLE('',#35997,0.1);
#12208=CIRCLE('',#35999,0.1);
#12209=CIRCLE('',#36001,0.1);
#12210=CIRCLE('',#36002,0.1);
#12211=CIRCLE('',#36004,0.1);
#12212=CIRCLE('',#36005,0.1);
#12213=CIRCLE('',#36007,0.1);
#12214=CIRCLE('',#36008,0.1);
#12215=CIRCLE('',#36011,2.65);
#12216=CIRCLE('',#36012,2.65);
#12217=CIRCLE('',#36013,0.3);
#12218=CIRCLE('',#36015,0.3);
#12219=CIRCLE('',#36017,0.300000000000001);
#12220=CIRCLE('',#36018,2.95);
#12221=CIRCLE('',#36019,0.300000018904248);
#12222=CIRCLE('',#36022,0.299999999999999);
#12223=CIRCLE('',#36023,2.95);
#12224=CIRCLE('',#36024,0.300000075511691);
#12225=CIRCLE('',#36026,2.95);
#12226=CIRCLE('',#36028,0.3);
#12227=CIRCLE('',#36029,2.95);
#12228=CIRCLE('',#36032,2.95);
#12229=CIRCLE('',#36033,0.300000017917961);
#12230=CIRCLE('',#36035,2.95);
#12231=CIRCLE('',#36037,0.3);
#12232=CIRCLE('',#36038,0.300000000000001);
#12233=CIRCLE('',#36041,0.3);
#12234=CIRCLE('',#36043,0.5);
#12235=CIRCLE('',#36044,0.3);
#12236=CIRCLE('',#36049,3.98150447852);
#12237=CIRCLE('',#36050,0.299999999999992);
#12238=CIRCLE('',#36054,1.);
#12239=CIRCLE('',#36056,0.300000000004292);
#12240=CIRCLE('',#36057,4.46095497423);
#12241=CIRCLE('',#36058,0.299999910435179);
#12242=CIRCLE('',#36061,0.300000000000002);
#12243=CIRCLE('',#36064,0.0999999999999994);
#12244=CIRCLE('',#36069,0.0999999999999994);
#12245=CIRCLE('',#36072,0.300000000000002);
#12246=CIRCLE('',#36075,1.);
#12247=CIRCLE('',#36078,0.5);
#12248=CIRCLE('',#36081,0.5);
#12249=CIRCLE('',#36084,0.5);
#12250=CIRCLE('',#36087,0.1);
#12251=CIRCLE('',#36090,0.1);
#12252=CIRCLE('',#36093,0.1);
#12253=CIRCLE('',#36096,0.0999999999999994);
#12254=CIRCLE('',#36099,0.0999999999999994);
#12255=CIRCLE('',#36102,0.1);
#12256=CIRCLE('',#36105,2.65);
#12257=CIRCLE('',#36107,0.1);
#12258=CIRCLE('',#36108,3.05);
#12259=CIRCLE('',#36109,0.1);
#12260=CIRCLE('',#36111,0.0999999999999994);
#12261=CIRCLE('',#36113,0.3);
#12262=CIRCLE('',#36114,4.15601973046);
#12263=CIRCLE('',#36115,0.3);
#12264=CIRCLE('',#36117,0.699999999999999);
#12265=CIRCLE('',#36118,0.8);
#12266=CIRCLE('',#36119,3.85);
#12267=CIRCLE('',#36120,0.8);
#12268=CIRCLE('',#36121,0.699999999999999);
#12269=CIRCLE('',#36122,0.799999999999999);
#12270=CIRCLE('',#36123,2.95);
#12271=CIRCLE('',#36125,0.0999999999999994);
#12272=CIRCLE('',#36127,0.3);
#12273=CIRCLE('',#36128,0.3);
#12274=CIRCLE('',#36129,0.3);
#12275=CIRCLE('',#36134,0.1);
#12276=CIRCLE('',#36136,0.1);
#12277=CIRCLE('',#36137,0.9);
#12278=CIRCLE('',#36139,0.1);
#12279=CIRCLE('',#36141,0.1);
#12280=CIRCLE('',#36142,0.199999999999999);
#12281=CIRCLE('',#36144,0.1);
#12282=CIRCLE('',#36145,0.199999999999999);
#12283=CIRCLE('',#36147,0.1);
#12284=CIRCLE('',#36149,0.1);
#12285=CIRCLE('',#36150,0.9);
#12286=CIRCLE('',#36152,0.1);
#12287=CIRCLE('',#36154,0.1);
#12288=CIRCLE('',#36155,0.4);
#12289=CIRCLE('',#36157,0.1);
#12290=CIRCLE('',#36159,0.1);
#12291=CIRCLE('',#36160,0.6);
#12292=CIRCLE('',#36162,0.1);
#12293=CIRCLE('',#36164,0.1);
#12294=CIRCLE('',#36165,0.6);
#12295=CIRCLE('',#36167,0.1);
#12296=CIRCLE('',#36169,0.1);
#12297=CIRCLE('',#36171,0.1);
#12298=CIRCLE('',#36172,0.1);
#12299=CIRCLE('',#36174,0.1);
#12300=CIRCLE('',#36176,0.1);
#12301=CIRCLE('',#36177,0.1);
#12302=CIRCLE('',#36179,0.1);
#12303=CIRCLE('',#36180,0.2);
#12304=CIRCLE('',#36182,0.1);
#12305=CIRCLE('',#36184,0.0999999999999994);
#12306=CIRCLE('',#36186,0.1);
#12307=CIRCLE('',#36187,0.1);
#12308=CIRCLE('',#36189,0.0999999999999994);
#12309=CIRCLE('',#36191,0.1);
#12310=CIRCLE('',#36192,0.1);
#12311=CIRCLE('',#36194,0.1);
#12312=CIRCLE('',#36195,0.2);
#12313=CIRCLE('',#36198,1.4);
#12314=CIRCLE('',#36200,0.1);
#12315=CIRCLE('',#36202,2.62880107536);
#12316=CIRCLE('',#36203,2.44564212855);
#12317=CIRCLE('',#36204,2.44564212855);
#12318=CIRCLE('',#36207,2.65);
#12319=CIRCLE('',#36208,0.3);
#12320=CIRCLE('',#36210,0.3);
#12321=CIRCLE('',#36211,0.3);
#12322=CIRCLE('',#36213,0.3);
#12323=CIRCLE('',#36214,1.);
#12324=CIRCLE('',#36216,0.3);
#12325=CIRCLE('',#36217,0.999999999999999);
#12326=CIRCLE('',#36218,0.3);
#12327=CIRCLE('',#36221,0.3);
#12328=CIRCLE('',#36222,0.5);
#12329=CIRCLE('',#36224,0.300000000000001);
#12330=CIRCLE('',#36225,0.3);
#12331=CIRCLE('',#36228,0.3);
#12332=CIRCLE('',#36230,0.3);
#12333=CIRCLE('',#36231,0.5);
#12334=CIRCLE('',#36234,0.3);
#12335=CIRCLE('',#36235,0.5);
#12336=CIRCLE('',#36236,0.3);
#12337=CIRCLE('',#36238,4.15);
#12338=CIRCLE('',#36241,0.1);
#12339=CIRCLE('',#36242,2.36684105317747);
#12340=CIRCLE('',#36243,2.36684105317747);
#12341=CIRCLE('',#36244,2.36684105317747);
#12342=CIRCLE('',#36250,1.4);
#12343=CIRCLE('',#36252,0.1);
#12344=CIRCLE('',#36254,0.5);
#12345=CIRCLE('',#36255,0.400000000000001);
#12346=CIRCLE('',#36256,0.1);
#12347=CIRCLE('',#36258,0.1);
#12348=CIRCLE('',#36260,1.);
#12349=CIRCLE('',#36261,1.1);
#12350=CIRCLE('',#36262,0.1);
#12351=CIRCLE('',#36264,0.1);
#12352=CIRCLE('',#36266,0.3);
#12353=CIRCLE('',#36269,0.300045031714467);
#12354=CIRCLE('',#36270,3.98150447852);
#12355=CIRCLE('',#36273,0.1);
#12356=CIRCLE('',#36274,2.65);
#12357=CIRCLE('',#36277,0.3);
#12358=CIRCLE('',#36278,1.);
#12359=CIRCLE('',#36279,0.3);
#12360=CIRCLE('',#36280,1.3);
#12361=CIRCLE('',#36282,0.299999999999998);
#12362=CIRCLE('',#36283,0.3);
#12363=CIRCLE('',#36284,0.5);
#12364=CIRCLE('',#36285,0.3);
#12365=CIRCLE('',#36286,0.2);
#12366=CIRCLE('',#36291,0.3);
#12367=CIRCLE('',#36293,0.999999999999999);
#12368=CIRCLE('',#36294,0.1);
#12369=CIRCLE('',#36295,1.1);
#12370=CIRCLE('',#36296,0.1);
#12371=CIRCLE('',#36298,0.1);
#12372=CIRCLE('',#36300,3.05);
#12373=CIRCLE('',#36301,0.400000000000001);
#12374=CIRCLE('',#36302,0.6);
#12375=CIRCLE('',#36303,0.6);
#12376=CIRCLE('',#36304,0.9);
#12377=CIRCLE('',#36305,1.1);
#12378=CIRCLE('',#36307,0.1);
#12379=CIRCLE('',#36309,0.1);
#12380=CIRCLE('',#36311,0.1);
#12381=CIRCLE('',#36313,0.5);
#12382=CIRCLE('',#36319,0.1);
#12383=CIRCLE('',#36321,0.5);
#12384=CIRCLE('',#36322,0.1);
#12385=CIRCLE('',#36324,0.1);
#12386=CIRCLE('',#36326,0.5);
#12387=CIRCLE('',#36327,0.1);
#12388=CIRCLE('',#36329,0.1);
#12389=CIRCLE('',#36331,1.);
#12390=CIRCLE('',#36332,0.1);
#12391=CIRCLE('',#36334,0.1);
#12392=CIRCLE('',#36336,1.);
#12393=CIRCLE('',#36344,0.5);
#12394=CIRCLE('',#36345,0.3);
#12395=CIRCLE('',#36346,0.2);
#12396=CIRCLE('',#36350,0.5);
#12397=CIRCLE('',#36351,0.3);
#12398=CIRCLE('',#36354,4.15);
#12399=CIRCLE('',#36356,0.5);
#12400=CIRCLE('',#36358,0.300088662981395);
#12401=CIRCLE('',#36362,0.3);
#12402=CIRCLE('',#36364,4.45);
#14926=VERTEX_POINT('',#78625);
#14927=VERTEX_POINT('',#78626);
#14928=VERTEX_POINT('',#78633);
#14929=VERTEX_POINT('',#78635);
#14930=VERTEX_POINT('',#78637);
#14931=VERTEX_POINT('',#78639);
#14932=VERTEX_POINT('',#78648);
#14933=VERTEX_POINT('',#78649);
#14934=VERTEX_POINT('',#78651);
#14935=VERTEX_POINT('',#78653);
#14936=VERTEX_POINT('',#78655);
#14937=VERTEX_POINT('',#78657);
#14938=VERTEX_POINT('',#78661);
#14939=VERTEX_POINT('',#78662);
#14940=VERTEX_POINT('',#78664);
#14941=VERTEX_POINT('',#78666);
#14942=VERTEX_POINT('',#78668);
#14943=VERTEX_POINT('',#78670);
#14944=VERTEX_POINT('',#78674);
#14945=VERTEX_POINT('',#78675);
#14946=VERTEX_POINT('',#78677);
#14947=VERTEX_POINT('',#78684);
#14948=VERTEX_POINT('',#78686);
#14949=VERTEX_POINT('',#78688);
#14950=VERTEX_POINT('',#78692);
#14951=VERTEX_POINT('',#78693);
#14952=VERTEX_POINT('',#78695);
#14953=VERTEX_POINT('',#78702);
#14954=VERTEX_POINT('',#78704);
#14955=VERTEX_POINT('',#78711);
#14956=VERTEX_POINT('',#78715);
#14957=VERTEX_POINT('',#78716);
#14958=VERTEX_POINT('',#78718);
#14959=VERTEX_POINT('',#78725);
#14960=VERTEX_POINT('',#78727);
#14961=VERTEX_POINT('',#78948);
#14962=VERTEX_POINT('',#78994);
#14963=VERTEX_POINT('',#78995);
#14964=VERTEX_POINT('',#78999);
#14965=VERTEX_POINT('',#79067);
#14966=VERTEX_POINT('',#79137);
#14967=VERTEX_POINT('',#79138);
#14968=VERTEX_POINT('',#79187);
#14969=VERTEX_POINT('',#79191);
#14970=VERTEX_POINT('',#79253);
#14971=VERTEX_POINT('',#79254);
#14972=VERTEX_POINT('',#79352);
#14973=VERTEX_POINT('',#79376);
#14974=VERTEX_POINT('',#79379);
#14975=VERTEX_POINT('',#79380);
#14976=VERTEX_POINT('',#79382);
#14977=VERTEX_POINT('',#79392);
#14978=VERTEX_POINT('',#79406);
#14979=VERTEX_POINT('',#79429);
#14980=VERTEX_POINT('',#79431);
#14981=VERTEX_POINT('',#79476);
#14982=VERTEX_POINT('',#79502);
#14983=VERTEX_POINT('',#79547);
#14984=VERTEX_POINT('',#79588);
#14985=VERTEX_POINT('',#79618);
#14986=VERTEX_POINT('',#79659);
#14987=VERTEX_POINT('',#79661);
#14988=VERTEX_POINT('',#79685);
#14989=VERTEX_POINT('',#79698);
#14990=VERTEX_POINT('',#79752);
#14991=VERTEX_POINT('',#79755);
#14992=VERTEX_POINT('',#79759);
#14993=VERTEX_POINT('',#79760);
#14994=VERTEX_POINT('',#79762);
#14995=VERTEX_POINT('',#79764);
#14996=VERTEX_POINT('',#79766);
#14997=VERTEX_POINT('',#79768);
#14998=VERTEX_POINT('',#79770);
#14999=VERTEX_POINT('',#79772);
#15000=VERTEX_POINT('',#79776);
#15001=VERTEX_POINT('',#79778);
#15002=VERTEX_POINT('',#79782);
#15003=VERTEX_POINT('',#79786);
#15004=VERTEX_POINT('',#79798);
#15005=VERTEX_POINT('',#79802);
#15006=VERTEX_POINT('',#79814);
#15007=VERTEX_POINT('',#79818);
#15008=VERTEX_POINT('',#79822);
#15009=VERTEX_POINT('',#79832);
#15010=VERTEX_POINT('',#79858);
#15011=VERTEX_POINT('',#79868);
#15012=VERTEX_POINT('',#79875);
#15013=VERTEX_POINT('',#79877);
#15014=VERTEX_POINT('',#79881);
#15015=VERTEX_POINT('',#79882);
#15016=VERTEX_POINT('',#79884);
#15017=VERTEX_POINT('',#79962);
#15018=VERTEX_POINT('',#79966);
#15019=VERTEX_POINT('',#79970);
#15020=VERTEX_POINT('',#79974);
#15021=VERTEX_POINT('',#79978);
#15022=VERTEX_POINT('',#80017);
#15023=VERTEX_POINT('',#80030);
#15024=VERTEX_POINT('',#80086);
#15025=VERTEX_POINT('',#80088);
#15026=VERTEX_POINT('',#80090);
#15027=VERTEX_POINT('',#80129);
#15028=VERTEX_POINT('',#80131);
#15029=VERTEX_POINT('',#80197);
#15030=VERTEX_POINT('',#80209);
#15031=VERTEX_POINT('',#80210);
#15032=VERTEX_POINT('',#80223);
#15033=VERTEX_POINT('',#80235);
#15034=VERTEX_POINT('',#80237);
#15035=VERTEX_POINT('',#80241);
#15036=VERTEX_POINT('',#80245);
#15037=VERTEX_POINT('',#80249);
#15038=VERTEX_POINT('',#80253);
#15039=VERTEX_POINT('',#80257);
#15040=VERTEX_POINT('',#80261);
#15041=VERTEX_POINT('',#80320);
#15042=VERTEX_POINT('',#80324);
#15043=VERTEX_POINT('',#80325);
#15044=VERTEX_POINT('',#80330);
#15045=VERTEX_POINT('',#80332);
#15046=VERTEX_POINT('',#80336);
#15047=VERTEX_POINT('',#80340);
#15048=VERTEX_POINT('',#80342);
#15049=VERTEX_POINT('',#80344);
#15050=VERTEX_POINT('',#80346);
#15051=VERTEX_POINT('',#80459);
#15052=VERTEX_POINT('',#80463);
#15053=VERTEX_POINT('',#80464);
#15054=VERTEX_POINT('',#80471);
#15055=VERTEX_POINT('',#80475);
#15056=VERTEX_POINT('',#80476);
#15057=VERTEX_POINT('',#80478);
#15058=VERTEX_POINT('',#80480);
#15059=VERTEX_POINT('',#80482);
#15060=VERTEX_POINT('',#80484);
#15061=VERTEX_POINT('',#80486);
#15062=VERTEX_POINT('',#80488);
#15063=VERTEX_POINT('',#80490);
#15064=VERTEX_POINT('',#80492);
#15065=VERTEX_POINT('',#80494);
#15066=VERTEX_POINT('',#80496);
#15067=VERTEX_POINT('',#80498);
#15068=VERTEX_POINT('',#80500);
#15069=VERTEX_POINT('',#80502);
#15070=VERTEX_POINT('',#80504);
#15071=VERTEX_POINT('',#80506);
#15072=VERTEX_POINT('',#80508);
#15073=VERTEX_POINT('',#80510);
#15074=VERTEX_POINT('',#80512);
#15075=VERTEX_POINT('',#80514);
#15076=VERTEX_POINT('',#80516);
#15077=VERTEX_POINT('',#80518);
#15078=VERTEX_POINT('',#80520);
#15079=VERTEX_POINT('',#80523);
#15080=VERTEX_POINT('',#80525);
#15081=VERTEX_POINT('',#80527);
#15082=VERTEX_POINT('',#80529);
#15083=VERTEX_POINT('',#80531);
#15084=VERTEX_POINT('',#80533);
#15085=VERTEX_POINT('',#80535);
#15086=VERTEX_POINT('',#80537);
#15087=VERTEX_POINT('',#80543);
#15088=VERTEX_POINT('',#80545);
#15089=VERTEX_POINT('',#80549);
#15090=VERTEX_POINT('',#80551);
#15091=VERTEX_POINT('',#80555);
#15092=VERTEX_POINT('',#80557);
#15093=VERTEX_POINT('',#80559);
#15094=VERTEX_POINT('',#80562);
#15095=VERTEX_POINT('',#80567);
#15096=VERTEX_POINT('',#80569);
#15097=VERTEX_POINT('',#80580);
#15098=VERTEX_POINT('',#80582);
#15099=VERTEX_POINT('',#80591);
#15100=VERTEX_POINT('',#80593);
#15101=VERTEX_POINT('',#80597);
#15102=VERTEX_POINT('',#80601);
#15103=VERTEX_POINT('',#80605);
#15104=VERTEX_POINT('',#80609);
#15105=VERTEX_POINT('',#80613);
#15106=VERTEX_POINT('',#80615);
#15107=VERTEX_POINT('',#80625);
#15108=VERTEX_POINT('',#80629);
#15109=VERTEX_POINT('',#80633);
#15110=VERTEX_POINT('',#80637);
#15111=VERTEX_POINT('',#80639);
#15112=VERTEX_POINT('',#80643);
#15113=VERTEX_POINT('',#80647);
#15114=VERTEX_POINT('',#80651);
#15115=VERTEX_POINT('',#80655);
#15116=VERTEX_POINT('',#80659);
#15117=VERTEX_POINT('',#80663);
#15118=VERTEX_POINT('',#80667);
#15119=VERTEX_POINT('',#80671);
#15120=VERTEX_POINT('',#80675);
#15121=VERTEX_POINT('',#80679);
#15122=VERTEX_POINT('',#80683);
#15123=VERTEX_POINT('',#80685);
#15124=VERTEX_POINT('',#80689);
#15125=VERTEX_POINT('',#80691);
#15126=VERTEX_POINT('',#80695);
#15127=VERTEX_POINT('',#80699);
#15128=VERTEX_POINT('',#80703);
#15129=VERTEX_POINT('',#80705);
#15130=VERTEX_POINT('',#80709);
#15131=VERTEX_POINT('',#80711);
#15132=VERTEX_POINT('',#80715);
#15133=VERTEX_POINT('',#80721);
#15134=VERTEX_POINT('',#80722);
#15135=VERTEX_POINT('',#80729);
#15136=VERTEX_POINT('',#80731);
#15137=VERTEX_POINT('',#80738);
#15138=VERTEX_POINT('',#80740);
#15139=VERTEX_POINT('',#80744);
#15140=VERTEX_POINT('',#80746);
#15141=VERTEX_POINT('',#80750);
#15142=VERTEX_POINT('',#80752);
#15143=VERTEX_POINT('',#80764);
#15144=VERTEX_POINT('',#80775);
#15145=VERTEX_POINT('',#80779);
#15146=VERTEX_POINT('',#80781);
#15147=VERTEX_POINT('',#80785);
#15148=VERTEX_POINT('',#80791);
#15149=VERTEX_POINT('',#80881);
#15150=VERTEX_POINT('',#80887);
#15151=VERTEX_POINT('',#80889);
#15152=VERTEX_POINT('',#80893);
#15153=VERTEX_POINT('',#80897);
#15154=VERTEX_POINT('',#80899);
#15155=VERTEX_POINT('',#80903);
#15156=VERTEX_POINT('',#81648);
#15157=VERTEX_POINT('',#81652);
#15158=VERTEX_POINT('',#81656);
#15159=VERTEX_POINT('',#81660);
#15160=VERTEX_POINT('',#81664);
#15161=VERTEX_POINT('',#81668);
#15162=VERTEX_POINT('',#81672);
#15163=VERTEX_POINT('',#81676);
#15164=VERTEX_POINT('',#81680);
#15165=VERTEX_POINT('',#81684);
#15166=VERTEX_POINT('',#81690);
#15167=VERTEX_POINT('',#81692);
#15168=VERTEX_POINT('',#81698);
#15169=VERTEX_POINT('',#81700);
#15170=VERTEX_POINT('',#81704);
#15171=VERTEX_POINT('',#81708);
#15172=VERTEX_POINT('',#81714);
#15173=VERTEX_POINT('',#81716);
#15174=VERTEX_POINT('',#81722);
#15175=VERTEX_POINT('',#81724);
#15176=VERTEX_POINT('',#81728);
#15177=VERTEX_POINT('',#81734);
#15178=VERTEX_POINT('',#81738);
#15179=VERTEX_POINT('',#81740);
#15180=VERTEX_POINT('',#81811);
#15181=VERTEX_POINT('',#81815);
#15182=VERTEX_POINT('',#81817);
#15183=VERTEX_POINT('',#81821);
#15184=VERTEX_POINT('',#81823);
#15185=VERTEX_POINT('',#81825);
#15186=VERTEX_POINT('',#81827);
#15187=VERTEX_POINT('',#81829);
#15188=VERTEX_POINT('',#81831);
#15189=VERTEX_POINT('',#81833);
#15190=VERTEX_POINT('',#81835);
#15191=VERTEX_POINT('',#81837);
#15192=VERTEX_POINT('',#81840);
#15193=VERTEX_POINT('',#81889);
#15194=VERTEX_POINT('',#81893);
#15195=VERTEX_POINT('',#81895);
#15196=VERTEX_POINT('',#82014);
#15197=VERTEX_POINT('',#82016);
#15198=VERTEX_POINT('',#82020);
#15199=VERTEX_POINT('',#82024);
#15200=VERTEX_POINT('',#82028);
#15201=VERTEX_POINT('',#82032);
#15202=VERTEX_POINT('',#82036);
#15203=VERTEX_POINT('',#82040);
#15204=VERTEX_POINT('',#82044);
#15205=VERTEX_POINT('',#82048);
#15206=VERTEX_POINT('',#82052);
#15207=VERTEX_POINT('',#82056);
#15208=VERTEX_POINT('',#82060);
#15209=VERTEX_POINT('',#82064);
#15210=VERTEX_POINT('',#82068);
#15211=VERTEX_POINT('',#82074);
#15212=VERTEX_POINT('',#82081);
#15213=VERTEX_POINT('',#82086);
#15214=VERTEX_POINT('',#82090);
#15215=VERTEX_POINT('',#82096);
#15216=VERTEX_POINT('',#82103);
#15217=VERTEX_POINT('',#82108);
#15218=VERTEX_POINT('',#82114);
#15219=VERTEX_POINT('',#82119);
#15220=VERTEX_POINT('',#82121);
#15221=VERTEX_POINT('',#82123);
#15222=VERTEX_POINT('',#82127);
#15223=VERTEX_POINT('',#82131);
#15224=VERTEX_POINT('',#82135);
#15225=VERTEX_POINT('',#82137);
#15226=VERTEX_POINT('',#82141);
#15227=VERTEX_POINT('',#82145);
#15228=VERTEX_POINT('',#82147);
#15229=VERTEX_POINT('',#82153);
#15230=VERTEX_POINT('',#82157);
#15231=VERTEX_POINT('',#82163);
#15232=VERTEX_POINT('',#82197);
#15233=VERTEX_POINT('',#82203);
#15234=VERTEX_POINT('',#82205);
#15235=VERTEX_POINT('',#82211);
#15236=VERTEX_POINT('',#82215);
#15237=VERTEX_POINT('',#82217);
#15238=VERTEX_POINT('',#82219);
#15239=VERTEX_POINT('',#82227);
#15240=VERTEX_POINT('',#82231);
#15241=VERTEX_POINT('',#82235);
#15242=VERTEX_POINT('',#82237);
#15243=VERTEX_POINT('',#82241);
#15244=VERTEX_POINT('',#82243);
#15245=VERTEX_POINT('',#82247);
#15246=VERTEX_POINT('',#82249);
#15247=VERTEX_POINT('',#82253);
#15248=VERTEX_POINT('',#82255);
#15249=VERTEX_POINT('',#82264);
#15250=VERTEX_POINT('',#82270);
#15251=VERTEX_POINT('',#82275);
#15252=VERTEX_POINT('',#82276);
#15253=VERTEX_POINT('',#82278);
#15254=VERTEX_POINT('',#82280);
#15255=VERTEX_POINT('',#82284);
#15256=VERTEX_POINT('',#82286);
#15257=VERTEX_POINT('',#82298);
#15258=VERTEX_POINT('',#82299);
#15259=VERTEX_POINT('',#82301);
#15260=VERTEX_POINT('',#82303);
#15261=VERTEX_POINT('',#82440);
#15262=VERTEX_POINT('',#82442);
#15263=VERTEX_POINT('',#82446);
#15264=VERTEX_POINT('',#82447);
#15265=VERTEX_POINT('',#82449);
#15266=VERTEX_POINT('',#82451);
#15267=VERTEX_POINT('',#82455);
#15268=VERTEX_POINT('',#82457);
#15269=VERTEX_POINT('',#82461);
#15270=VERTEX_POINT('',#82463);
#15271=VERTEX_POINT('',#82466);
#15272=VERTEX_POINT('',#82468);
#15273=VERTEX_POINT('',#82470);
#15274=VERTEX_POINT('',#82472);
#15275=VERTEX_POINT('',#82474);
#15276=VERTEX_POINT('',#82476);
#15277=VERTEX_POINT('',#82478);
#15278=VERTEX_POINT('',#82545);
#15279=VERTEX_POINT('',#82547);
#15280=VERTEX_POINT('',#82603);
#15281=VERTEX_POINT('',#82614);
#15282=VERTEX_POINT('',#82620);
#15283=VERTEX_POINT('',#82624);
#15284=VERTEX_POINT('',#82628);
#15285=VERTEX_POINT('',#82632);
#15286=VERTEX_POINT('',#82636);
#15287=VERTEX_POINT('',#82640);
#15288=VERTEX_POINT('',#82646);
#15289=VERTEX_POINT('',#82648);
#15290=VERTEX_POINT('',#82668);
#15291=VERTEX_POINT('',#82726);
#15292=VERTEX_POINT('',#82730);
#15293=VERTEX_POINT('',#82769);
#15294=VERTEX_POINT('',#82911);
#15295=VERTEX_POINT('',#82917);
#15296=VERTEX_POINT('',#82921);
#15297=VERTEX_POINT('',#82925);
#15298=VERTEX_POINT('',#82929);
#15299=VERTEX_POINT('',#83027);
#15300=VERTEX_POINT('',#83029);
#15301=VERTEX_POINT('',#83167);
#15302=VERTEX_POINT('',#83177);
#18780=EDGE_CURVE('',#14926,#14927,#1763,.T.);
#18781=EDGE_CURVE('',#14928,#14926,#606,.T.);
#18782=EDGE_CURVE('',#14928,#14929,#12037,.T.);
#18783=EDGE_CURVE('',#14929,#14930,#607,.T.);
#18784=EDGE_CURVE('',#14930,#14931,#1764,.T.);
#18785=EDGE_CURVE('',#14927,#14931,#12038,.T.);
#18786=EDGE_CURVE('',#14932,#14933,#608,.T.);
#18787=EDGE_CURVE('',#14934,#14932,#12039,.T.);
#18788=EDGE_CURVE('',#14934,#14935,#12040,.T.);
#18789=EDGE_CURVE('',#14935,#14936,#12041,.T.);
#18790=EDGE_CURVE('',#14936,#14937,#12042,.T.);
#18791=EDGE_CURVE('',#14933,#14937,#12043,.T.);
#18792=EDGE_CURVE('',#14938,#14939,#12044,.T.);
#18793=EDGE_CURVE('',#14939,#14940,#12045,.T.);
#18794=EDGE_CURVE('',#14941,#14940,#12046,.T.);
#18795=EDGE_CURVE('',#14942,#14941,#12047,.T.);
#18796=EDGE_CURVE('',#14943,#14942,#12048,.T.);
#18797=EDGE_CURVE('',#14943,#14938,#12049,.T.);
#18798=EDGE_CURVE('',#14944,#14945,#12050,.T.);
#18799=EDGE_CURVE('',#14945,#14946,#1765,.T.);
#18800=EDGE_CURVE('',#14947,#14946,#12051,.T.);
#18801=EDGE_CURVE('',#14948,#14947,#12052,.T.);
#18802=EDGE_CURVE('',#14949,#14948,#12053,.T.);
#18803=EDGE_CURVE('',#14949,#14944,#12054,.T.);
#18804=EDGE_CURVE('',#14950,#14951,#609,.T.);
#18805=EDGE_CURVE('',#14951,#14952,#1766,.T.);
#18806=EDGE_CURVE('',#14953,#14952,#12055,.T.);
#18807=EDGE_CURVE('',#14954,#14953,#1767,.T.);
#18808=EDGE_CURVE('',#14955,#14954,#610,.T.);
#18809=EDGE_CURVE('',#14955,#14950,#12056,.T.);
#18810=EDGE_CURVE('',#14956,#14957,#12057,.T.);
#18811=EDGE_CURVE('',#14958,#14957,#1768,.T.);
#18812=EDGE_CURVE('',#14959,#14958,#12058,.T.);
#18813=EDGE_CURVE('',#14960,#14959,#1769,.T.);
#18814=EDGE_CURVE('',#14961,#14960,#1770,.T.);
#18815=EDGE_CURVE('',#14961,#14956,#12059,.T.);
#18816=EDGE_CURVE('',#14962,#14963,#8446,.T.);
#18817=EDGE_CURVE('',#14962,#14963,#12060,.T.);
#18818=EDGE_CURVE('',#14964,#14962,#1771,.T.);
#18819=EDGE_CURVE('',#14964,#14965,#8447,.T.);
#18820=EDGE_CURVE('',#14963,#14965,#1772,.T.);
#18821=EDGE_CURVE('',#14966,#14967,#8448,.T.);
#18822=EDGE_CURVE('',#14965,#14966,#12061,.T.);
#18823=EDGE_CURVE('',#14967,#14964,#12062,.T.);
#18824=EDGE_CURVE('',#14957,#14967,#1773,.T.);
#18825=EDGE_CURVE('',#14956,#14957,#8449,.T.);
#18826=EDGE_CURVE('',#14966,#14956,#1774,.T.);
#18827=EDGE_CURVE('',#14968,#14964,#12063,.T.);
#18828=EDGE_CURVE('',#14968,#14962,#12064,.T.);
#18829=EDGE_CURVE('',#14969,#14967,#12065,.T.);
#18830=EDGE_CURVE('',#14969,#14968,#12066,.T.);
#18831=EDGE_CURVE('',#14958,#14969,#1775,.T.);
#18832=EDGE_CURVE('',#14970,#14971,#1776,.T.);
#18833=EDGE_CURVE('',#14971,#14972,#12067,.T.);
#18834=EDGE_CURVE('',#14972,#14961,#1777,.T.);
#18835=EDGE_CURVE('',#14960,#14973,#12068,.T.);
#18836=EDGE_CURVE('',#14968,#14970,#12069,.T.);
#18837=EDGE_CURVE('',#14974,#14975,#12070,.T.);
#18838=EDGE_CURVE('',#14976,#14974,#1778,.T.);
#18839=EDGE_CURVE('',#14977,#14976,#12071,.T.);
#18840=EDGE_CURVE('',#14950,#14977,#1779,.T.);
#18841=EDGE_CURVE('',#14978,#14955,#1780,.T.);
#18842=EDGE_CURVE('',#14979,#14978,#12072,.T.);
#18843=EDGE_CURVE('',#14980,#14979,#12073,.T.);
#18844=EDGE_CURVE('',#14944,#14980,#1781,.T.);
#18845=EDGE_CURVE('',#14981,#14949,#1782,.T.);
#18846=EDGE_CURVE('',#14982,#14981,#12074,.T.);
#18847=EDGE_CURVE('',#14938,#14982,#1783,.T.);
#18848=EDGE_CURVE('',#14983,#14943,#1784,.T.);
#18849=EDGE_CURVE('',#14984,#14983,#12075,.T.);
#18850=EDGE_CURVE('',#14935,#14984,#1785,.T.);
#18851=EDGE_CURVE('',#14985,#14934,#1786,.T.);
#18852=EDGE_CURVE('',#14986,#14985,#12076,.T.);
#18853=EDGE_CURVE('',#14987,#14986,#12077,.T.);
#18854=EDGE_CURVE('',#14929,#14987,#1787,.T.);
#18855=EDGE_CURVE('',#14988,#14928,#1788,.T.);
#18856=EDGE_CURVE('',#14989,#14988,#12078,.T.);
#18857=EDGE_CURVE('',#14975,#14989,#1789,.T.);
#18858=EDGE_CURVE('',#14971,#14963,#12079,.T.);
#18859=EDGE_CURVE('',#14971,#14965,#12080,.T.);
#18860=EDGE_CURVE('',#14972,#14966,#12081,.T.);
#18861=EDGE_CURVE('',#14990,#14990,#12082,.T.);
#18862=EDGE_CURVE('',#14990,#14991,#8450,.T.);
#18863=EDGE_CURVE('',#14991,#14991,#12083,.T.);
#18864=EDGE_CURVE('',#14992,#14993,#12084,.T.);
#18865=EDGE_CURVE('',#14994,#14993,#8451,.T.);
#18866=EDGE_CURVE('',#14995,#14994,#12085,.T.);
#18867=EDGE_CURVE('',#14996,#14995,#8452,.T.);
#18868=EDGE_CURVE('',#14997,#14996,#12086,.T.);
#18869=EDGE_CURVE('',#14998,#14997,#8453,.T.);
#18870=EDGE_CURVE('',#14999,#14998,#12087,.T.);
#18871=EDGE_CURVE('',#14992,#14999,#8454,.T.);
#18872=EDGE_CURVE('',#14999,#15000,#12088,.T.);
#18873=EDGE_CURVE('',#15001,#15000,#8455,.T.);
#18874=EDGE_CURVE('',#14992,#15001,#611,.T.);
#18875=EDGE_CURVE('',#14998,#15002,#12089,.T.);
#18876=EDGE_CURVE('',#15000,#15002,#12090,.T.);
#18877=EDGE_CURVE('',#14997,#15003,#12091,.T.);
#18878=EDGE_CURVE('',#15002,#15003,#8456,.T.);
#18879=EDGE_CURVE('',#14996,#15004,#12092,.T.);
#18880=EDGE_CURVE('',#15003,#15004,#12093,.T.);
#18881=EDGE_CURVE('',#14995,#15005,#12094,.T.);
#18882=EDGE_CURVE('',#15004,#15005,#8457,.T.);
#18883=EDGE_CURVE('',#14994,#15006,#12095,.T.);
#18884=EDGE_CURVE('',#15005,#15006,#12096,.T.);
#18885=EDGE_CURVE('',#14993,#15007,#12097,.T.);
#18886=EDGE_CURVE('',#15006,#15007,#8458,.T.);
#18887=EDGE_CURVE('',#14993,#15008,#1790,.T.);
#18888=EDGE_CURVE('',#15009,#14992,#1791,.T.);
#18889=EDGE_CURVE('',#15010,#15009,#1792,.T.);
#18890=EDGE_CURVE('',#15011,#15010,#1793,.T.);
#18891=EDGE_CURVE('',#15011,#15012,#12098,.T.);
#18892=EDGE_CURVE('',#15012,#15013,#12099,.T.);
#18893=EDGE_CURVE('',#15008,#15013,#12100,.T.);
#18894=EDGE_CURVE('',#15014,#15015,#8459,.T.);
#18895=EDGE_CURVE('',#15015,#15016,#8460,.T.);
#18896=EDGE_CURVE('',#15016,#15001,#1794,.T.);
#18897=EDGE_CURVE('',#15000,#15014,#8461,.T.);
#18898=EDGE_CURVE('',#15009,#15016,#612,.T.);
#18899=EDGE_CURVE('',#15002,#15017,#8462,.T.);
#18900=EDGE_CURVE('',#15017,#15014,#12101,.T.);
#18901=EDGE_CURVE('',#15018,#15017,#8463,.T.);
#18902=EDGE_CURVE('',#15018,#15003,#8464,.T.);
#18903=EDGE_CURVE('',#15019,#15018,#12102,.T.);
#18904=EDGE_CURVE('',#15019,#15004,#8465,.T.);
#18905=EDGE_CURVE('',#15020,#15019,#8466,.T.);
#18906=EDGE_CURVE('',#15020,#15005,#8467,.T.);
#18907=EDGE_CURVE('',#15021,#15020,#12103,.T.);
#18908=EDGE_CURVE('',#15021,#15006,#8468,.T.);
#18909=EDGE_CURVE('',#15008,#15022,#613,.T.);
#18910=EDGE_CURVE('',#15007,#15022,#1795,.T.);
#18911=EDGE_CURVE('',#15022,#15023,#1796,.T.);
#18912=EDGE_CURVE('',#15023,#15024,#8469,.T.);
#18913=EDGE_CURVE('',#15024,#15025,#8470,.T.);
#18914=EDGE_CURVE('',#15026,#15025,#8471,.T.);
#18915=EDGE_CURVE('',#15026,#15021,#8472,.T.);
#18916=EDGE_CURVE('',#15010,#15027,#614,.T.);
#18917=EDGE_CURVE('',#15028,#15027,#1797,.T.);
#18918=EDGE_CURVE('',#15011,#15028,#615,.T.);
#18919=EDGE_CURVE('',#15027,#15016,#1798,.T.);
#18920=EDGE_CURVE('',#15029,#15012,#12104,.T.);
#18921=EDGE_CURVE('',#15029,#15011,#1799,.T.);
#18922=EDGE_CURVE('',#15030,#15031,#12105,.T.);
#18923=EDGE_CURVE('',#15031,#15013,#8473,.T.);
#18924=EDGE_CURVE('',#15030,#15012,#8474,.T.);
#18925=EDGE_CURVE('',#15013,#15032,#12106,.T.);
#18926=EDGE_CURVE('',#15008,#15032,#1800,.T.);
#18927=EDGE_CURVE('',#15014,#15033,#12107,.T.);
#18928=EDGE_CURVE('',#15033,#15034,#8475,.T.);
#18929=EDGE_CURVE('',#15015,#15034,#12108,.T.);
#18930=EDGE_CURVE('',#15015,#15035,#12109,.T.);
#18931=EDGE_CURVE('',#15035,#15027,#8476,.T.);
#18932=EDGE_CURVE('',#15017,#15036,#12110,.T.);
#18933=EDGE_CURVE('',#15036,#15033,#12111,.T.);
#18934=EDGE_CURVE('',#15018,#15037,#12112,.T.);
#18935=EDGE_CURVE('',#15037,#15036,#8477,.T.);
#18936=EDGE_CURVE('',#15019,#15038,#12113,.T.);
#18937=EDGE_CURVE('',#15038,#15037,#12114,.T.);
#18938=EDGE_CURVE('',#15020,#15039,#12115,.T.);
#18939=EDGE_CURVE('',#15039,#15038,#8478,.T.);
#18940=EDGE_CURVE('',#15021,#15040,#12116,.T.);
#18941=EDGE_CURVE('',#15040,#15039,#12117,.T.);
#18942=EDGE_CURVE('',#15032,#15023,#12118,.T.);
#18943=EDGE_CURVE('',#15041,#15024,#12119,.T.);
#18944=EDGE_CURVE('',#15032,#15041,#8479,.T.);
#18945=EDGE_CURVE('',#15042,#15043,#8480,.T.);
#18946=EDGE_CURVE('',#15043,#15025,#12120,.T.);
#18947=EDGE_CURVE('',#15042,#15024,#12121,.T.);
#18948=EDGE_CURVE('',#15044,#15026,#12122,.T.);
#18949=EDGE_CURVE('',#15025,#15045,#12123,.T.);
#18950=EDGE_CURVE('',#15044,#15045,#8481,.T.);
#18951=EDGE_CURVE('',#15026,#15046,#12124,.T.);
#18952=EDGE_CURVE('',#15046,#15040,#8482,.T.);
#18953=EDGE_CURVE('',#15035,#15047,#8483,.T.);
#18954=EDGE_CURVE('',#15047,#15048,#8484,.T.);
#18955=EDGE_CURVE('',#15048,#15049,#8485,.T.);
#18956=EDGE_CURVE('',#15049,#15050,#8486,.T.);
#18957=EDGE_CURVE('',#15050,#15028,#1801,.T.);
#18958=EDGE_CURVE('',#15029,#15050,#12125,.T.);
#18959=EDGE_CURVE('',#15051,#15029,#8487,.T.);
#18960=EDGE_CURVE('',#15051,#15030,#12126,.T.);
#18961=EDGE_CURVE('',#15052,#15053,#12127,.T.);
#18962=EDGE_CURVE('',#15053,#15031,#12128,.T.);
#18963=EDGE_CURVE('',#15052,#15030,#12129,.T.);
#18964=EDGE_CURVE('',#15031,#15041,#12130,.T.);
#18965=EDGE_CURVE('',#15034,#15054,#12131,.T.);
#18966=EDGE_CURVE('',#15035,#15054,#12132,.T.);
#18967=EDGE_CURVE('',#15055,#15056,#8488,.T.);
#18968=EDGE_CURVE('',#15057,#15055,#12133,.T.);
#18969=EDGE_CURVE('',#15058,#15057,#8489,.T.);
#18970=EDGE_CURVE('',#15059,#15058,#8490,.T.);
#18971=EDGE_CURVE('',#15060,#15059,#8491,.T.);
#18972=EDGE_CURVE('',#15061,#15060,#12134,.T.);
#18973=EDGE_CURVE('',#15062,#15061,#8492,.T.);
#18974=EDGE_CURVE('',#15063,#15062,#8493,.T.);
#18975=EDGE_CURVE('',#15064,#15063,#8494,.T.);
#18976=EDGE_CURVE('',#15065,#15064,#12135,.T.);
#18977=EDGE_CURVE('',#15066,#15065,#8495,.T.);
#18978=EDGE_CURVE('',#15067,#15066,#12136,.T.);
#18979=EDGE_CURVE('',#15068,#15067,#8496,.T.);
#18980=EDGE_CURVE('',#15069,#15068,#12137,.T.);
#18981=EDGE_CURVE('',#15070,#15069,#8497,.T.);
#18982=EDGE_CURVE('',#15071,#15070,#12138,.T.);
#18983=EDGE_CURVE('',#15072,#15071,#8498,.T.);
#18984=EDGE_CURVE('',#15073,#15072,#12139,.T.);
#18985=EDGE_CURVE('',#15074,#15073,#12140,.T.);
#18986=EDGE_CURVE('',#15075,#15074,#8499,.T.);
#18987=EDGE_CURVE('',#15076,#15075,#12141,.T.);
#18988=EDGE_CURVE('',#15077,#15076,#8500,.T.);
#18989=EDGE_CURVE('',#15078,#15077,#12142,.T.);
#18990=EDGE_CURVE('',#15054,#15078,#8501,.T.);
#18991=EDGE_CURVE('',#15079,#15046,#12143,.T.);
#18992=EDGE_CURVE('',#15080,#15079,#8502,.T.);
#18993=EDGE_CURVE('',#15081,#15080,#12144,.T.);
#18994=EDGE_CURVE('',#15082,#15081,#8503,.T.);
#18995=EDGE_CURVE('',#15083,#15082,#12145,.T.);
#18996=EDGE_CURVE('',#15084,#15083,#12146,.T.);
#18997=EDGE_CURVE('',#15085,#15084,#8504,.T.);
#18998=EDGE_CURVE('',#15086,#15085,#12147,.T.);
#18999=EDGE_CURVE('',#15056,#15086,#8505,.T.);
#19000=EDGE_CURVE('',#15042,#15041,#12148,.T.);
#19001=EDGE_CURVE('',#14978,#15087,#12149,.T.);
#19002=EDGE_CURVE('',#15088,#15087,#12150,.T.);
#19003=EDGE_CURVE('',#14979,#15088,#12151,.T.);
#19004=EDGE_CURVE('',#15089,#15087,#12152,.T.);
#19005=EDGE_CURVE('',#15090,#15089,#8506,.T.);
#19006=EDGE_CURVE('',#15043,#15090,#12153,.T.);
#19007=EDGE_CURVE('',#15053,#15042,#12154,.T.);
#19008=EDGE_CURVE('',#15091,#15052,#12155,.T.);
#19009=EDGE_CURVE('',#15092,#15091,#8507,.T.);
#19010=EDGE_CURVE('',#15093,#15092,#12156,.T.);
#19011=EDGE_CURVE('',#15088,#15093,#8508,.T.);
#19012=EDGE_CURVE('',#15094,#15094,#12157,.T.);
#19013=EDGE_CURVE('',#15090,#15045,#12158,.T.);
#19014=EDGE_CURVE('',#15045,#15095,#8509,.T.);
#19015=EDGE_CURVE('',#15096,#15095,#8510,.T.);
#19016=EDGE_CURVE('',#15096,#15044,#8511,.T.);
#19017=EDGE_CURVE('',#15044,#15079,#12159,.T.);
#19018=EDGE_CURVE('',#15091,#15049,#12160,.T.);
#19019=EDGE_CURVE('',#15092,#15048,#12161,.T.);
#19020=EDGE_CURVE('',#15049,#15051,#12162,.T.);
#19021=EDGE_CURVE('',#15047,#15097,#12163,.T.);
#19022=EDGE_CURVE('',#15097,#15098,#8512,.T.);
#19023=EDGE_CURVE('',#15098,#15048,#12164,.T.);
#19024=EDGE_CURVE('',#15047,#15078,#12165,.T.);
#19025=EDGE_CURVE('',#15091,#15051,#12166,.T.);
#19026=EDGE_CURVE('',#15099,#15086,#12167,.T.);
#19027=EDGE_CURVE('',#15100,#15099,#8513,.T.);
#19028=EDGE_CURVE('',#15056,#15100,#616,.T.);
#19029=EDGE_CURVE('',#15101,#15085,#12168,.T.);
#19030=EDGE_CURVE('',#15099,#15101,#12169,.T.);
#19031=EDGE_CURVE('',#15102,#15084,#12170,.T.);
#19032=EDGE_CURVE('',#15101,#15102,#8514,.T.);
#19033=EDGE_CURVE('',#15103,#15083,#12171,.T.);
#19034=EDGE_CURVE('',#15102,#15103,#12172,.T.);
#19035=EDGE_CURVE('',#15104,#15082,#12173,.T.);
#19036=EDGE_CURVE('',#15103,#15104,#12174,.T.);
#19037=EDGE_CURVE('',#15105,#15082,#12175,.T.);
#19038=EDGE_CURVE('',#15106,#15081,#12176,.T.);
#19039=EDGE_CURVE('',#15105,#15106,#8515,.T.);
#19040=EDGE_CURVE('',#15096,#15080,#12177,.T.);
#19041=EDGE_CURVE('',#15106,#15096,#12178,.T.);
#19042=EDGE_CURVE('',#15097,#15077,#12179,.T.);
#19043=EDGE_CURVE('',#15107,#15076,#12180,.T.);
#19044=EDGE_CURVE('',#15097,#15107,#8516,.T.);
#19045=EDGE_CURVE('',#15108,#15075,#12181,.T.);
#19046=EDGE_CURVE('',#15107,#15108,#12182,.T.);
#19047=EDGE_CURVE('',#15109,#15074,#12183,.T.);
#19048=EDGE_CURVE('',#15108,#15109,#8517,.T.);
#19049=EDGE_CURVE('',#15110,#15074,#12184,.T.);
#19050=EDGE_CURVE('',#15111,#15073,#12185,.T.);
#19051=EDGE_CURVE('',#15110,#15111,#12186,.T.);
#19052=EDGE_CURVE('',#15112,#15072,#12187,.T.);
#19053=EDGE_CURVE('',#15111,#15112,#12188,.T.);
#19054=EDGE_CURVE('',#15113,#15071,#12189,.T.);
#19055=EDGE_CURVE('',#15112,#15113,#8518,.T.);
#19056=EDGE_CURVE('',#15114,#15070,#12190,.T.);
#19057=EDGE_CURVE('',#15113,#15114,#12191,.T.);
#19058=EDGE_CURVE('',#15115,#15069,#12192,.T.);
#19059=EDGE_CURVE('',#15114,#15115,#8519,.T.);
#19060=EDGE_CURVE('',#15116,#15068,#12193,.T.);
#19061=EDGE_CURVE('',#15115,#15116,#12194,.T.);
#19062=EDGE_CURVE('',#15117,#15067,#12195,.T.);
#19063=EDGE_CURVE('',#15116,#15117,#8520,.T.);
#19064=EDGE_CURVE('',#15118,#15066,#12196,.T.);
#19065=EDGE_CURVE('',#15117,#15118,#12197,.T.);
#19066=EDGE_CURVE('',#15119,#15065,#12198,.T.);
#19067=EDGE_CURVE('',#15118,#15119,#8521,.T.);
#19068=EDGE_CURVE('',#15120,#15064,#12199,.T.);
#19069=EDGE_CURVE('',#15119,#15120,#12200,.T.);
#19070=EDGE_CURVE('',#15121,#15063,#12201,.T.);
#19071=EDGE_CURVE('',#15120,#15121,#8522,.T.);
#19072=EDGE_CURVE('',#15122,#15063,#12202,.T.);
#19073=EDGE_CURVE('',#15123,#15062,#12203,.T.);
#19074=EDGE_CURVE('',#15122,#15123,#8523,.T.);
#19075=EDGE_CURVE('',#15124,#15062,#12204,.T.);
#19076=EDGE_CURVE('',#15125,#15061,#12205,.T.);
#19077=EDGE_CURVE('',#15124,#15125,#8524,.T.);
#19078=EDGE_CURVE('',#15126,#15060,#12206,.T.);
#19079=EDGE_CURVE('',#15125,#15126,#12207,.T.);
#19080=EDGE_CURVE('',#15127,#15059,#12208,.T.);
#19081=EDGE_CURVE('',#15126,#15127,#8525,.T.);
#19082=EDGE_CURVE('',#15128,#15059,#12209,.T.);
#19083=EDGE_CURVE('',#15129,#15058,#12210,.T.);
#19084=EDGE_CURVE('',#15128,#15129,#8526,.T.);
#19085=EDGE_CURVE('',#15130,#15058,#12211,.T.);
#19086=EDGE_CURVE('',#15131,#15057,#12212,.T.);
#19087=EDGE_CURVE('',#15130,#15131,#8527,.T.);
#19088=EDGE_CURVE('',#15132,#15055,#12213,.T.);
#19089=EDGE_CURVE('',#15131,#15132,#12214,.T.);
#19090=EDGE_CURVE('',#15132,#15100,#8528,.T.);
#19091=EDGE_CURVE('',#15133,#15134,#12215,.T.);
#19092=EDGE_CURVE('',#15134,#15133,#12216,.T.);
#19093=EDGE_CURVE('',#15133,#15094,#12217,.T.);
#19094=EDGE_CURVE('',#15093,#15098,#12218,.T.);
#19095=EDGE_CURVE('',#14981,#15135,#12219,.T.);
#19096=EDGE_CURVE('',#15136,#15135,#12220,.T.);
#19097=EDGE_CURVE('',#14982,#15136,#12221,.T.);
#19098=EDGE_CURVE('',#15110,#15135,#8529,.T.);
#19099=EDGE_CURVE('',#15111,#15136,#8530,.T.);
#19100=EDGE_CURVE('',#14983,#15137,#12222,.T.);
#19101=EDGE_CURVE('',#15138,#15137,#12223,.T.);
#19102=EDGE_CURVE('',#14984,#15138,#12224,.T.);
#19103=EDGE_CURVE('',#15137,#15139,#8531,.T.);
#19104=EDGE_CURVE('',#15140,#15139,#12225,.T.);
#19105=EDGE_CURVE('',#15140,#15138,#8532,.T.);
#19106=EDGE_CURVE('',#14976,#15141,#12226,.T.);
#19107=EDGE_CURVE('',#15142,#15141,#12227,.T.);
#19108=EDGE_CURVE('',#14977,#15142,#1802,.T.);
#19109=EDGE_CURVE('',#15103,#15141,#8533,.T.);
#19110=EDGE_CURVE('',#15104,#15142,#8534,.T.);
#19111=EDGE_CURVE('',#14988,#15143,#1803,.T.);
#19112=EDGE_CURVE('',#15144,#15143,#12228,.T.);
#19113=EDGE_CURVE('',#14989,#15144,#12229,.T.);
#19114=EDGE_CURVE('',#15145,#15143,#8535,.T.);
#19115=EDGE_CURVE('',#15146,#15145,#12230,.T.);
#19116=EDGE_CURVE('',#15144,#15146,#8536,.T.);
#19117=EDGE_CURVE('',#15147,#15088,#12231,.T.);
#19118=EDGE_CURVE('',#14979,#15147,#12232,.T.);
#19119=EDGE_CURVE('',#15147,#15098,#8537,.T.);
#19120=EDGE_CURVE('',#14978,#15148,#1804,.T.);
#19121=EDGE_CURVE('',#15087,#15148,#12233,.T.);
#19122=EDGE_CURVE('',#15095,#15148,#12234,.T.);
#19123=EDGE_CURVE('',#15089,#15095,#12235,.T.);
#19124=EDGE_CURVE('',#15148,#14953,#1805,.T.);
#19125=EDGE_CURVE('',#15106,#14953,#8538,.T.);
#19126=EDGE_CURVE('',#15149,#15147,#12236,.T.);
#19127=EDGE_CURVE('',#14980,#15149,#12237,.T.);
#19128=EDGE_CURVE('',#15107,#15149,#8539,.T.);
#19129=EDGE_CURVE('',#15099,#15150,#8540,.T.);
#19130=EDGE_CURVE('',#15151,#15150,#8541,.T.);
#19131=EDGE_CURVE('',#15100,#15151,#8542,.T.);
#19132=EDGE_CURVE('',#15101,#15152,#8543,.T.);
#19133=EDGE_CURVE('',#15150,#15152,#12238,.T.);
#19134=EDGE_CURVE('',#14975,#15153,#12239,.T.);
#19135=EDGE_CURVE('',#15154,#15153,#12240,.T.);
#19136=EDGE_CURVE('',#14974,#15154,#12241,.T.);
#19137=EDGE_CURVE('',#15153,#15155,#8544,.T.);
#19138=EDGE_CURVE('',#15152,#15155,#8545,.T.);
#19139=EDGE_CURVE('',#15102,#15154,#8546,.T.);
#19140=EDGE_CURVE('',#15153,#15144,#1806,.T.);
#19141=EDGE_CURVE('',#15155,#15146,#12242,.T.);
#19142=EDGE_CURVE('',#15141,#15154,#1807,.T.);
#19143=EDGE_CURVE('',#15104,#15105,#12243,.T.);
#19144=EDGE_CURVE('',#15105,#14952,#8547,.T.);
#19145=EDGE_CURVE('',#14946,#15149,#1808,.T.);
#19146=EDGE_CURVE('',#15108,#14946,#8548,.T.);
#19147=EDGE_CURVE('',#15109,#14947,#8549,.T.);
#19148=EDGE_CURVE('',#15109,#15110,#12244,.T.);
#19149=EDGE_CURVE('',#14940,#15136,#1809,.T.);
#19150=EDGE_CURVE('',#15112,#14940,#8550,.T.);
#19151=EDGE_CURVE('',#15137,#14941,#1810,.T.);
#19152=EDGE_CURVE('',#14941,#15156,#8551,.T.);
#19153=EDGE_CURVE('',#15139,#15156,#12245,.T.);
#19154=EDGE_CURVE('',#15113,#15157,#8552,.T.);
#19155=EDGE_CURVE('',#15156,#15157,#8553,.T.);
#19156=EDGE_CURVE('',#15114,#15158,#8554,.T.);
#19157=EDGE_CURVE('',#15157,#15158,#12246,.T.);
#19158=EDGE_CURVE('',#15115,#15159,#8555,.T.);
#19159=EDGE_CURVE('',#15158,#15159,#8556,.T.);
#19160=EDGE_CURVE('',#15116,#15160,#8557,.T.);
#19161=EDGE_CURVE('',#15159,#15160,#12247,.T.);
#19162=EDGE_CURVE('',#15161,#15117,#8558,.T.);
#19163=EDGE_CURVE('',#15160,#15161,#8559,.T.);
#19164=EDGE_CURVE('',#15162,#15118,#8560,.T.);
#19165=EDGE_CURVE('',#15161,#15162,#12248,.T.);
#19166=EDGE_CURVE('',#15163,#15119,#8561,.T.);
#19167=EDGE_CURVE('',#15162,#15163,#8562,.T.);
#19168=EDGE_CURVE('',#15164,#15120,#8563,.T.);
#19169=EDGE_CURVE('',#15163,#15164,#12249,.T.);
#19170=EDGE_CURVE('',#15121,#15165,#8564,.T.);
#19171=EDGE_CURVE('',#15164,#15165,#8565,.T.);
#19172=EDGE_CURVE('',#15121,#15122,#12250,.T.);
#19173=EDGE_CURVE('',#15123,#15166,#8566,.T.);
#19174=EDGE_CURVE('',#15167,#15166,#8567,.T.);
#19175=EDGE_CURVE('',#15122,#15167,#8568,.T.);
#19176=EDGE_CURVE('',#15123,#15124,#12251,.T.);
#19177=EDGE_CURVE('',#15168,#15125,#8569,.T.);
#19178=EDGE_CURVE('',#15169,#15168,#8570,.T.);
#19179=EDGE_CURVE('',#15124,#15169,#8571,.T.);
#19180=EDGE_CURVE('',#15170,#15126,#8572,.T.);
#19181=EDGE_CURVE('',#15168,#15170,#12252,.T.);
#19182=EDGE_CURVE('',#15127,#15171,#8573,.T.);
#19183=EDGE_CURVE('',#15170,#15171,#8574,.T.);
#19184=EDGE_CURVE('',#15127,#15128,#12253,.T.);
#19185=EDGE_CURVE('',#15129,#15172,#8575,.T.);
#19186=EDGE_CURVE('',#15173,#15172,#8576,.T.);
#19187=EDGE_CURVE('',#15128,#15173,#8577,.T.);
#19188=EDGE_CURVE('',#15129,#15130,#12254,.T.);
#19189=EDGE_CURVE('',#15174,#15131,#8578,.T.);
#19190=EDGE_CURVE('',#15175,#15174,#8579,.T.);
#19191=EDGE_CURVE('',#15130,#15175,#8580,.T.);
#19192=EDGE_CURVE('',#15176,#15132,#8581,.T.);
#19193=EDGE_CURVE('',#15174,#15176,#12255,.T.);
#19194=EDGE_CURVE('',#15176,#15151,#8582,.T.);
#19195=EDGE_CURVE('',#15177,#15177,#12256,.T.);
#19196=EDGE_CURVE('',#15177,#15134,#8583,.T.);
#19197=EDGE_CURVE('',#15139,#15178,#12257,.T.);
#19198=EDGE_CURVE('',#15179,#15178,#12258,.T.);
#19199=EDGE_CURVE('',#15140,#15179,#12259,.T.);
#19200=EDGE_CURVE('',#14937,#15138,#1811,.T.);
#19201=EDGE_CURVE('',#15180,#15140,#12260,.T.);
#19202=EDGE_CURVE('',#15180,#14937,#8584,.T.);
#19203=EDGE_CURVE('',#14986,#15181,#12261,.T.);
#19204=EDGE_CURVE('',#15182,#15181,#12262,.T.);
#19205=EDGE_CURVE('',#14987,#15182,#12263,.T.);
#19206=EDGE_CURVE('',#15181,#15183,#8585,.T.);
#19207=EDGE_CURVE('',#15183,#15184,#12264,.T.);
#19208=EDGE_CURVE('',#15184,#15185,#8586,.T.);
#19209=EDGE_CURVE('',#15185,#15186,#12265,.T.);
#19210=EDGE_CURVE('',#15186,#15187,#12266,.T.);
#19211=EDGE_CURVE('',#15187,#15188,#12267,.T.);
#19212=EDGE_CURVE('',#15188,#15189,#8587,.T.);
#19213=EDGE_CURVE('',#15189,#15190,#12268,.T.);
#19214=EDGE_CURVE('',#15190,#15191,#8588,.T.);
#19215=EDGE_CURVE('',#15191,#15182,#12269,.T.);
#19216=EDGE_CURVE('',#15192,#15192,#12270,.T.);
#19217=EDGE_CURVE('',#15143,#14927,#1812,.T.);
#19218=EDGE_CURVE('',#15193,#14927,#8589,.T.);
#19219=EDGE_CURVE('',#15145,#15193,#12271,.T.);
#19220=EDGE_CURVE('',#15188,#15194,#12272,.T.);
#19221=EDGE_CURVE('',#15194,#15195,#12273,.T.);
#19222=EDGE_CURVE('',#15188,#15195,#12274,.T.);
#19223=EDGE_CURVE('',#15135,#14947,#1813,.T.);
#19224=EDGE_CURVE('',#14952,#15142,#1814,.T.);
#19225=EDGE_CURVE('',#15196,#15151,#617,.T.);
#19226=EDGE_CURVE('',#15150,#15197,#12275,.T.);
#19227=EDGE_CURVE('',#15196,#15197,#8590,.T.);
#19228=EDGE_CURVE('',#15152,#15198,#12276,.T.);
#19229=EDGE_CURVE('',#15197,#15198,#12277,.T.);
#19230=EDGE_CURVE('',#15155,#15199,#12278,.T.);
#19231=EDGE_CURVE('',#15198,#15199,#8591,.T.);
#19232=EDGE_CURVE('',#15146,#15200,#12279,.T.);
#19233=EDGE_CURVE('',#15199,#15200,#12280,.T.);
#19234=EDGE_CURVE('',#15156,#15201,#12281,.T.);
#19235=EDGE_CURVE('',#15178,#15201,#12282,.T.);
#19236=EDGE_CURVE('',#15157,#15202,#12283,.T.);
#19237=EDGE_CURVE('',#15201,#15202,#8592,.T.);
#19238=EDGE_CURVE('',#15158,#15203,#12284,.T.);
#19239=EDGE_CURVE('',#15202,#15203,#12285,.T.);
#19240=EDGE_CURVE('',#15159,#15204,#12286,.T.);
#19241=EDGE_CURVE('',#15203,#15204,#8593,.T.);
#19242=EDGE_CURVE('',#15160,#15205,#12287,.T.);
#19243=EDGE_CURVE('',#15204,#15205,#12288,.T.);
#19244=EDGE_CURVE('',#15161,#15206,#12289,.T.);
#19245=EDGE_CURVE('',#15205,#15206,#8594,.T.);
#19246=EDGE_CURVE('',#15162,#15207,#12290,.T.);
#19247=EDGE_CURVE('',#15206,#15207,#12291,.T.);
#19248=EDGE_CURVE('',#15163,#15208,#12292,.T.);
#19249=EDGE_CURVE('',#15207,#15208,#8595,.T.);
#19250=EDGE_CURVE('',#15164,#15209,#12293,.T.);
#19251=EDGE_CURVE('',#15208,#15209,#12294,.T.);
#19252=EDGE_CURVE('',#15165,#15210,#12295,.T.);
#19253=EDGE_CURVE('',#15209,#15210,#8596,.T.);
#19254=EDGE_CURVE('',#15165,#15167,#12296,.T.);
#19255=EDGE_CURVE('',#15166,#15211,#12297,.T.);
#19256=EDGE_CURVE('',#15210,#15211,#8597,.T.);
#19257=EDGE_CURVE('',#15167,#15210,#12298,.T.);
#19258=EDGE_CURVE('',#15166,#15169,#12299,.T.);
#19259=EDGE_CURVE('',#15168,#15212,#12300,.T.);
#19260=EDGE_CURVE('',#15211,#15212,#8598,.T.);
#19261=EDGE_CURVE('',#15169,#15211,#12301,.T.);
#19262=EDGE_CURVE('',#15170,#15213,#12302,.T.);
#19263=EDGE_CURVE('',#15212,#15213,#12303,.T.);
#19264=EDGE_CURVE('',#15171,#15214,#12304,.T.);
#19265=EDGE_CURVE('',#15213,#15214,#8599,.T.);
#19266=EDGE_CURVE('',#15171,#15173,#12305,.T.);
#19267=EDGE_CURVE('',#15172,#15215,#12306,.T.);
#19268=EDGE_CURVE('',#15214,#15215,#8600,.T.);
#19269=EDGE_CURVE('',#15173,#15214,#12307,.T.);
#19270=EDGE_CURVE('',#15172,#15175,#12308,.T.);
#19271=EDGE_CURVE('',#15174,#15216,#12309,.T.);
#19272=EDGE_CURVE('',#15215,#15216,#8601,.T.);
#19273=EDGE_CURVE('',#15175,#15215,#12310,.T.);
#19274=EDGE_CURVE('',#15176,#15217,#12311,.T.);
#19275=EDGE_CURVE('',#15216,#15217,#12312,.T.);
#19276=EDGE_CURVE('',#15217,#15196,#8602,.T.);
#19277=EDGE_CURVE('',#15218,#15218,#12313,.T.);
#19278=EDGE_CURVE('',#15180,#15179,#12314,.T.);
#19279=EDGE_CURVE('',#15219,#15219,#12315,.T.);
#19280=EDGE_CURVE('',#15219,#15220,#8603,.T.);
#19281=EDGE_CURVE('',#15221,#15220,#12316,.T.);
#19282=EDGE_CURVE('',#15220,#15221,#12317,.T.);
#19283=EDGE_CURVE('',#15222,#15180,#8604,.T.);
#19284=EDGE_CURVE('',#15222,#14933,#8605,.T.);
#19285=EDGE_CURVE('',#15223,#15223,#12318,.T.);
#19286=EDGE_CURVE('',#15223,#15192,#12319,.T.);
#19287=EDGE_CURVE('',#15184,#15224,#12320,.T.);
#19288=EDGE_CURVE('',#15224,#15225,#8606,.T.);
#19289=EDGE_CURVE('',#15185,#15225,#12321,.T.);
#19290=EDGE_CURVE('',#15183,#15226,#12322,.T.);
#19291=EDGE_CURVE('',#15226,#15224,#12323,.T.);
#19292=EDGE_CURVE('',#15189,#15227,#12324,.T.);
#19293=EDGE_CURVE('',#15227,#15228,#12325,.T.);
#19294=EDGE_CURVE('',#15190,#15228,#12326,.T.);
#19295=EDGE_CURVE('',#15195,#15227,#8607,.T.);
#19296=EDGE_CURVE('',#15187,#15229,#12327,.T.);
#19297=EDGE_CURVE('',#15229,#15194,#12328,.T.);
#19298=EDGE_CURVE('',#14986,#15230,#12329,.T.);
#19299=EDGE_CURVE('',#15181,#15230,#12330,.T.);
#19300=EDGE_CURVE('',#15230,#15226,#8608,.T.);
#19301=EDGE_CURVE('',#15231,#15182,#12331,.T.);
#19302=EDGE_CURVE('',#14987,#15231,#1815,.T.);
#19303=EDGE_CURVE('',#15191,#15232,#12332,.T.);
#19304=EDGE_CURVE('',#15232,#15231,#12333,.T.);
#19305=EDGE_CURVE('',#15228,#15232,#8609,.T.);
#19306=EDGE_CURVE('',#15185,#15233,#12334,.T.);
#19307=EDGE_CURVE('',#15233,#15234,#12335,.T.);
#19308=EDGE_CURVE('',#15186,#15234,#12336,.T.);
#19309=EDGE_CURVE('',#15234,#15229,#12337,.T.);
#19310=EDGE_CURVE('',#15235,#14931,#8610,.T.);
#19311=EDGE_CURVE('',#15193,#15235,#8611,.T.);
#19312=EDGE_CURVE('',#15221,#15236,#12338,.T.);
#19313=EDGE_CURVE('',#15237,#15236,#12339,.T.);
#19314=EDGE_CURVE('',#15238,#15237,#12340,.T.);
#19315=EDGE_CURVE('',#15236,#15238,#12341,.T.);
#19316=EDGE_CURVE('',#15239,#15239,#12342,.T.);
#19317=EDGE_CURVE('',#15239,#15218,#8612,.T.);
#19318=EDGE_CURVE('',#15240,#15179,#8613,.T.);
#19319=EDGE_CURVE('',#15222,#15240,#12343,.T.);
#19320=EDGE_CURVE('',#15241,#15222,#12344,.T.);
#19321=EDGE_CURVE('',#15242,#15240,#12345,.T.);
#19322=EDGE_CURVE('',#15241,#15242,#12346,.T.);
#19323=EDGE_CURVE('',#15243,#15241,#8614,.T.);
#19324=EDGE_CURVE('',#15244,#15242,#8615,.T.);
#19325=EDGE_CURVE('',#15243,#15244,#12347,.T.);
#19326=EDGE_CURVE('',#15245,#15243,#12348,.T.);
#19327=EDGE_CURVE('',#15246,#15244,#12349,.T.);
#19328=EDGE_CURVE('',#15245,#15246,#12350,.T.);
#19329=EDGE_CURVE('',#15247,#15245,#8616,.T.);
#19330=EDGE_CURVE('',#15248,#15246,#8617,.T.);
#19331=EDGE_CURVE('',#15247,#15248,#12351,.T.);
#19332=EDGE_CURVE('',#15225,#15233,#12352,.T.);
#19333=EDGE_CURVE('',#15245,#15224,#8618,.T.);
#19334=EDGE_CURVE('',#15243,#15226,#8619,.T.);
#19335=EDGE_CURVE('',#14985,#15249,#12353,.T.);
#19336=EDGE_CURVE('',#15230,#15249,#12354,.T.);
#19337=EDGE_CURVE('',#15241,#15249,#8620,.T.);
#19338=EDGE_CURVE('',#15219,#15250,#12355,.T.);
#19339=EDGE_CURVE('',#15250,#15250,#12356,.T.);
#19340=EDGE_CURVE('',#15251,#15252,#12357,.T.);
#19341=EDGE_CURVE('',#15252,#15253,#12358,.T.);
#19342=EDGE_CURVE('',#15254,#15253,#12359,.T.);
#19343=EDGE_CURVE('',#15251,#15254,#12360,.T.);
#19344=EDGE_CURVE('',#15255,#15194,#8621,.T.);
#19345=EDGE_CURVE('',#15255,#15256,#12361,.T.);
#19346=EDGE_CURVE('',#15256,#15195,#8622,.T.);
#19347=EDGE_CURVE('',#15257,#15258,#12362,.T.);
#19348=EDGE_CURVE('',#15258,#15259,#12363,.T.);
#19349=EDGE_CURVE('',#15260,#15259,#12364,.T.);
#19350=EDGE_CURVE('',#15257,#15260,#12365,.T.);
#19351=EDGE_CURVE('',#15253,#15258,#8623,.T.);
#19352=EDGE_CURVE('',#15254,#15257,#8624,.T.);
#19353=EDGE_CURVE('',#15249,#14933,#1816,.T.);
#19354=EDGE_CURVE('',#15223,#15250,#8625,.T.);
#19355=EDGE_CURVE('',#15259,#15261,#8626,.T.);
#19356=EDGE_CURVE('',#15262,#15261,#12366,.T.);
#19357=EDGE_CURVE('',#15260,#15262,#8627,.T.);
#19358=EDGE_CURVE('',#15263,#15264,#12367,.T.);
#19359=EDGE_CURVE('',#15264,#15265,#12368,.T.);
#19360=EDGE_CURVE('',#15266,#15265,#12369,.T.);
#19361=EDGE_CURVE('',#15263,#15266,#12370,.T.);
#19362=EDGE_CURVE('',#15267,#15263,#8628,.T.);
#19363=EDGE_CURVE('',#15268,#15266,#8629,.T.);
#19364=EDGE_CURVE('',#15267,#15268,#12371,.T.);
#19365=EDGE_CURVE('',#15200,#15269,#12372,.T.);
#19366=EDGE_CURVE('',#15269,#15270,#8630,.T.);
#19367=EDGE_CURVE('',#15270,#15268,#12373,.T.);
#19368=EDGE_CURVE('',#15265,#15271,#8631,.T.);
#19369=EDGE_CURVE('',#15271,#15272,#12374,.T.);
#19370=EDGE_CURVE('',#15272,#15273,#8632,.T.);
#19371=EDGE_CURVE('',#15273,#15274,#12375,.T.);
#19372=EDGE_CURVE('',#15274,#15275,#8633,.T.);
#19373=EDGE_CURVE('',#15275,#15276,#12376,.T.);
#19374=EDGE_CURVE('',#15276,#15277,#8634,.T.);
#19375=EDGE_CURVE('',#15277,#15248,#12377,.T.);
#19376=EDGE_CURVE('',#15145,#15269,#12378,.T.);
#19377=EDGE_CURVE('',#15193,#15269,#12379,.T.);
#19378=EDGE_CURVE('',#15235,#15270,#12380,.T.);
#19379=EDGE_CURVE('',#15235,#15267,#12381,.T.);
#19380=EDGE_CURVE('',#14931,#15231,#1817,.T.);
#19381=EDGE_CURVE('',#15267,#15232,#8635,.T.);
#19382=EDGE_CURVE('',#15263,#15228,#8636,.T.);
#19383=EDGE_CURVE('',#15264,#15227,#8637,.T.);
#19384=EDGE_CURVE('',#15264,#15278,#8638,.T.);
#19385=EDGE_CURVE('',#15279,#15256,#1818,.T.);
#19386=EDGE_CURVE('',#15280,#15279,#1819,.T.);
#19387=EDGE_CURVE('',#15281,#15280,#8639,.T.);
#19388=EDGE_CURVE('',#15278,#15281,#8640,.T.);
#19389=EDGE_CURVE('',#15278,#15271,#12382,.T.);
#19390=EDGE_CURVE('',#15278,#15282,#12383,.T.);
#19391=EDGE_CURVE('',#15282,#15272,#12384,.T.);
#19392=EDGE_CURVE('',#15282,#15283,#8641,.T.);
#19393=EDGE_CURVE('',#15283,#15273,#12385,.T.);
#19394=EDGE_CURVE('',#15283,#15284,#12386,.T.);
#19395=EDGE_CURVE('',#15284,#15274,#12387,.T.);
#19396=EDGE_CURVE('',#15284,#15285,#8642,.T.);
#19397=EDGE_CURVE('',#15285,#15275,#12388,.T.);
#19398=EDGE_CURVE('',#15285,#15286,#12389,.T.);
#19399=EDGE_CURVE('',#15286,#15276,#12390,.T.);
#19400=EDGE_CURVE('',#15286,#15287,#8643,.T.);
#19401=EDGE_CURVE('',#15287,#15277,#12391,.T.);
#19402=EDGE_CURVE('',#15287,#15247,#12392,.T.);
#19403=EDGE_CURVE('',#15287,#15288,#8644,.T.);
#19404=EDGE_CURVE('',#15289,#15288,#1820,.T.);
#19405=EDGE_CURVE('',#15247,#15289,#8645,.T.);
#19406=EDGE_CURVE('',#15252,#15286,#8646,.T.);
#19407=EDGE_CURVE('',#15290,#15252,#8647,.T.);
#19408=EDGE_CURVE('',#15288,#15290,#1821,.T.);
#19409=EDGE_CURVE('',#15253,#15285,#8648,.T.);
#19410=EDGE_CURVE('',#15284,#15258,#8649,.T.);
#19411=EDGE_CURVE('',#15283,#15259,#8650,.T.);
#19412=EDGE_CURVE('',#15282,#15261,#8651,.T.);
#19413=EDGE_CURVE('',#15261,#15281,#12393,.T.);
#19414=EDGE_CURVE('',#15291,#15281,#12394,.T.);
#19415=EDGE_CURVE('',#15262,#15291,#12395,.T.);
#19416=EDGE_CURVE('',#15292,#15280,#618,.T.);
#19417=EDGE_CURVE('',#15291,#15292,#8652,.T.);
#19418=EDGE_CURVE('',#15293,#15279,#619,.T.);
#19419=EDGE_CURVE('',#15292,#15293,#1822,.T.);
#19420=EDGE_CURVE('',#15293,#15255,#1823,.T.);
#19421=EDGE_CURVE('',#15294,#15255,#12396,.T.);
#19422=EDGE_CURVE('',#15293,#15294,#12397,.T.);
#19423=EDGE_CURVE('',#15229,#15294,#8653,.T.);
#19424=EDGE_CURVE('',#15234,#15295,#8654,.T.);
#19425=EDGE_CURVE('',#15295,#15294,#12398,.T.);
#19426=EDGE_CURVE('',#15233,#15296,#8655,.T.);
#19427=EDGE_CURVE('',#15296,#15295,#12399,.T.);
#19428=EDGE_CURVE('',#15225,#15297,#8656,.T.);
#19429=EDGE_CURVE('',#15296,#15297,#12400,.T.);
#19430=EDGE_CURVE('',#15298,#15289,#1824,.T.);
#19431=EDGE_CURVE('',#15297,#15298,#1825,.T.);
#19432=EDGE_CURVE('',#15299,#15298,#620,.T.);
#19433=EDGE_CURVE('',#15300,#15289,#621,.T.);
#19434=EDGE_CURVE('',#15299,#15300,#1826,.T.);
#19435=EDGE_CURVE('',#15296,#15299,#1827,.T.);
#19436=EDGE_CURVE('',#15299,#15295,#12401,.T.);
#19437=EDGE_CURVE('',#15300,#15301,#1828,.T.);
#19438=EDGE_CURVE('',#15301,#15302,#1829,.T.);
#19439=EDGE_CURVE('',#15302,#15292,#12402,.T.);
#19440=EDGE_CURVE('',#15301,#15288,#622,.T.);
#19441=EDGE_CURVE('',#15302,#15290,#623,.T.);
#19442=EDGE_CURVE('',#15302,#15251,#8657,.T.);
#26017=ORIENTED_EDGE('',*,*,#18780,.F.);
#26018=ORIENTED_EDGE('',*,*,#18781,.F.);
#26019=ORIENTED_EDGE('',*,*,#18782,.T.);
#26020=ORIENTED_EDGE('',*,*,#18783,.T.);
#26021=ORIENTED_EDGE('',*,*,#18784,.T.);
#26022=ORIENTED_EDGE('',*,*,#18785,.F.);
#26023=ORIENTED_EDGE('',*,*,#18786,.F.);
#26024=ORIENTED_EDGE('',*,*,#18787,.F.);
#26025=ORIENTED_EDGE('',*,*,#18788,.T.);
#26026=ORIENTED_EDGE('',*,*,#18789,.T.);
#26027=ORIENTED_EDGE('',*,*,#18790,.T.);
#26028=ORIENTED_EDGE('',*,*,#18791,.F.);
#26029=ORIENTED_EDGE('',*,*,#18792,.T.);
#26030=ORIENTED_EDGE('',*,*,#18793,.T.);
#26031=ORIENTED_EDGE('',*,*,#18794,.F.);
#26032=ORIENTED_EDGE('',*,*,#18795,.F.);
#26033=ORIENTED_EDGE('',*,*,#18796,.F.);
#26034=ORIENTED_EDGE('',*,*,#18797,.T.);
#26035=ORIENTED_EDGE('',*,*,#18798,.T.);
#26036=ORIENTED_EDGE('',*,*,#18799,.T.);
#26037=ORIENTED_EDGE('',*,*,#18800,.F.);
#26038=ORIENTED_EDGE('',*,*,#18801,.F.);
#26039=ORIENTED_EDGE('',*,*,#18802,.F.);
#26040=ORIENTED_EDGE('',*,*,#18803,.T.);
#26041=ORIENTED_EDGE('',*,*,#18804,.T.);
#26042=ORIENTED_EDGE('',*,*,#18805,.T.);
#26043=ORIENTED_EDGE('',*,*,#18806,.F.);
#26044=ORIENTED_EDGE('',*,*,#18807,.F.);
#26045=ORIENTED_EDGE('',*,*,#18808,.F.);
#26046=ORIENTED_EDGE('',*,*,#18809,.T.);
#26047=ORIENTED_EDGE('',*,*,#18810,.T.);
#26048=ORIENTED_EDGE('',*,*,#18811,.F.);
#26049=ORIENTED_EDGE('',*,*,#18812,.F.);
#26050=ORIENTED_EDGE('',*,*,#18813,.F.);
#26051=ORIENTED_EDGE('',*,*,#18814,.F.);
#26052=ORIENTED_EDGE('',*,*,#18815,.T.);
#26053=ORIENTED_EDGE('',*,*,#18816,.T.);
#26054=ORIENTED_EDGE('',*,*,#18817,.F.);
#26055=ORIENTED_EDGE('',*,*,#18818,.F.);
#26056=ORIENTED_EDGE('',*,*,#18819,.T.);
#26057=ORIENTED_EDGE('',*,*,#18820,.F.);
#26058=ORIENTED_EDGE('',*,*,#18816,.F.);
#26059=ORIENTED_EDGE('',*,*,#18821,.F.);
#26060=ORIENTED_EDGE('',*,*,#18822,.F.);
#26061=ORIENTED_EDGE('',*,*,#18819,.F.);
#26062=ORIENTED_EDGE('',*,*,#18823,.F.);
#26063=ORIENTED_EDGE('',*,*,#18821,.T.);
#26064=ORIENTED_EDGE('',*,*,#18824,.F.);
#26065=ORIENTED_EDGE('',*,*,#18825,.F.);
#26066=ORIENTED_EDGE('',*,*,#18826,.F.);
#26067=ORIENTED_EDGE('',*,*,#18810,.F.);
#26068=ORIENTED_EDGE('',*,*,#18825,.T.);
#26069=ORIENTED_EDGE('',*,*,#18827,.T.);
#26070=ORIENTED_EDGE('',*,*,#18818,.T.);
#26071=ORIENTED_EDGE('',*,*,#18828,.F.);
#26072=ORIENTED_EDGE('',*,*,#18829,.T.);
#26073=ORIENTED_EDGE('',*,*,#18823,.T.);
#26074=ORIENTED_EDGE('',*,*,#18827,.F.);
#26075=ORIENTED_EDGE('',*,*,#18830,.F.);
#26076=ORIENTED_EDGE('',*,*,#18811,.T.);
#26077=ORIENTED_EDGE('',*,*,#18824,.T.);
#26078=ORIENTED_EDGE('',*,*,#18829,.F.);
#26079=ORIENTED_EDGE('',*,*,#18831,.F.);
#26080=ORIENTED_EDGE('',*,*,#18832,.T.);
#26081=ORIENTED_EDGE('',*,*,#18833,.T.);
#26082=ORIENTED_EDGE('',*,*,#18834,.T.);
#26083=ORIENTED_EDGE('',*,*,#18814,.T.);
#26084=ORIENTED_EDGE('',*,*,#18835,.T.);
#26085=ORIENTED_EDGE('',*,*,#18835,.F.);
#26086=ORIENTED_EDGE('',*,*,#18813,.T.);
#26087=ORIENTED_EDGE('',*,*,#18812,.T.);
#26088=ORIENTED_EDGE('',*,*,#18831,.T.);
#26089=ORIENTED_EDGE('',*,*,#18830,.T.);
#26090=ORIENTED_EDGE('',*,*,#18836,.T.);
#26091=ORIENTED_EDGE('',*,*,#18837,.F.);
#26092=ORIENTED_EDGE('',*,*,#18838,.F.);
#26093=ORIENTED_EDGE('',*,*,#18839,.F.);
#26094=ORIENTED_EDGE('',*,*,#18840,.F.);
#26095=ORIENTED_EDGE('',*,*,#18809,.F.);
#26096=ORIENTED_EDGE('',*,*,#18841,.F.);
#26097=ORIENTED_EDGE('',*,*,#18842,.F.);
#26098=ORIENTED_EDGE('',*,*,#18843,.F.);
#26099=ORIENTED_EDGE('',*,*,#18844,.F.);
#26100=ORIENTED_EDGE('',*,*,#18803,.F.);
#26101=ORIENTED_EDGE('',*,*,#18845,.F.);
#26102=ORIENTED_EDGE('',*,*,#18846,.F.);
#26103=ORIENTED_EDGE('',*,*,#18847,.F.);
#26104=ORIENTED_EDGE('',*,*,#18797,.F.);
#26105=ORIENTED_EDGE('',*,*,#18848,.F.);
#26106=ORIENTED_EDGE('',*,*,#18849,.F.);
#26107=ORIENTED_EDGE('',*,*,#18850,.F.);
#26108=ORIENTED_EDGE('',*,*,#18788,.F.);
#26109=ORIENTED_EDGE('',*,*,#18851,.F.);
#26110=ORIENTED_EDGE('',*,*,#18852,.F.);
#26111=ORIENTED_EDGE('',*,*,#18853,.F.);
#26112=ORIENTED_EDGE('',*,*,#18854,.F.);
#26113=ORIENTED_EDGE('',*,*,#18782,.F.);
#26114=ORIENTED_EDGE('',*,*,#18855,.F.);
#26115=ORIENTED_EDGE('',*,*,#18856,.F.);
#26116=ORIENTED_EDGE('',*,*,#18857,.F.);
#26117=ORIENTED_EDGE('',*,*,#18858,.T.);
#26118=ORIENTED_EDGE('',*,*,#18820,.T.);
#26119=ORIENTED_EDGE('',*,*,#18859,.F.);
#26120=ORIENTED_EDGE('',*,*,#18859,.T.);
#26121=ORIENTED_EDGE('',*,*,#18822,.T.);
#26122=ORIENTED_EDGE('',*,*,#18860,.F.);
#26123=ORIENTED_EDGE('',*,*,#18833,.F.);
#26124=ORIENTED_EDGE('',*,*,#18860,.T.);
#26125=ORIENTED_EDGE('',*,*,#18826,.T.);
#26126=ORIENTED_EDGE('',*,*,#18815,.F.);
#26127=ORIENTED_EDGE('',*,*,#18834,.F.);
#26128=ORIENTED_EDGE('',*,*,#18828,.T.);
#26129=ORIENTED_EDGE('',*,*,#18817,.T.);
#26130=ORIENTED_EDGE('',*,*,#18858,.F.);
#26131=ORIENTED_EDGE('',*,*,#18832,.F.);
#26132=ORIENTED_EDGE('',*,*,#18836,.F.);
#26133=ORIENTED_EDGE('',*,*,#18861,.F.);
#26134=ORIENTED_EDGE('',*,*,#18861,.T.);
#26135=ORIENTED_EDGE('',*,*,#18862,.T.);
#26136=ORIENTED_EDGE('',*,*,#18863,.T.);
#26137=ORIENTED_EDGE('',*,*,#18862,.F.);
#26138=ORIENTED_EDGE('',*,*,#18864,.T.);
#26139=ORIENTED_EDGE('',*,*,#18865,.F.);
#26140=ORIENTED_EDGE('',*,*,#18866,.F.);
#26141=ORIENTED_EDGE('',*,*,#18867,.F.);
#26142=ORIENTED_EDGE('',*,*,#18868,.F.);
#26143=ORIENTED_EDGE('',*,*,#18869,.F.);
#26144=ORIENTED_EDGE('',*,*,#18870,.F.);
#26145=ORIENTED_EDGE('',*,*,#18871,.F.);
#26146=ORIENTED_EDGE('',*,*,#18863,.F.);
#26147=ORIENTED_EDGE('',*,*,#18871,.T.);
#26148=ORIENTED_EDGE('',*,*,#18872,.T.);
#26149=ORIENTED_EDGE('',*,*,#18873,.F.);
#26150=ORIENTED_EDGE('',*,*,#18874,.F.);
#26151=ORIENTED_EDGE('',*,*,#18870,.T.);
#26152=ORIENTED_EDGE('',*,*,#18875,.T.);
#26153=ORIENTED_EDGE('',*,*,#18876,.F.);
#26154=ORIENTED_EDGE('',*,*,#18872,.F.);
#26155=ORIENTED_EDGE('',*,*,#18869,.T.);
#26156=ORIENTED_EDGE('',*,*,#18877,.T.);
#26157=ORIENTED_EDGE('',*,*,#18878,.F.);
#26158=ORIENTED_EDGE('',*,*,#18875,.F.);
#26159=ORIENTED_EDGE('',*,*,#18868,.T.);
#26160=ORIENTED_EDGE('',*,*,#18879,.T.);
#26161=ORIENTED_EDGE('',*,*,#18880,.F.);
#26162=ORIENTED_EDGE('',*,*,#18877,.F.);
#26163=ORIENTED_EDGE('',*,*,#18867,.T.);
#26164=ORIENTED_EDGE('',*,*,#18881,.T.);
#26165=ORIENTED_EDGE('',*,*,#18882,.F.);
#26166=ORIENTED_EDGE('',*,*,#18879,.F.);
#26167=ORIENTED_EDGE('',*,*,#18866,.T.);
#26168=ORIENTED_EDGE('',*,*,#18883,.T.);
#26169=ORIENTED_EDGE('',*,*,#18884,.F.);
#26170=ORIENTED_EDGE('',*,*,#18881,.F.);
#26171=ORIENTED_EDGE('',*,*,#18865,.T.);
#26172=ORIENTED_EDGE('',*,*,#18885,.T.);
#26173=ORIENTED_EDGE('',*,*,#18886,.F.);
#26174=ORIENTED_EDGE('',*,*,#18883,.F.);
#26175=ORIENTED_EDGE('',*,*,#18887,.F.);
#26176=ORIENTED_EDGE('',*,*,#18864,.F.);
#26177=ORIENTED_EDGE('',*,*,#18888,.F.);
#26178=ORIENTED_EDGE('',*,*,#18889,.F.);
#26179=ORIENTED_EDGE('',*,*,#18890,.F.);
#26180=ORIENTED_EDGE('',*,*,#18891,.T.);
#26181=ORIENTED_EDGE('',*,*,#18892,.T.);
#26182=ORIENTED_EDGE('',*,*,#18893,.F.);
#26183=ORIENTED_EDGE('',*,*,#18894,.T.);
#26184=ORIENTED_EDGE('',*,*,#18895,.T.);
#26185=ORIENTED_EDGE('',*,*,#18896,.T.);
#26186=ORIENTED_EDGE('',*,*,#18873,.T.);
#26187=ORIENTED_EDGE('',*,*,#18897,.T.);
#26188=ORIENTED_EDGE('',*,*,#18888,.T.);
#26189=ORIENTED_EDGE('',*,*,#18874,.T.);
#26190=ORIENTED_EDGE('',*,*,#18896,.F.);
#26191=ORIENTED_EDGE('',*,*,#18898,.F.);
#26192=ORIENTED_EDGE('',*,*,#18897,.F.);
#26193=ORIENTED_EDGE('',*,*,#18876,.T.);
#26194=ORIENTED_EDGE('',*,*,#18899,.T.);
#26195=ORIENTED_EDGE('',*,*,#18900,.T.);
#26196=ORIENTED_EDGE('',*,*,#18901,.T.);
#26197=ORIENTED_EDGE('',*,*,#18899,.F.);
#26198=ORIENTED_EDGE('',*,*,#18878,.T.);
#26199=ORIENTED_EDGE('',*,*,#18902,.F.);
#26200=ORIENTED_EDGE('',*,*,#18903,.T.);
#26201=ORIENTED_EDGE('',*,*,#18902,.T.);
#26202=ORIENTED_EDGE('',*,*,#18880,.T.);
#26203=ORIENTED_EDGE('',*,*,#18904,.F.);
#26204=ORIENTED_EDGE('',*,*,#18905,.T.);
#26205=ORIENTED_EDGE('',*,*,#18904,.T.);
#26206=ORIENTED_EDGE('',*,*,#18882,.T.);
#26207=ORIENTED_EDGE('',*,*,#18906,.F.);
#26208=ORIENTED_EDGE('',*,*,#18907,.T.);
#26209=ORIENTED_EDGE('',*,*,#18906,.T.);
#26210=ORIENTED_EDGE('',*,*,#18884,.T.);
#26211=ORIENTED_EDGE('',*,*,#18908,.F.);
#26212=ORIENTED_EDGE('',*,*,#18887,.T.);
#26213=ORIENTED_EDGE('',*,*,#18909,.T.);
#26214=ORIENTED_EDGE('',*,*,#18910,.F.);
#26215=ORIENTED_EDGE('',*,*,#18885,.F.);
#26216=ORIENTED_EDGE('',*,*,#18908,.T.);
#26217=ORIENTED_EDGE('',*,*,#18886,.T.);
#26218=ORIENTED_EDGE('',*,*,#18910,.T.);
#26219=ORIENTED_EDGE('',*,*,#18911,.T.);
#26220=ORIENTED_EDGE('',*,*,#18912,.T.);
#26221=ORIENTED_EDGE('',*,*,#18913,.T.);
#26222=ORIENTED_EDGE('',*,*,#18914,.F.);
#26223=ORIENTED_EDGE('',*,*,#18915,.T.);
#26224=ORIENTED_EDGE('',*,*,#18890,.T.);
#26225=ORIENTED_EDGE('',*,*,#18916,.T.);
#26226=ORIENTED_EDGE('',*,*,#18917,.F.);
#26227=ORIENTED_EDGE('',*,*,#18918,.F.);
#26228=ORIENTED_EDGE('',*,*,#18889,.T.);
#26229=ORIENTED_EDGE('',*,*,#18898,.T.);
#26230=ORIENTED_EDGE('',*,*,#18919,.F.);
#26231=ORIENTED_EDGE('',*,*,#18916,.F.);
#26232=ORIENTED_EDGE('',*,*,#18920,.T.);
#26233=ORIENTED_EDGE('',*,*,#18891,.F.);
#26234=ORIENTED_EDGE('',*,*,#18921,.F.);
#26235=ORIENTED_EDGE('',*,*,#18922,.T.);
#26236=ORIENTED_EDGE('',*,*,#18923,.T.);
#26237=ORIENTED_EDGE('',*,*,#18892,.F.);
#26238=ORIENTED_EDGE('',*,*,#18924,.F.);
#26239=ORIENTED_EDGE('',*,*,#18893,.T.);
#26240=ORIENTED_EDGE('',*,*,#18925,.T.);
#26241=ORIENTED_EDGE('',*,*,#18926,.F.);
#26242=ORIENTED_EDGE('',*,*,#18927,.T.);
#26243=ORIENTED_EDGE('',*,*,#18928,.T.);
#26244=ORIENTED_EDGE('',*,*,#18929,.F.);
#26245=ORIENTED_EDGE('',*,*,#18894,.F.);
#26246=ORIENTED_EDGE('',*,*,#18930,.T.);
#26247=ORIENTED_EDGE('',*,*,#18931,.T.);
#26248=ORIENTED_EDGE('',*,*,#18919,.T.);
#26249=ORIENTED_EDGE('',*,*,#18895,.F.);
#26250=ORIENTED_EDGE('',*,*,#18932,.T.);
#26251=ORIENTED_EDGE('',*,*,#18933,.T.);
#26252=ORIENTED_EDGE('',*,*,#18927,.F.);
#26253=ORIENTED_EDGE('',*,*,#18900,.F.);
#26254=ORIENTED_EDGE('',*,*,#18934,.T.);
#26255=ORIENTED_EDGE('',*,*,#18935,.T.);
#26256=ORIENTED_EDGE('',*,*,#18932,.F.);
#26257=ORIENTED_EDGE('',*,*,#18901,.F.);
#26258=ORIENTED_EDGE('',*,*,#18936,.T.);
#26259=ORIENTED_EDGE('',*,*,#18937,.T.);
#26260=ORIENTED_EDGE('',*,*,#18934,.F.);
#26261=ORIENTED_EDGE('',*,*,#18903,.F.);
#26262=ORIENTED_EDGE('',*,*,#18938,.T.);
#26263=ORIENTED_EDGE('',*,*,#18939,.T.);
#26264=ORIENTED_EDGE('',*,*,#18936,.F.);
#26265=ORIENTED_EDGE('',*,*,#18905,.F.);
#26266=ORIENTED_EDGE('',*,*,#18940,.T.);
#26267=ORIENTED_EDGE('',*,*,#18941,.T.);
#26268=ORIENTED_EDGE('',*,*,#18938,.F.);
#26269=ORIENTED_EDGE('',*,*,#18907,.F.);
#26270=ORIENTED_EDGE('',*,*,#18926,.T.);
#26271=ORIENTED_EDGE('',*,*,#18942,.T.);
#26272=ORIENTED_EDGE('',*,*,#18911,.F.);
#26273=ORIENTED_EDGE('',*,*,#18909,.F.);
#26274=ORIENTED_EDGE('',*,*,#18943,.T.);
#26275=ORIENTED_EDGE('',*,*,#18912,.F.);
#26276=ORIENTED_EDGE('',*,*,#18942,.F.);
#26277=ORIENTED_EDGE('',*,*,#18944,.T.);
#26278=ORIENTED_EDGE('',*,*,#18945,.T.);
#26279=ORIENTED_EDGE('',*,*,#18946,.T.);
#26280=ORIENTED_EDGE('',*,*,#18913,.F.);
#26281=ORIENTED_EDGE('',*,*,#18947,.F.);
#26282=ORIENTED_EDGE('',*,*,#18948,.T.);
#26283=ORIENTED_EDGE('',*,*,#18914,.T.);
#26284=ORIENTED_EDGE('',*,*,#18949,.T.);
#26285=ORIENTED_EDGE('',*,*,#18950,.F.);
#26286=ORIENTED_EDGE('',*,*,#18951,.T.);
#26287=ORIENTED_EDGE('',*,*,#18952,.T.);
#26288=ORIENTED_EDGE('',*,*,#18940,.F.);
#26289=ORIENTED_EDGE('',*,*,#18915,.F.);
#26290=ORIENTED_EDGE('',*,*,#18953,.T.);
#26291=ORIENTED_EDGE('',*,*,#18954,.T.);
#26292=ORIENTED_EDGE('',*,*,#18955,.T.);
#26293=ORIENTED_EDGE('',*,*,#18956,.T.);
#26294=ORIENTED_EDGE('',*,*,#18957,.T.);
#26295=ORIENTED_EDGE('',*,*,#18917,.T.);
#26296=ORIENTED_EDGE('',*,*,#18931,.F.);
#26297=ORIENTED_EDGE('',*,*,#18921,.T.);
#26298=ORIENTED_EDGE('',*,*,#18918,.T.);
#26299=ORIENTED_EDGE('',*,*,#18957,.F.);
#26300=ORIENTED_EDGE('',*,*,#18958,.F.);
#26301=ORIENTED_EDGE('',*,*,#18924,.T.);
#26302=ORIENTED_EDGE('',*,*,#18920,.F.);
#26303=ORIENTED_EDGE('',*,*,#18959,.F.);
#26304=ORIENTED_EDGE('',*,*,#18960,.T.);
#26305=ORIENTED_EDGE('',*,*,#18961,.T.);
#26306=ORIENTED_EDGE('',*,*,#18962,.T.);
#26307=ORIENTED_EDGE('',*,*,#18922,.F.);
#26308=ORIENTED_EDGE('',*,*,#18963,.F.);
#26309=ORIENTED_EDGE('',*,*,#18944,.F.);
#26310=ORIENTED_EDGE('',*,*,#18925,.F.);
#26311=ORIENTED_EDGE('',*,*,#18923,.F.);
#26312=ORIENTED_EDGE('',*,*,#18964,.T.);
#26313=ORIENTED_EDGE('',*,*,#18929,.T.);
#26314=ORIENTED_EDGE('',*,*,#18965,.T.);
#26315=ORIENTED_EDGE('',*,*,#18966,.F.);
#26316=ORIENTED_EDGE('',*,*,#18930,.F.);
#26317=ORIENTED_EDGE('',*,*,#18967,.F.);
#26318=ORIENTED_EDGE('',*,*,#18968,.F.);
#26319=ORIENTED_EDGE('',*,*,#18969,.F.);
#26320=ORIENTED_EDGE('',*,*,#18970,.F.);
#26321=ORIENTED_EDGE('',*,*,#18971,.F.);
#26322=ORIENTED_EDGE('',*,*,#18972,.F.);
#26323=ORIENTED_EDGE('',*,*,#18973,.F.);
#26324=ORIENTED_EDGE('',*,*,#18974,.F.);
#26325=ORIENTED_EDGE('',*,*,#18975,.F.);
#26326=ORIENTED_EDGE('',*,*,#18976,.F.);
#26327=ORIENTED_EDGE('',*,*,#18977,.F.);
#26328=ORIENTED_EDGE('',*,*,#18978,.F.);
#26329=ORIENTED_EDGE('',*,*,#18979,.F.);
#26330=ORIENTED_EDGE('',*,*,#18980,.F.);
#26331=ORIENTED_EDGE('',*,*,#18981,.F.);
#26332=ORIENTED_EDGE('',*,*,#18982,.F.);
#26333=ORIENTED_EDGE('',*,*,#18983,.F.);
#26334=ORIENTED_EDGE('',*,*,#18984,.F.);
#26335=ORIENTED_EDGE('',*,*,#18985,.F.);
#26336=ORIENTED_EDGE('',*,*,#18986,.F.);
#26337=ORIENTED_EDGE('',*,*,#18987,.F.);
#26338=ORIENTED_EDGE('',*,*,#18988,.F.);
#26339=ORIENTED_EDGE('',*,*,#18989,.F.);
#26340=ORIENTED_EDGE('',*,*,#18990,.F.);
#26341=ORIENTED_EDGE('',*,*,#18965,.F.);
#26342=ORIENTED_EDGE('',*,*,#18928,.F.);
#26343=ORIENTED_EDGE('',*,*,#18933,.F.);
#26344=ORIENTED_EDGE('',*,*,#18935,.F.);
#26345=ORIENTED_EDGE('',*,*,#18937,.F.);
#26346=ORIENTED_EDGE('',*,*,#18939,.F.);
#26347=ORIENTED_EDGE('',*,*,#18941,.F.);
#26348=ORIENTED_EDGE('',*,*,#18952,.F.);
#26349=ORIENTED_EDGE('',*,*,#18991,.F.);
#26350=ORIENTED_EDGE('',*,*,#18992,.F.);
#26351=ORIENTED_EDGE('',*,*,#18993,.F.);
#26352=ORIENTED_EDGE('',*,*,#18994,.F.);
#26353=ORIENTED_EDGE('',*,*,#18995,.F.);
#26354=ORIENTED_EDGE('',*,*,#18996,.F.);
#26355=ORIENTED_EDGE('',*,*,#18997,.F.);
#26356=ORIENTED_EDGE('',*,*,#18998,.F.);
#26357=ORIENTED_EDGE('',*,*,#18999,.F.);
#26358=ORIENTED_EDGE('',*,*,#18947,.T.);
#26359=ORIENTED_EDGE('',*,*,#18943,.F.);
#26360=ORIENTED_EDGE('',*,*,#19000,.F.);
#26361=ORIENTED_EDGE('',*,*,#18842,.T.);
#26362=ORIENTED_EDGE('',*,*,#19001,.T.);
#26363=ORIENTED_EDGE('',*,*,#19002,.F.);
#26364=ORIENTED_EDGE('',*,*,#19003,.F.);
#26365=ORIENTED_EDGE('',*,*,#19004,.F.);
#26366=ORIENTED_EDGE('',*,*,#19005,.F.);
#26367=ORIENTED_EDGE('',*,*,#19006,.F.);
#26368=ORIENTED_EDGE('',*,*,#18945,.F.);
#26369=ORIENTED_EDGE('',*,*,#19007,.F.);
#26370=ORIENTED_EDGE('',*,*,#18961,.F.);
#26371=ORIENTED_EDGE('',*,*,#19008,.F.);
#26372=ORIENTED_EDGE('',*,*,#19009,.F.);
#26373=ORIENTED_EDGE('',*,*,#19010,.F.);
#26374=ORIENTED_EDGE('',*,*,#19011,.F.);
#26375=ORIENTED_EDGE('',*,*,#19002,.T.);
#26376=ORIENTED_EDGE('',*,*,#19012,.T.);
#26377=ORIENTED_EDGE('',*,*,#19006,.T.);
#26378=ORIENTED_EDGE('',*,*,#19013,.T.);
#26379=ORIENTED_EDGE('',*,*,#18949,.F.);
#26380=ORIENTED_EDGE('',*,*,#18946,.F.);
#26381=ORIENTED_EDGE('',*,*,#18950,.T.);
#26382=ORIENTED_EDGE('',*,*,#19014,.T.);
#26383=ORIENTED_EDGE('',*,*,#19015,.F.);
#26384=ORIENTED_EDGE('',*,*,#19016,.T.);
#26385=ORIENTED_EDGE('',*,*,#19017,.T.);
#26386=ORIENTED_EDGE('',*,*,#18991,.T.);
#26387=ORIENTED_EDGE('',*,*,#18951,.F.);
#26388=ORIENTED_EDGE('',*,*,#18948,.F.);
#26389=ORIENTED_EDGE('',*,*,#19009,.T.);
#26390=ORIENTED_EDGE('',*,*,#19018,.T.);
#26391=ORIENTED_EDGE('',*,*,#18955,.F.);
#26392=ORIENTED_EDGE('',*,*,#19019,.F.);
#26393=ORIENTED_EDGE('',*,*,#19020,.T.);
#26394=ORIENTED_EDGE('',*,*,#18959,.T.);
#26395=ORIENTED_EDGE('',*,*,#18958,.T.);
#26396=ORIENTED_EDGE('',*,*,#18956,.F.);
#26397=ORIENTED_EDGE('',*,*,#19021,.T.);
#26398=ORIENTED_EDGE('',*,*,#19022,.T.);
#26399=ORIENTED_EDGE('',*,*,#19023,.T.);
#26400=ORIENTED_EDGE('',*,*,#18954,.F.);
#26401=ORIENTED_EDGE('',*,*,#18966,.T.);
#26402=ORIENTED_EDGE('',*,*,#18990,.T.);
#26403=ORIENTED_EDGE('',*,*,#19024,.F.);
#26404=ORIENTED_EDGE('',*,*,#18953,.F.);
#26405=ORIENTED_EDGE('',*,*,#19008,.T.);
#26406=ORIENTED_EDGE('',*,*,#18963,.T.);
#26407=ORIENTED_EDGE('',*,*,#18960,.F.);
#26408=ORIENTED_EDGE('',*,*,#19025,.F.);
#26409=ORIENTED_EDGE('',*,*,#19007,.T.);
#26410=ORIENTED_EDGE('',*,*,#19000,.T.);
#26411=ORIENTED_EDGE('',*,*,#18964,.F.);
#26412=ORIENTED_EDGE('',*,*,#18962,.F.);
#26413=ORIENTED_EDGE('',*,*,#18999,.T.);
#26414=ORIENTED_EDGE('',*,*,#19026,.F.);
#26415=ORIENTED_EDGE('',*,*,#19027,.F.);
#26416=ORIENTED_EDGE('',*,*,#19028,.F.);
#26417=ORIENTED_EDGE('',*,*,#19026,.T.);
#26418=ORIENTED_EDGE('',*,*,#18998,.T.);
#26419=ORIENTED_EDGE('',*,*,#19029,.F.);
#26420=ORIENTED_EDGE('',*,*,#19030,.F.);
#26421=ORIENTED_EDGE('',*,*,#19029,.T.);
#26422=ORIENTED_EDGE('',*,*,#18997,.T.);
#26423=ORIENTED_EDGE('',*,*,#19031,.F.);
#26424=ORIENTED_EDGE('',*,*,#19032,.F.);
#26425=ORIENTED_EDGE('',*,*,#19031,.T.);
#26426=ORIENTED_EDGE('',*,*,#18996,.T.);
#26427=ORIENTED_EDGE('',*,*,#19033,.F.);
#26428=ORIENTED_EDGE('',*,*,#19034,.F.);
#26429=ORIENTED_EDGE('',*,*,#19033,.T.);
#26430=ORIENTED_EDGE('',*,*,#18995,.T.);
#26431=ORIENTED_EDGE('',*,*,#19035,.F.);
#26432=ORIENTED_EDGE('',*,*,#19036,.F.);
#26433=ORIENTED_EDGE('',*,*,#19037,.T.);
#26434=ORIENTED_EDGE('',*,*,#18994,.T.);
#26435=ORIENTED_EDGE('',*,*,#19038,.F.);
#26436=ORIENTED_EDGE('',*,*,#19039,.F.);
#26437=ORIENTED_EDGE('',*,*,#19038,.T.);
#26438=ORIENTED_EDGE('',*,*,#18993,.T.);
#26439=ORIENTED_EDGE('',*,*,#19040,.F.);
#26440=ORIENTED_EDGE('',*,*,#19041,.F.);
#26441=ORIENTED_EDGE('',*,*,#19040,.T.);
#26442=ORIENTED_EDGE('',*,*,#18992,.T.);
#26443=ORIENTED_EDGE('',*,*,#19017,.F.);
#26444=ORIENTED_EDGE('',*,*,#19016,.F.);
#26445=ORIENTED_EDGE('',*,*,#19024,.T.);
#26446=ORIENTED_EDGE('',*,*,#18989,.T.);
#26447=ORIENTED_EDGE('',*,*,#19042,.F.);
#26448=ORIENTED_EDGE('',*,*,#19021,.F.);
#26449=ORIENTED_EDGE('',*,*,#19042,.T.);
#26450=ORIENTED_EDGE('',*,*,#18988,.T.);
#26451=ORIENTED_EDGE('',*,*,#19043,.F.);
#26452=ORIENTED_EDGE('',*,*,#19044,.F.);
#26453=ORIENTED_EDGE('',*,*,#19043,.T.);
#26454=ORIENTED_EDGE('',*,*,#18987,.T.);
#26455=ORIENTED_EDGE('',*,*,#19045,.F.);
#26456=ORIENTED_EDGE('',*,*,#19046,.F.);
#26457=ORIENTED_EDGE('',*,*,#19045,.T.);
#26458=ORIENTED_EDGE('',*,*,#18986,.T.);
#26459=ORIENTED_EDGE('',*,*,#19047,.F.);
#26460=ORIENTED_EDGE('',*,*,#19048,.F.);
#26461=ORIENTED_EDGE('',*,*,#19049,.T.);
#26462=ORIENTED_EDGE('',*,*,#18985,.T.);
#26463=ORIENTED_EDGE('',*,*,#19050,.F.);
#26464=ORIENTED_EDGE('',*,*,#19051,.F.);
#26465=ORIENTED_EDGE('',*,*,#19050,.T.);
#26466=ORIENTED_EDGE('',*,*,#18984,.T.);
#26467=ORIENTED_EDGE('',*,*,#19052,.F.);
#26468=ORIENTED_EDGE('',*,*,#19053,.F.);
#26469=ORIENTED_EDGE('',*,*,#19052,.T.);
#26470=ORIENTED_EDGE('',*,*,#18983,.T.);
#26471=ORIENTED_EDGE('',*,*,#19054,.F.);
#26472=ORIENTED_EDGE('',*,*,#19055,.F.);
#26473=ORIENTED_EDGE('',*,*,#19054,.T.);
#26474=ORIENTED_EDGE('',*,*,#18982,.T.);
#26475=ORIENTED_EDGE('',*,*,#19056,.F.);
#26476=ORIENTED_EDGE('',*,*,#19057,.F.);
#26477=ORIENTED_EDGE('',*,*,#19056,.T.);
#26478=ORIENTED_EDGE('',*,*,#18981,.T.);
#26479=ORIENTED_EDGE('',*,*,#19058,.F.);
#26480=ORIENTED_EDGE('',*,*,#19059,.F.);
#26481=ORIENTED_EDGE('',*,*,#19058,.T.);
#26482=ORIENTED_EDGE('',*,*,#18980,.T.);
#26483=ORIENTED_EDGE('',*,*,#19060,.F.);
#26484=ORIENTED_EDGE('',*,*,#19061,.F.);
#26485=ORIENTED_EDGE('',*,*,#19060,.T.);
#26486=ORIENTED_EDGE('',*,*,#18979,.T.);
#26487=ORIENTED_EDGE('',*,*,#19062,.F.);
#26488=ORIENTED_EDGE('',*,*,#19063,.F.);
#26489=ORIENTED_EDGE('',*,*,#19062,.T.);
#26490=ORIENTED_EDGE('',*,*,#18978,.T.);
#26491=ORIENTED_EDGE('',*,*,#19064,.F.);
#26492=ORIENTED_EDGE('',*,*,#19065,.F.);
#26493=ORIENTED_EDGE('',*,*,#19064,.T.);
#26494=ORIENTED_EDGE('',*,*,#18977,.T.);
#26495=ORIENTED_EDGE('',*,*,#19066,.F.);
#26496=ORIENTED_EDGE('',*,*,#19067,.F.);
#26497=ORIENTED_EDGE('',*,*,#19066,.T.);
#26498=ORIENTED_EDGE('',*,*,#18976,.T.);
#26499=ORIENTED_EDGE('',*,*,#19068,.F.);
#26500=ORIENTED_EDGE('',*,*,#19069,.F.);
#26501=ORIENTED_EDGE('',*,*,#19068,.T.);
#26502=ORIENTED_EDGE('',*,*,#18975,.T.);
#26503=ORIENTED_EDGE('',*,*,#19070,.F.);
#26504=ORIENTED_EDGE('',*,*,#19071,.F.);
#26505=ORIENTED_EDGE('',*,*,#19072,.T.);
#26506=ORIENTED_EDGE('',*,*,#18974,.T.);
#26507=ORIENTED_EDGE('',*,*,#19073,.F.);
#26508=ORIENTED_EDGE('',*,*,#19074,.F.);
#26509=ORIENTED_EDGE('',*,*,#19075,.T.);
#26510=ORIENTED_EDGE('',*,*,#18973,.T.);
#26511=ORIENTED_EDGE('',*,*,#19076,.F.);
#26512=ORIENTED_EDGE('',*,*,#19077,.F.);
#26513=ORIENTED_EDGE('',*,*,#19076,.T.);
#26514=ORIENTED_EDGE('',*,*,#18972,.T.);
#26515=ORIENTED_EDGE('',*,*,#19078,.F.);
#26516=ORIENTED_EDGE('',*,*,#19079,.F.);
#26517=ORIENTED_EDGE('',*,*,#19078,.T.);
#26518=ORIENTED_EDGE('',*,*,#18971,.T.);
#26519=ORIENTED_EDGE('',*,*,#19080,.F.);
#26520=ORIENTED_EDGE('',*,*,#19081,.F.);
#26521=ORIENTED_EDGE('',*,*,#19082,.T.);
#26522=ORIENTED_EDGE('',*,*,#18970,.T.);
#26523=ORIENTED_EDGE('',*,*,#19083,.F.);
#26524=ORIENTED_EDGE('',*,*,#19084,.F.);
#26525=ORIENTED_EDGE('',*,*,#19085,.T.);
#26526=ORIENTED_EDGE('',*,*,#18969,.T.);
#26527=ORIENTED_EDGE('',*,*,#19086,.F.);
#26528=ORIENTED_EDGE('',*,*,#19087,.F.);
#26529=ORIENTED_EDGE('',*,*,#19086,.T.);
#26530=ORIENTED_EDGE('',*,*,#18968,.T.);
#26531=ORIENTED_EDGE('',*,*,#19088,.F.);
#26532=ORIENTED_EDGE('',*,*,#19089,.F.);
#26533=ORIENTED_EDGE('',*,*,#19090,.F.);
#26534=ORIENTED_EDGE('',*,*,#19088,.T.);
#26535=ORIENTED_EDGE('',*,*,#18967,.T.);
#26536=ORIENTED_EDGE('',*,*,#19028,.T.);
#26537=ORIENTED_EDGE('',*,*,#19091,.T.);
#26538=ORIENTED_EDGE('',*,*,#19092,.T.);
#26539=ORIENTED_EDGE('',*,*,#19093,.T.);
#26540=ORIENTED_EDGE('',*,*,#19012,.F.);
#26541=ORIENTED_EDGE('',*,*,#19093,.F.);
#26542=ORIENTED_EDGE('',*,*,#19010,.T.);
#26543=ORIENTED_EDGE('',*,*,#19019,.T.);
#26544=ORIENTED_EDGE('',*,*,#19023,.F.);
#26545=ORIENTED_EDGE('',*,*,#19094,.F.);
#26546=ORIENTED_EDGE('',*,*,#18846,.T.);
#26547=ORIENTED_EDGE('',*,*,#19095,.T.);
#26548=ORIENTED_EDGE('',*,*,#19096,.F.);
#26549=ORIENTED_EDGE('',*,*,#19097,.F.);
#26550=ORIENTED_EDGE('',*,*,#19096,.T.);
#26551=ORIENTED_EDGE('',*,*,#19098,.F.);
#26552=ORIENTED_EDGE('',*,*,#19051,.T.);
#26553=ORIENTED_EDGE('',*,*,#19099,.T.);
#26554=ORIENTED_EDGE('',*,*,#18849,.T.);
#26555=ORIENTED_EDGE('',*,*,#19100,.T.);
#26556=ORIENTED_EDGE('',*,*,#19101,.F.);
#26557=ORIENTED_EDGE('',*,*,#19102,.F.);
#26558=ORIENTED_EDGE('',*,*,#19101,.T.);
#26559=ORIENTED_EDGE('',*,*,#19103,.T.);
#26560=ORIENTED_EDGE('',*,*,#19104,.F.);
#26561=ORIENTED_EDGE('',*,*,#19105,.T.);
#26562=ORIENTED_EDGE('',*,*,#18839,.T.);
#26563=ORIENTED_EDGE('',*,*,#19106,.T.);
#26564=ORIENTED_EDGE('',*,*,#19107,.F.);
#26565=ORIENTED_EDGE('',*,*,#19108,.F.);
#26566=ORIENTED_EDGE('',*,*,#19107,.T.);
#26567=ORIENTED_EDGE('',*,*,#19109,.F.);
#26568=ORIENTED_EDGE('',*,*,#19036,.T.);
#26569=ORIENTED_EDGE('',*,*,#19110,.T.);
#26570=ORIENTED_EDGE('',*,*,#18856,.T.);
#26571=ORIENTED_EDGE('',*,*,#19111,.T.);
#26572=ORIENTED_EDGE('',*,*,#19112,.F.);
#26573=ORIENTED_EDGE('',*,*,#19113,.F.);
#26574=ORIENTED_EDGE('',*,*,#19112,.T.);
#26575=ORIENTED_EDGE('',*,*,#19114,.F.);
#26576=ORIENTED_EDGE('',*,*,#19115,.F.);
#26577=ORIENTED_EDGE('',*,*,#19116,.F.);
#26578=ORIENTED_EDGE('',*,*,#19003,.T.);
#26579=ORIENTED_EDGE('',*,*,#19117,.F.);
#26580=ORIENTED_EDGE('',*,*,#19118,.F.);
#26581=ORIENTED_EDGE('',*,*,#19117,.T.);
#26582=ORIENTED_EDGE('',*,*,#19011,.T.);
#26583=ORIENTED_EDGE('',*,*,#19094,.T.);
#26584=ORIENTED_EDGE('',*,*,#19119,.F.);
#26585=ORIENTED_EDGE('',*,*,#19120,.T.);
#26586=ORIENTED_EDGE('',*,*,#19121,.F.);
#26587=ORIENTED_EDGE('',*,*,#19001,.F.);
#26588=ORIENTED_EDGE('',*,*,#19121,.T.);
#26589=ORIENTED_EDGE('',*,*,#19122,.F.);
#26590=ORIENTED_EDGE('',*,*,#19123,.F.);
#26591=ORIENTED_EDGE('',*,*,#19004,.T.);
#26592=ORIENTED_EDGE('',*,*,#19005,.T.);
#26593=ORIENTED_EDGE('',*,*,#19123,.T.);
#26594=ORIENTED_EDGE('',*,*,#19014,.F.);
#26595=ORIENTED_EDGE('',*,*,#19013,.F.);
#26596=ORIENTED_EDGE('',*,*,#18841,.T.);
#26597=ORIENTED_EDGE('',*,*,#18808,.T.);
#26598=ORIENTED_EDGE('',*,*,#18807,.T.);
#26599=ORIENTED_EDGE('',*,*,#19124,.F.);
#26600=ORIENTED_EDGE('',*,*,#19120,.F.);
#26601=ORIENTED_EDGE('',*,*,#19125,.F.);
#26602=ORIENTED_EDGE('',*,*,#19041,.T.);
#26603=ORIENTED_EDGE('',*,*,#19015,.T.);
#26604=ORIENTED_EDGE('',*,*,#19122,.T.);
#26605=ORIENTED_EDGE('',*,*,#19124,.T.);
#26606=ORIENTED_EDGE('',*,*,#19025,.T.);
#26607=ORIENTED_EDGE('',*,*,#19020,.F.);
#26608=ORIENTED_EDGE('',*,*,#19018,.F.);
#26609=ORIENTED_EDGE('',*,*,#18843,.T.);
#26610=ORIENTED_EDGE('',*,*,#19118,.T.);
#26611=ORIENTED_EDGE('',*,*,#19126,.F.);
#26612=ORIENTED_EDGE('',*,*,#19127,.F.);
#26613=ORIENTED_EDGE('',*,*,#19126,.T.);
#26614=ORIENTED_EDGE('',*,*,#19119,.T.);
#26615=ORIENTED_EDGE('',*,*,#19022,.F.);
#26616=ORIENTED_EDGE('',*,*,#19044,.T.);
#26617=ORIENTED_EDGE('',*,*,#19128,.T.);
#26618=ORIENTED_EDGE('',*,*,#19027,.T.);
#26619=ORIENTED_EDGE('',*,*,#19129,.T.);
#26620=ORIENTED_EDGE('',*,*,#19130,.F.);
#26621=ORIENTED_EDGE('',*,*,#19131,.F.);
#26622=ORIENTED_EDGE('',*,*,#19132,.T.);
#26623=ORIENTED_EDGE('',*,*,#19133,.F.);
#26624=ORIENTED_EDGE('',*,*,#19129,.F.);
#26625=ORIENTED_EDGE('',*,*,#19030,.T.);
#26626=ORIENTED_EDGE('',*,*,#18837,.T.);
#26627=ORIENTED_EDGE('',*,*,#19134,.T.);
#26628=ORIENTED_EDGE('',*,*,#19135,.F.);
#26629=ORIENTED_EDGE('',*,*,#19136,.F.);
#26630=ORIENTED_EDGE('',*,*,#19135,.T.);
#26631=ORIENTED_EDGE('',*,*,#19137,.T.);
#26632=ORIENTED_EDGE('',*,*,#19138,.F.);
#26633=ORIENTED_EDGE('',*,*,#19132,.F.);
#26634=ORIENTED_EDGE('',*,*,#19032,.T.);
#26635=ORIENTED_EDGE('',*,*,#19139,.T.);
#26636=ORIENTED_EDGE('',*,*,#18857,.T.);
#26637=ORIENTED_EDGE('',*,*,#19113,.T.);
#26638=ORIENTED_EDGE('',*,*,#19140,.F.);
#26639=ORIENTED_EDGE('',*,*,#19134,.F.);
#26640=ORIENTED_EDGE('',*,*,#19116,.T.);
#26641=ORIENTED_EDGE('',*,*,#19141,.F.);
#26642=ORIENTED_EDGE('',*,*,#19137,.F.);
#26643=ORIENTED_EDGE('',*,*,#19140,.T.);
#26644=ORIENTED_EDGE('',*,*,#18838,.T.);
#26645=ORIENTED_EDGE('',*,*,#19136,.T.);
#26646=ORIENTED_EDGE('',*,*,#19142,.F.);
#26647=ORIENTED_EDGE('',*,*,#19106,.F.);
#26648=ORIENTED_EDGE('',*,*,#19139,.F.);
#26649=ORIENTED_EDGE('',*,*,#19034,.T.);
#26650=ORIENTED_EDGE('',*,*,#19109,.T.);
#26651=ORIENTED_EDGE('',*,*,#19142,.T.);
#26652=ORIENTED_EDGE('',*,*,#19035,.T.);
#26653=ORIENTED_EDGE('',*,*,#19037,.F.);
#26654=ORIENTED_EDGE('',*,*,#19143,.F.);
#26655=ORIENTED_EDGE('',*,*,#19144,.F.);
#26656=ORIENTED_EDGE('',*,*,#19039,.T.);
#26657=ORIENTED_EDGE('',*,*,#19125,.T.);
#26658=ORIENTED_EDGE('',*,*,#18806,.T.);
#26659=ORIENTED_EDGE('',*,*,#18844,.T.);
#26660=ORIENTED_EDGE('',*,*,#19127,.T.);
#26661=ORIENTED_EDGE('',*,*,#19145,.F.);
#26662=ORIENTED_EDGE('',*,*,#18799,.F.);
#26663=ORIENTED_EDGE('',*,*,#18798,.F.);
#26664=ORIENTED_EDGE('',*,*,#19128,.F.);
#26665=ORIENTED_EDGE('',*,*,#19046,.T.);
#26666=ORIENTED_EDGE('',*,*,#19146,.T.);
#26667=ORIENTED_EDGE('',*,*,#19145,.T.);
#26668=ORIENTED_EDGE('',*,*,#19146,.F.);
#26669=ORIENTED_EDGE('',*,*,#19048,.T.);
#26670=ORIENTED_EDGE('',*,*,#19147,.T.);
#26671=ORIENTED_EDGE('',*,*,#18800,.T.);
#26672=ORIENTED_EDGE('',*,*,#19047,.T.);
#26673=ORIENTED_EDGE('',*,*,#19049,.F.);
#26674=ORIENTED_EDGE('',*,*,#19148,.F.);
#26675=ORIENTED_EDGE('',*,*,#18847,.T.);
#26676=ORIENTED_EDGE('',*,*,#19097,.T.);
#26677=ORIENTED_EDGE('',*,*,#19149,.F.);
#26678=ORIENTED_EDGE('',*,*,#18793,.F.);
#26679=ORIENTED_EDGE('',*,*,#18792,.F.);
#26680=ORIENTED_EDGE('',*,*,#19099,.F.);
#26681=ORIENTED_EDGE('',*,*,#19053,.T.);
#26682=ORIENTED_EDGE('',*,*,#19150,.T.);
#26683=ORIENTED_EDGE('',*,*,#19149,.T.);
#26684=ORIENTED_EDGE('',*,*,#18848,.T.);
#26685=ORIENTED_EDGE('',*,*,#18796,.T.);
#26686=ORIENTED_EDGE('',*,*,#18795,.T.);
#26687=ORIENTED_EDGE('',*,*,#19151,.F.);
#26688=ORIENTED_EDGE('',*,*,#19100,.F.);
#26689=ORIENTED_EDGE('',*,*,#19152,.T.);
#26690=ORIENTED_EDGE('',*,*,#19153,.F.);
#26691=ORIENTED_EDGE('',*,*,#19103,.F.);
#26692=ORIENTED_EDGE('',*,*,#19151,.T.);
#26693=ORIENTED_EDGE('',*,*,#19150,.F.);
#26694=ORIENTED_EDGE('',*,*,#19055,.T.);
#26695=ORIENTED_EDGE('',*,*,#19154,.T.);
#26696=ORIENTED_EDGE('',*,*,#19155,.F.);
#26697=ORIENTED_EDGE('',*,*,#19152,.F.);
#26698=ORIENTED_EDGE('',*,*,#18794,.T.);
#26699=ORIENTED_EDGE('',*,*,#19156,.T.);
#26700=ORIENTED_EDGE('',*,*,#19157,.F.);
#26701=ORIENTED_EDGE('',*,*,#19154,.F.);
#26702=ORIENTED_EDGE('',*,*,#19057,.T.);
#26703=ORIENTED_EDGE('',*,*,#19158,.T.);
#26704=ORIENTED_EDGE('',*,*,#19159,.F.);
#26705=ORIENTED_EDGE('',*,*,#19156,.F.);
#26706=ORIENTED_EDGE('',*,*,#19059,.T.);
#26707=ORIENTED_EDGE('',*,*,#19160,.T.);
#26708=ORIENTED_EDGE('',*,*,#19161,.F.);
#26709=ORIENTED_EDGE('',*,*,#19158,.F.);
#26710=ORIENTED_EDGE('',*,*,#19061,.T.);
#26711=ORIENTED_EDGE('',*,*,#19162,.F.);
#26712=ORIENTED_EDGE('',*,*,#19163,.F.);
#26713=ORIENTED_EDGE('',*,*,#19160,.F.);
#26714=ORIENTED_EDGE('',*,*,#19063,.T.);
#26715=ORIENTED_EDGE('',*,*,#19065,.T.);
#26716=ORIENTED_EDGE('',*,*,#19164,.F.);
#26717=ORIENTED_EDGE('',*,*,#19165,.F.);
#26718=ORIENTED_EDGE('',*,*,#19162,.T.);
#26719=ORIENTED_EDGE('',*,*,#19166,.F.);
#26720=ORIENTED_EDGE('',*,*,#19167,.F.);
#26721=ORIENTED_EDGE('',*,*,#19164,.T.);
#26722=ORIENTED_EDGE('',*,*,#19067,.T.);
#26723=ORIENTED_EDGE('',*,*,#19069,.T.);
#26724=ORIENTED_EDGE('',*,*,#19168,.F.);
#26725=ORIENTED_EDGE('',*,*,#19169,.F.);
#26726=ORIENTED_EDGE('',*,*,#19166,.T.);
#26727=ORIENTED_EDGE('',*,*,#19170,.T.);
#26728=ORIENTED_EDGE('',*,*,#19171,.F.);
#26729=ORIENTED_EDGE('',*,*,#19168,.T.);
#26730=ORIENTED_EDGE('',*,*,#19071,.T.);
#26731=ORIENTED_EDGE('',*,*,#19070,.T.);
#26732=ORIENTED_EDGE('',*,*,#19072,.F.);
#26733=ORIENTED_EDGE('',*,*,#19172,.F.);
#26734=ORIENTED_EDGE('',*,*,#19173,.T.);
#26735=ORIENTED_EDGE('',*,*,#19174,.F.);
#26736=ORIENTED_EDGE('',*,*,#19175,.F.);
#26737=ORIENTED_EDGE('',*,*,#19074,.T.);
#26738=ORIENTED_EDGE('',*,*,#19073,.T.);
#26739=ORIENTED_EDGE('',*,*,#19075,.F.);
#26740=ORIENTED_EDGE('',*,*,#19176,.F.);
#26741=ORIENTED_EDGE('',*,*,#19177,.F.);
#26742=ORIENTED_EDGE('',*,*,#19178,.F.);
#26743=ORIENTED_EDGE('',*,*,#19179,.F.);
#26744=ORIENTED_EDGE('',*,*,#19077,.T.);
#26745=ORIENTED_EDGE('',*,*,#19079,.T.);
#26746=ORIENTED_EDGE('',*,*,#19180,.F.);
#26747=ORIENTED_EDGE('',*,*,#19181,.F.);
#26748=ORIENTED_EDGE('',*,*,#19177,.T.);
#26749=ORIENTED_EDGE('',*,*,#19182,.T.);
#26750=ORIENTED_EDGE('',*,*,#19183,.F.);
#26751=ORIENTED_EDGE('',*,*,#19180,.T.);
#26752=ORIENTED_EDGE('',*,*,#19081,.T.);
#26753=ORIENTED_EDGE('',*,*,#19080,.T.);
#26754=ORIENTED_EDGE('',*,*,#19082,.F.);
#26755=ORIENTED_EDGE('',*,*,#19184,.F.);
#26756=ORIENTED_EDGE('',*,*,#19185,.T.);
#26757=ORIENTED_EDGE('',*,*,#19186,.F.);
#26758=ORIENTED_EDGE('',*,*,#19187,.F.);
#26759=ORIENTED_EDGE('',*,*,#19084,.T.);
#26760=ORIENTED_EDGE('',*,*,#19083,.T.);
#26761=ORIENTED_EDGE('',*,*,#19085,.F.);
#26762=ORIENTED_EDGE('',*,*,#19188,.F.);
#26763=ORIENTED_EDGE('',*,*,#19087,.T.);
#26764=ORIENTED_EDGE('',*,*,#19189,.F.);
#26765=ORIENTED_EDGE('',*,*,#19190,.F.);
#26766=ORIENTED_EDGE('',*,*,#19191,.F.);
#26767=ORIENTED_EDGE('',*,*,#19089,.T.);
#26768=ORIENTED_EDGE('',*,*,#19192,.F.);
#26769=ORIENTED_EDGE('',*,*,#19193,.F.);
#26770=ORIENTED_EDGE('',*,*,#19189,.T.);
#26771=ORIENTED_EDGE('',*,*,#19131,.T.);
#26772=ORIENTED_EDGE('',*,*,#19194,.F.);
#26773=ORIENTED_EDGE('',*,*,#19192,.T.);
#26774=ORIENTED_EDGE('',*,*,#19090,.T.);
#26775=ORIENTED_EDGE('',*,*,#19195,.T.);
#26776=ORIENTED_EDGE('',*,*,#19196,.T.);
#26777=ORIENTED_EDGE('',*,*,#19091,.F.);
#26778=ORIENTED_EDGE('',*,*,#19092,.F.);
#26779=ORIENTED_EDGE('',*,*,#19196,.F.);
#26780=ORIENTED_EDGE('',*,*,#19104,.T.);
#26781=ORIENTED_EDGE('',*,*,#19197,.T.);
#26782=ORIENTED_EDGE('',*,*,#19198,.F.);
#26783=ORIENTED_EDGE('',*,*,#19199,.F.);
#26784=ORIENTED_EDGE('',*,*,#18850,.T.);
#26785=ORIENTED_EDGE('',*,*,#19102,.T.);
#26786=ORIENTED_EDGE('',*,*,#19200,.F.);
#26787=ORIENTED_EDGE('',*,*,#18790,.F.);
#26788=ORIENTED_EDGE('',*,*,#18789,.F.);
#26789=ORIENTED_EDGE('',*,*,#19105,.F.);
#26790=ORIENTED_EDGE('',*,*,#19201,.F.);
#26791=ORIENTED_EDGE('',*,*,#19202,.T.);
#26792=ORIENTED_EDGE('',*,*,#19200,.T.);
#26793=ORIENTED_EDGE('',*,*,#18853,.T.);
#26794=ORIENTED_EDGE('',*,*,#19203,.T.);
#26795=ORIENTED_EDGE('',*,*,#19204,.F.);
#26796=ORIENTED_EDGE('',*,*,#19205,.F.);
#26797=ORIENTED_EDGE('',*,*,#19204,.T.);
#26798=ORIENTED_EDGE('',*,*,#19206,.T.);
#26799=ORIENTED_EDGE('',*,*,#19207,.T.);
#26800=ORIENTED_EDGE('',*,*,#19208,.T.);
#26801=ORIENTED_EDGE('',*,*,#19209,.T.);
#26802=ORIENTED_EDGE('',*,*,#19210,.T.);
#26803=ORIENTED_EDGE('',*,*,#19211,.T.);
#26804=ORIENTED_EDGE('',*,*,#19212,.T.);
#26805=ORIENTED_EDGE('',*,*,#19213,.T.);
#26806=ORIENTED_EDGE('',*,*,#19214,.T.);
#26807=ORIENTED_EDGE('',*,*,#19215,.T.);
#26808=ORIENTED_EDGE('',*,*,#19216,.F.);
#26809=ORIENTED_EDGE('',*,*,#18855,.T.);
#26810=ORIENTED_EDGE('',*,*,#18781,.T.);
#26811=ORIENTED_EDGE('',*,*,#18780,.T.);
#26812=ORIENTED_EDGE('',*,*,#19217,.F.);
#26813=ORIENTED_EDGE('',*,*,#19111,.F.);
#26814=ORIENTED_EDGE('',*,*,#19218,.F.);
#26815=ORIENTED_EDGE('',*,*,#19219,.F.);
#26816=ORIENTED_EDGE('',*,*,#19114,.T.);
#26817=ORIENTED_EDGE('',*,*,#19217,.T.);
#26818=ORIENTED_EDGE('',*,*,#19220,.T.);
#26819=ORIENTED_EDGE('',*,*,#19221,.T.);
#26820=ORIENTED_EDGE('',*,*,#19222,.F.);
#26821=ORIENTED_EDGE('',*,*,#18845,.T.);
#26822=ORIENTED_EDGE('',*,*,#18802,.T.);
#26823=ORIENTED_EDGE('',*,*,#18801,.T.);
#26824=ORIENTED_EDGE('',*,*,#19223,.F.);
#26825=ORIENTED_EDGE('',*,*,#19095,.F.);
#26826=ORIENTED_EDGE('',*,*,#19147,.F.);
#26827=ORIENTED_EDGE('',*,*,#19148,.T.);
#26828=ORIENTED_EDGE('',*,*,#19098,.T.);
#26829=ORIENTED_EDGE('',*,*,#19223,.T.);
#26830=ORIENTED_EDGE('',*,*,#18840,.T.);
#26831=ORIENTED_EDGE('',*,*,#19108,.T.);
#26832=ORIENTED_EDGE('',*,*,#19224,.F.);
#26833=ORIENTED_EDGE('',*,*,#18805,.F.);
#26834=ORIENTED_EDGE('',*,*,#18804,.F.);
#26835=ORIENTED_EDGE('',*,*,#19110,.F.);
#26836=ORIENTED_EDGE('',*,*,#19143,.T.);
#26837=ORIENTED_EDGE('',*,*,#19144,.T.);
#26838=ORIENTED_EDGE('',*,*,#19224,.T.);
#26839=ORIENTED_EDGE('',*,*,#19225,.T.);
#26840=ORIENTED_EDGE('',*,*,#19130,.T.);
#26841=ORIENTED_EDGE('',*,*,#19226,.T.);
#26842=ORIENTED_EDGE('',*,*,#19227,.F.);
#26843=ORIENTED_EDGE('',*,*,#19133,.T.);
#26844=ORIENTED_EDGE('',*,*,#19228,.T.);
#26845=ORIENTED_EDGE('',*,*,#19229,.F.);
#26846=ORIENTED_EDGE('',*,*,#19226,.F.);
#26847=ORIENTED_EDGE('',*,*,#19138,.T.);
#26848=ORIENTED_EDGE('',*,*,#19230,.T.);
#26849=ORIENTED_EDGE('',*,*,#19231,.F.);
#26850=ORIENTED_EDGE('',*,*,#19228,.F.);
#26851=ORIENTED_EDGE('',*,*,#19141,.T.);
#26852=ORIENTED_EDGE('',*,*,#19232,.T.);
#26853=ORIENTED_EDGE('',*,*,#19233,.F.);
#26854=ORIENTED_EDGE('',*,*,#19230,.F.);
#26855=ORIENTED_EDGE('',*,*,#19153,.T.);
#26856=ORIENTED_EDGE('',*,*,#19234,.T.);
#26857=ORIENTED_EDGE('',*,*,#19235,.F.);
#26858=ORIENTED_EDGE('',*,*,#19197,.F.);
#26859=ORIENTED_EDGE('',*,*,#19155,.T.);
#26860=ORIENTED_EDGE('',*,*,#19236,.T.);
#26861=ORIENTED_EDGE('',*,*,#19237,.F.);
#26862=ORIENTED_EDGE('',*,*,#19234,.F.);
#26863=ORIENTED_EDGE('',*,*,#19157,.T.);
#26864=ORIENTED_EDGE('',*,*,#19238,.T.);
#26865=ORIENTED_EDGE('',*,*,#19239,.F.);
#26866=ORIENTED_EDGE('',*,*,#19236,.F.);
#26867=ORIENTED_EDGE('',*,*,#19159,.T.);
#26868=ORIENTED_EDGE('',*,*,#19240,.T.);
#26869=ORIENTED_EDGE('',*,*,#19241,.F.);
#26870=ORIENTED_EDGE('',*,*,#19238,.F.);
#26871=ORIENTED_EDGE('',*,*,#19161,.T.);
#26872=ORIENTED_EDGE('',*,*,#19242,.T.);
#26873=ORIENTED_EDGE('',*,*,#19243,.F.);
#26874=ORIENTED_EDGE('',*,*,#19240,.F.);
#26875=ORIENTED_EDGE('',*,*,#19163,.T.);
#26876=ORIENTED_EDGE('',*,*,#19244,.T.);
#26877=ORIENTED_EDGE('',*,*,#19245,.F.);
#26878=ORIENTED_EDGE('',*,*,#19242,.F.);
#26879=ORIENTED_EDGE('',*,*,#19165,.T.);
#26880=ORIENTED_EDGE('',*,*,#19246,.T.);
#26881=ORIENTED_EDGE('',*,*,#19247,.F.);
#26882=ORIENTED_EDGE('',*,*,#19244,.F.);
#26883=ORIENTED_EDGE('',*,*,#19167,.T.);
#26884=ORIENTED_EDGE('',*,*,#19248,.T.);
#26885=ORIENTED_EDGE('',*,*,#19249,.F.);
#26886=ORIENTED_EDGE('',*,*,#19246,.F.);
#26887=ORIENTED_EDGE('',*,*,#19169,.T.);
#26888=ORIENTED_EDGE('',*,*,#19250,.T.);
#26889=ORIENTED_EDGE('',*,*,#19251,.F.);
#26890=ORIENTED_EDGE('',*,*,#19248,.F.);
#26891=ORIENTED_EDGE('',*,*,#19171,.T.);
#26892=ORIENTED_EDGE('',*,*,#19252,.T.);
#26893=ORIENTED_EDGE('',*,*,#19253,.F.);
#26894=ORIENTED_EDGE('',*,*,#19250,.F.);
#26895=ORIENTED_EDGE('',*,*,#19175,.T.);
#26896=ORIENTED_EDGE('',*,*,#19254,.F.);
#26897=ORIENTED_EDGE('',*,*,#19170,.F.);
#26898=ORIENTED_EDGE('',*,*,#19172,.T.);
#26899=ORIENTED_EDGE('',*,*,#19174,.T.);
#26900=ORIENTED_EDGE('',*,*,#19255,.T.);
#26901=ORIENTED_EDGE('',*,*,#19256,.F.);
#26902=ORIENTED_EDGE('',*,*,#19257,.F.);
#26903=ORIENTED_EDGE('',*,*,#19179,.T.);
#26904=ORIENTED_EDGE('',*,*,#19258,.F.);
#26905=ORIENTED_EDGE('',*,*,#19173,.F.);
#26906=ORIENTED_EDGE('',*,*,#19176,.T.);
#26907=ORIENTED_EDGE('',*,*,#19178,.T.);
#26908=ORIENTED_EDGE('',*,*,#19259,.T.);
#26909=ORIENTED_EDGE('',*,*,#19260,.F.);
#26910=ORIENTED_EDGE('',*,*,#19261,.F.);
#26911=ORIENTED_EDGE('',*,*,#19181,.T.);
#26912=ORIENTED_EDGE('',*,*,#19262,.T.);
#26913=ORIENTED_EDGE('',*,*,#19263,.F.);
#26914=ORIENTED_EDGE('',*,*,#19259,.F.);
#26915=ORIENTED_EDGE('',*,*,#19183,.T.);
#26916=ORIENTED_EDGE('',*,*,#19264,.T.);
#26917=ORIENTED_EDGE('',*,*,#19265,.F.);
#26918=ORIENTED_EDGE('',*,*,#19262,.F.);
#26919=ORIENTED_EDGE('',*,*,#19187,.T.);
#26920=ORIENTED_EDGE('',*,*,#19266,.F.);
#26921=ORIENTED_EDGE('',*,*,#19182,.F.);
#26922=ORIENTED_EDGE('',*,*,#19184,.T.);
#26923=ORIENTED_EDGE('',*,*,#19186,.T.);
#26924=ORIENTED_EDGE('',*,*,#19267,.T.);
#26925=ORIENTED_EDGE('',*,*,#19268,.F.);
#26926=ORIENTED_EDGE('',*,*,#19269,.F.);
#26927=ORIENTED_EDGE('',*,*,#19191,.T.);
#26928=ORIENTED_EDGE('',*,*,#19270,.F.);
#26929=ORIENTED_EDGE('',*,*,#19185,.F.);
#26930=ORIENTED_EDGE('',*,*,#19188,.T.);
#26931=ORIENTED_EDGE('',*,*,#19190,.T.);
#26932=ORIENTED_EDGE('',*,*,#19271,.T.);
#26933=ORIENTED_EDGE('',*,*,#19272,.F.);
#26934=ORIENTED_EDGE('',*,*,#19273,.F.);
#26935=ORIENTED_EDGE('',*,*,#19193,.T.);
#26936=ORIENTED_EDGE('',*,*,#19274,.T.);
#26937=ORIENTED_EDGE('',*,*,#19275,.F.);
#26938=ORIENTED_EDGE('',*,*,#19271,.F.);
#26939=ORIENTED_EDGE('',*,*,#19225,.F.);
#26940=ORIENTED_EDGE('',*,*,#19276,.F.);
#26941=ORIENTED_EDGE('',*,*,#19274,.F.);
#26942=ORIENTED_EDGE('',*,*,#19194,.T.);
#26943=ORIENTED_EDGE('',*,*,#19195,.F.);
#26944=ORIENTED_EDGE('',*,*,#19277,.F.);
#26945=ORIENTED_EDGE('',*,*,#19201,.T.);
#26946=ORIENTED_EDGE('',*,*,#19199,.T.);
#26947=ORIENTED_EDGE('',*,*,#19278,.F.);
#26948=ORIENTED_EDGE('',*,*,#19279,.T.);
#26949=ORIENTED_EDGE('',*,*,#19280,.T.);
#26950=ORIENTED_EDGE('',*,*,#19281,.F.);
#26951=ORIENTED_EDGE('',*,*,#19282,.F.);
#26952=ORIENTED_EDGE('',*,*,#19280,.F.);
#26953=ORIENTED_EDGE('',*,*,#18791,.T.);
#26954=ORIENTED_EDGE('',*,*,#19202,.F.);
#26955=ORIENTED_EDGE('',*,*,#19283,.F.);
#26956=ORIENTED_EDGE('',*,*,#19284,.T.);
#26957=ORIENTED_EDGE('',*,*,#19285,.F.);
#26958=ORIENTED_EDGE('',*,*,#19286,.T.);
#26959=ORIENTED_EDGE('',*,*,#19216,.T.);
#26960=ORIENTED_EDGE('',*,*,#19286,.F.);
#26961=ORIENTED_EDGE('',*,*,#19287,.T.);
#26962=ORIENTED_EDGE('',*,*,#19288,.T.);
#26963=ORIENTED_EDGE('',*,*,#19289,.F.);
#26964=ORIENTED_EDGE('',*,*,#19208,.F.);
#26965=ORIENTED_EDGE('',*,*,#19290,.T.);
#26966=ORIENTED_EDGE('',*,*,#19291,.T.);
#26967=ORIENTED_EDGE('',*,*,#19287,.F.);
#26968=ORIENTED_EDGE('',*,*,#19207,.F.);
#26969=ORIENTED_EDGE('',*,*,#19292,.T.);
#26970=ORIENTED_EDGE('',*,*,#19293,.T.);
#26971=ORIENTED_EDGE('',*,*,#19294,.F.);
#26972=ORIENTED_EDGE('',*,*,#19213,.F.);
#26973=ORIENTED_EDGE('',*,*,#19222,.T.);
#26974=ORIENTED_EDGE('',*,*,#19295,.T.);
#26975=ORIENTED_EDGE('',*,*,#19292,.F.);
#26976=ORIENTED_EDGE('',*,*,#19212,.F.);
#26977=ORIENTED_EDGE('',*,*,#19296,.T.);
#26978=ORIENTED_EDGE('',*,*,#19297,.T.);
#26979=ORIENTED_EDGE('',*,*,#19220,.F.);
#26980=ORIENTED_EDGE('',*,*,#19211,.F.);
#26981=ORIENTED_EDGE('',*,*,#19298,.T.);
#26982=ORIENTED_EDGE('',*,*,#19299,.F.);
#26983=ORIENTED_EDGE('',*,*,#19203,.F.);
#26984=ORIENTED_EDGE('',*,*,#19299,.T.);
#26985=ORIENTED_EDGE('',*,*,#19300,.T.);
#26986=ORIENTED_EDGE('',*,*,#19290,.F.);
#26987=ORIENTED_EDGE('',*,*,#19206,.F.);
#26988=ORIENTED_EDGE('',*,*,#19205,.T.);
#26989=ORIENTED_EDGE('',*,*,#19301,.F.);
#26990=ORIENTED_EDGE('',*,*,#19302,.F.);
#26991=ORIENTED_EDGE('',*,*,#19215,.F.);
#26992=ORIENTED_EDGE('',*,*,#19303,.T.);
#26993=ORIENTED_EDGE('',*,*,#19304,.T.);
#26994=ORIENTED_EDGE('',*,*,#19301,.T.);
#26995=ORIENTED_EDGE('',*,*,#19294,.T.);
#26996=ORIENTED_EDGE('',*,*,#19305,.T.);
#26997=ORIENTED_EDGE('',*,*,#19303,.F.);
#26998=ORIENTED_EDGE('',*,*,#19214,.F.);
#26999=ORIENTED_EDGE('',*,*,#19306,.T.);
#27000=ORIENTED_EDGE('',*,*,#19307,.T.);
#27001=ORIENTED_EDGE('',*,*,#19308,.F.);
#27002=ORIENTED_EDGE('',*,*,#19209,.F.);
#27003=ORIENTED_EDGE('',*,*,#19308,.T.);
#27004=ORIENTED_EDGE('',*,*,#19309,.T.);
#27005=ORIENTED_EDGE('',*,*,#19296,.F.);
#27006=ORIENTED_EDGE('',*,*,#19210,.F.);
#27007=ORIENTED_EDGE('',*,*,#18785,.T.);
#27008=ORIENTED_EDGE('',*,*,#19310,.F.);
#27009=ORIENTED_EDGE('',*,*,#19311,.F.);
#27010=ORIENTED_EDGE('',*,*,#19218,.T.);
#27011=ORIENTED_EDGE('',*,*,#19282,.T.);
#27012=ORIENTED_EDGE('',*,*,#19312,.T.);
#27013=ORIENTED_EDGE('',*,*,#19313,.F.);
#27014=ORIENTED_EDGE('',*,*,#19314,.F.);
#27015=ORIENTED_EDGE('',*,*,#19315,.F.);
#27016=ORIENTED_EDGE('',*,*,#19312,.F.);
#27017=ORIENTED_EDGE('',*,*,#19281,.T.);
#27018=ORIENTED_EDGE('',*,*,#19254,.T.);
#27019=ORIENTED_EDGE('',*,*,#19257,.T.);
#27020=ORIENTED_EDGE('',*,*,#19252,.F.);
#27021=ORIENTED_EDGE('',*,*,#19258,.T.);
#27022=ORIENTED_EDGE('',*,*,#19261,.T.);
#27023=ORIENTED_EDGE('',*,*,#19255,.F.);
#27024=ORIENTED_EDGE('',*,*,#19266,.T.);
#27025=ORIENTED_EDGE('',*,*,#19269,.T.);
#27026=ORIENTED_EDGE('',*,*,#19264,.F.);
#27027=ORIENTED_EDGE('',*,*,#19270,.T.);
#27028=ORIENTED_EDGE('',*,*,#19273,.T.);
#27029=ORIENTED_EDGE('',*,*,#19267,.F.);
#27030=ORIENTED_EDGE('',*,*,#19316,.T.);
#27031=ORIENTED_EDGE('',*,*,#19317,.T.);
#27032=ORIENTED_EDGE('',*,*,#19277,.T.);
#27033=ORIENTED_EDGE('',*,*,#19317,.F.);
#27034=ORIENTED_EDGE('',*,*,#19283,.T.);
#27035=ORIENTED_EDGE('',*,*,#19278,.T.);
#27036=ORIENTED_EDGE('',*,*,#19318,.F.);
#27037=ORIENTED_EDGE('',*,*,#19319,.F.);
#27038=ORIENTED_EDGE('',*,*,#19320,.T.);
#27039=ORIENTED_EDGE('',*,*,#19319,.T.);
#27040=ORIENTED_EDGE('',*,*,#19321,.F.);
#27041=ORIENTED_EDGE('',*,*,#19322,.F.);
#27042=ORIENTED_EDGE('',*,*,#19323,.T.);
#27043=ORIENTED_EDGE('',*,*,#19322,.T.);
#27044=ORIENTED_EDGE('',*,*,#19324,.F.);
#27045=ORIENTED_EDGE('',*,*,#19325,.F.);
#27046=ORIENTED_EDGE('',*,*,#19326,.T.);
#27047=ORIENTED_EDGE('',*,*,#19325,.T.);
#27048=ORIENTED_EDGE('',*,*,#19327,.F.);
#27049=ORIENTED_EDGE('',*,*,#19328,.F.);
#27050=ORIENTED_EDGE('',*,*,#19329,.T.);
#27051=ORIENTED_EDGE('',*,*,#19328,.T.);
#27052=ORIENTED_EDGE('',*,*,#19330,.F.);
#27053=ORIENTED_EDGE('',*,*,#19331,.F.);
#27054=ORIENTED_EDGE('',*,*,#19289,.T.);
#27055=ORIENTED_EDGE('',*,*,#19332,.T.);
#27056=ORIENTED_EDGE('',*,*,#19306,.F.);
#27057=ORIENTED_EDGE('',*,*,#19333,.T.);
#27058=ORIENTED_EDGE('',*,*,#19291,.F.);
#27059=ORIENTED_EDGE('',*,*,#19334,.F.);
#27060=ORIENTED_EDGE('',*,*,#19326,.F.);
#27061=ORIENTED_EDGE('',*,*,#18852,.T.);
#27062=ORIENTED_EDGE('',*,*,#19335,.T.);
#27063=ORIENTED_EDGE('',*,*,#19336,.F.);
#27064=ORIENTED_EDGE('',*,*,#19298,.F.);
#27065=ORIENTED_EDGE('',*,*,#19336,.T.);
#27066=ORIENTED_EDGE('',*,*,#19337,.F.);
#27067=ORIENTED_EDGE('',*,*,#19323,.F.);
#27068=ORIENTED_EDGE('',*,*,#19334,.T.);
#27069=ORIENTED_EDGE('',*,*,#19300,.F.);
#27070=ORIENTED_EDGE('',*,*,#19279,.F.);
#27071=ORIENTED_EDGE('',*,*,#19338,.T.);
#27072=ORIENTED_EDGE('',*,*,#19339,.T.);
#27073=ORIENTED_EDGE('',*,*,#19338,.F.);
#27074=ORIENTED_EDGE('',*,*,#19313,.T.);
#27075=ORIENTED_EDGE('',*,*,#19315,.T.);
#27076=ORIENTED_EDGE('',*,*,#19314,.T.);
#27077=ORIENTED_EDGE('',*,*,#19316,.F.);
#27078=ORIENTED_EDGE('',*,*,#19340,.T.);
#27079=ORIENTED_EDGE('',*,*,#19341,.T.);
#27080=ORIENTED_EDGE('',*,*,#19342,.F.);
#27081=ORIENTED_EDGE('',*,*,#19343,.F.);
#27082=ORIENTED_EDGE('',*,*,#19344,.F.);
#27083=ORIENTED_EDGE('',*,*,#19345,.T.);
#27084=ORIENTED_EDGE('',*,*,#19346,.T.);
#27085=ORIENTED_EDGE('',*,*,#19221,.F.);
#27086=ORIENTED_EDGE('',*,*,#19347,.T.);
#27087=ORIENTED_EDGE('',*,*,#19348,.T.);
#27088=ORIENTED_EDGE('',*,*,#19349,.F.);
#27089=ORIENTED_EDGE('',*,*,#19350,.F.);
#27090=ORIENTED_EDGE('',*,*,#19342,.T.);
#27091=ORIENTED_EDGE('',*,*,#19351,.T.);
#27092=ORIENTED_EDGE('',*,*,#19347,.F.);
#27093=ORIENTED_EDGE('',*,*,#19352,.F.);
#27094=ORIENTED_EDGE('',*,*,#18851,.T.);
#27095=ORIENTED_EDGE('',*,*,#18787,.T.);
#27096=ORIENTED_EDGE('',*,*,#18786,.T.);
#27097=ORIENTED_EDGE('',*,*,#19353,.F.);
#27098=ORIENTED_EDGE('',*,*,#19335,.F.);
#27099=ORIENTED_EDGE('',*,*,#19284,.F.);
#27100=ORIENTED_EDGE('',*,*,#19320,.F.);
#27101=ORIENTED_EDGE('',*,*,#19337,.T.);
#27102=ORIENTED_EDGE('',*,*,#19353,.T.);
#27103=ORIENTED_EDGE('',*,*,#19285,.T.);
#27104=ORIENTED_EDGE('',*,*,#19354,.T.);
#27105=ORIENTED_EDGE('',*,*,#19339,.F.);
#27106=ORIENTED_EDGE('',*,*,#19354,.F.);
#27107=ORIENTED_EDGE('',*,*,#19349,.T.);
#27108=ORIENTED_EDGE('',*,*,#19355,.T.);
#27109=ORIENTED_EDGE('',*,*,#19356,.F.);
#27110=ORIENTED_EDGE('',*,*,#19357,.F.);
#27111=ORIENTED_EDGE('',*,*,#19358,.T.);
#27112=ORIENTED_EDGE('',*,*,#19359,.T.);
#27113=ORIENTED_EDGE('',*,*,#19360,.F.);
#27114=ORIENTED_EDGE('',*,*,#19361,.F.);
#27115=ORIENTED_EDGE('',*,*,#19362,.T.);
#27116=ORIENTED_EDGE('',*,*,#19361,.T.);
#27117=ORIENTED_EDGE('',*,*,#19363,.F.);
#27118=ORIENTED_EDGE('',*,*,#19364,.F.);
#27119=ORIENTED_EDGE('',*,*,#19227,.T.);
#27120=ORIENTED_EDGE('',*,*,#19229,.T.);
#27121=ORIENTED_EDGE('',*,*,#19231,.T.);
#27122=ORIENTED_EDGE('',*,*,#19233,.T.);
#27123=ORIENTED_EDGE('',*,*,#19365,.T.);
#27124=ORIENTED_EDGE('',*,*,#19366,.T.);
#27125=ORIENTED_EDGE('',*,*,#19367,.T.);
#27126=ORIENTED_EDGE('',*,*,#19363,.T.);
#27127=ORIENTED_EDGE('',*,*,#19360,.T.);
#27128=ORIENTED_EDGE('',*,*,#19368,.T.);
#27129=ORIENTED_EDGE('',*,*,#19369,.T.);
#27130=ORIENTED_EDGE('',*,*,#19370,.T.);
#27131=ORIENTED_EDGE('',*,*,#19371,.T.);
#27132=ORIENTED_EDGE('',*,*,#19372,.T.);
#27133=ORIENTED_EDGE('',*,*,#19373,.T.);
#27134=ORIENTED_EDGE('',*,*,#19374,.T.);
#27135=ORIENTED_EDGE('',*,*,#19375,.T.);
#27136=ORIENTED_EDGE('',*,*,#19330,.T.);
#27137=ORIENTED_EDGE('',*,*,#19327,.T.);
#27138=ORIENTED_EDGE('',*,*,#19324,.T.);
#27139=ORIENTED_EDGE('',*,*,#19321,.T.);
#27140=ORIENTED_EDGE('',*,*,#19318,.T.);
#27141=ORIENTED_EDGE('',*,*,#19198,.T.);
#27142=ORIENTED_EDGE('',*,*,#19235,.T.);
#27143=ORIENTED_EDGE('',*,*,#19237,.T.);
#27144=ORIENTED_EDGE('',*,*,#19239,.T.);
#27145=ORIENTED_EDGE('',*,*,#19241,.T.);
#27146=ORIENTED_EDGE('',*,*,#19243,.T.);
#27147=ORIENTED_EDGE('',*,*,#19245,.T.);
#27148=ORIENTED_EDGE('',*,*,#19247,.T.);
#27149=ORIENTED_EDGE('',*,*,#19249,.T.);
#27150=ORIENTED_EDGE('',*,*,#19251,.T.);
#27151=ORIENTED_EDGE('',*,*,#19253,.T.);
#27152=ORIENTED_EDGE('',*,*,#19256,.T.);
#27153=ORIENTED_EDGE('',*,*,#19260,.T.);
#27154=ORIENTED_EDGE('',*,*,#19263,.T.);
#27155=ORIENTED_EDGE('',*,*,#19265,.T.);
#27156=ORIENTED_EDGE('',*,*,#19268,.T.);
#27157=ORIENTED_EDGE('',*,*,#19272,.T.);
#27158=ORIENTED_EDGE('',*,*,#19275,.T.);
#27159=ORIENTED_EDGE('',*,*,#19276,.T.);
#27160=ORIENTED_EDGE('',*,*,#19115,.T.);
#27161=ORIENTED_EDGE('',*,*,#19376,.T.);
#27162=ORIENTED_EDGE('',*,*,#19365,.F.);
#27163=ORIENTED_EDGE('',*,*,#19232,.F.);
#27164=ORIENTED_EDGE('',*,*,#19219,.T.);
#27165=ORIENTED_EDGE('',*,*,#19377,.T.);
#27166=ORIENTED_EDGE('',*,*,#19376,.F.);
#27167=ORIENTED_EDGE('',*,*,#19311,.T.);
#27168=ORIENTED_EDGE('',*,*,#19378,.T.);
#27169=ORIENTED_EDGE('',*,*,#19366,.F.);
#27170=ORIENTED_EDGE('',*,*,#19377,.F.);
#27171=ORIENTED_EDGE('',*,*,#19379,.T.);
#27172=ORIENTED_EDGE('',*,*,#19364,.T.);
#27173=ORIENTED_EDGE('',*,*,#19367,.F.);
#27174=ORIENTED_EDGE('',*,*,#19378,.F.);
#27175=ORIENTED_EDGE('',*,*,#18854,.T.);
#27176=ORIENTED_EDGE('',*,*,#19302,.T.);
#27177=ORIENTED_EDGE('',*,*,#19380,.F.);
#27178=ORIENTED_EDGE('',*,*,#18784,.F.);
#27179=ORIENTED_EDGE('',*,*,#18783,.F.);
#27180=ORIENTED_EDGE('',*,*,#19304,.F.);
#27181=ORIENTED_EDGE('',*,*,#19381,.F.);
#27182=ORIENTED_EDGE('',*,*,#19379,.F.);
#27183=ORIENTED_EDGE('',*,*,#19310,.T.);
#27184=ORIENTED_EDGE('',*,*,#19380,.T.);
#27185=ORIENTED_EDGE('',*,*,#19362,.F.);
#27186=ORIENTED_EDGE('',*,*,#19381,.T.);
#27187=ORIENTED_EDGE('',*,*,#19305,.F.);
#27188=ORIENTED_EDGE('',*,*,#19382,.F.);
#27189=ORIENTED_EDGE('',*,*,#19382,.T.);
#27190=ORIENTED_EDGE('',*,*,#19293,.F.);
#27191=ORIENTED_EDGE('',*,*,#19383,.F.);
#27192=ORIENTED_EDGE('',*,*,#19358,.F.);
#27193=ORIENTED_EDGE('',*,*,#19384,.F.);
#27194=ORIENTED_EDGE('',*,*,#19383,.T.);
#27195=ORIENTED_EDGE('',*,*,#19295,.F.);
#27196=ORIENTED_EDGE('',*,*,#19346,.F.);
#27197=ORIENTED_EDGE('',*,*,#19385,.F.);
#27198=ORIENTED_EDGE('',*,*,#19386,.F.);
#27199=ORIENTED_EDGE('',*,*,#19387,.F.);
#27200=ORIENTED_EDGE('',*,*,#19388,.F.);
#27201=ORIENTED_EDGE('',*,*,#19384,.T.);
#27202=ORIENTED_EDGE('',*,*,#19389,.T.);
#27203=ORIENTED_EDGE('',*,*,#19368,.F.);
#27204=ORIENTED_EDGE('',*,*,#19359,.F.);
#27205=ORIENTED_EDGE('',*,*,#19390,.T.);
#27206=ORIENTED_EDGE('',*,*,#19391,.T.);
#27207=ORIENTED_EDGE('',*,*,#19369,.F.);
#27208=ORIENTED_EDGE('',*,*,#19389,.F.);
#27209=ORIENTED_EDGE('',*,*,#19392,.T.);
#27210=ORIENTED_EDGE('',*,*,#19393,.T.);
#27211=ORIENTED_EDGE('',*,*,#19370,.F.);
#27212=ORIENTED_EDGE('',*,*,#19391,.F.);
#27213=ORIENTED_EDGE('',*,*,#19394,.T.);
#27214=ORIENTED_EDGE('',*,*,#19395,.T.);
#27215=ORIENTED_EDGE('',*,*,#19371,.F.);
#27216=ORIENTED_EDGE('',*,*,#19393,.F.);
#27217=ORIENTED_EDGE('',*,*,#19396,.T.);
#27218=ORIENTED_EDGE('',*,*,#19397,.T.);
#27219=ORIENTED_EDGE('',*,*,#19372,.F.);
#27220=ORIENTED_EDGE('',*,*,#19395,.F.);
#27221=ORIENTED_EDGE('',*,*,#19398,.T.);
#27222=ORIENTED_EDGE('',*,*,#19399,.T.);
#27223=ORIENTED_EDGE('',*,*,#19373,.F.);
#27224=ORIENTED_EDGE('',*,*,#19397,.F.);
#27225=ORIENTED_EDGE('',*,*,#19400,.T.);
#27226=ORIENTED_EDGE('',*,*,#19401,.T.);
#27227=ORIENTED_EDGE('',*,*,#19374,.F.);
#27228=ORIENTED_EDGE('',*,*,#19399,.F.);
#27229=ORIENTED_EDGE('',*,*,#19402,.T.);
#27230=ORIENTED_EDGE('',*,*,#19331,.T.);
#27231=ORIENTED_EDGE('',*,*,#19375,.F.);
#27232=ORIENTED_EDGE('',*,*,#19401,.F.);
#27233=ORIENTED_EDGE('',*,*,#19403,.T.);
#27234=ORIENTED_EDGE('',*,*,#19404,.F.);
#27235=ORIENTED_EDGE('',*,*,#19405,.F.);
#27236=ORIENTED_EDGE('',*,*,#19402,.F.);
#27237=ORIENTED_EDGE('',*,*,#19406,.F.);
#27238=ORIENTED_EDGE('',*,*,#19407,.F.);
#27239=ORIENTED_EDGE('',*,*,#19408,.F.);
#27240=ORIENTED_EDGE('',*,*,#19403,.F.);
#27241=ORIENTED_EDGE('',*,*,#19400,.F.);
#27242=ORIENTED_EDGE('',*,*,#19398,.F.);
#27243=ORIENTED_EDGE('',*,*,#19409,.F.);
#27244=ORIENTED_EDGE('',*,*,#19341,.F.);
#27245=ORIENTED_EDGE('',*,*,#19406,.T.);
#27246=ORIENTED_EDGE('',*,*,#19410,.T.);
#27247=ORIENTED_EDGE('',*,*,#19351,.F.);
#27248=ORIENTED_EDGE('',*,*,#19409,.T.);
#27249=ORIENTED_EDGE('',*,*,#19396,.F.);
#27250=ORIENTED_EDGE('',*,*,#19411,.T.);
#27251=ORIENTED_EDGE('',*,*,#19348,.F.);
#27252=ORIENTED_EDGE('',*,*,#19410,.F.);
#27253=ORIENTED_EDGE('',*,*,#19394,.F.);
#27254=ORIENTED_EDGE('',*,*,#19412,.T.);
#27255=ORIENTED_EDGE('',*,*,#19355,.F.);
#27256=ORIENTED_EDGE('',*,*,#19411,.F.);
#27257=ORIENTED_EDGE('',*,*,#19392,.F.);
#27258=ORIENTED_EDGE('',*,*,#19388,.T.);
#27259=ORIENTED_EDGE('',*,*,#19413,.F.);
#27260=ORIENTED_EDGE('',*,*,#19412,.F.);
#27261=ORIENTED_EDGE('',*,*,#19390,.F.);
#27262=ORIENTED_EDGE('',*,*,#19356,.T.);
#27263=ORIENTED_EDGE('',*,*,#19413,.T.);
#27264=ORIENTED_EDGE('',*,*,#19414,.F.);
#27265=ORIENTED_EDGE('',*,*,#19415,.F.);
#27266=ORIENTED_EDGE('',*,*,#19414,.T.);
#27267=ORIENTED_EDGE('',*,*,#19387,.T.);
#27268=ORIENTED_EDGE('',*,*,#19416,.F.);
#27269=ORIENTED_EDGE('',*,*,#19417,.F.);
#27270=ORIENTED_EDGE('',*,*,#19416,.T.);
#27271=ORIENTED_EDGE('',*,*,#19386,.T.);
#27272=ORIENTED_EDGE('',*,*,#19418,.F.);
#27273=ORIENTED_EDGE('',*,*,#19419,.F.);
#27274=ORIENTED_EDGE('',*,*,#19418,.T.);
#27275=ORIENTED_EDGE('',*,*,#19385,.T.);
#27276=ORIENTED_EDGE('',*,*,#19345,.F.);
#27277=ORIENTED_EDGE('',*,*,#19420,.F.);
#27278=ORIENTED_EDGE('',*,*,#19420,.T.);
#27279=ORIENTED_EDGE('',*,*,#19421,.F.);
#27280=ORIENTED_EDGE('',*,*,#19422,.F.);
#27281=ORIENTED_EDGE('',*,*,#19297,.F.);
#27282=ORIENTED_EDGE('',*,*,#19423,.T.);
#27283=ORIENTED_EDGE('',*,*,#19421,.T.);
#27284=ORIENTED_EDGE('',*,*,#19344,.T.);
#27285=ORIENTED_EDGE('',*,*,#19424,.T.);
#27286=ORIENTED_EDGE('',*,*,#19425,.T.);
#27287=ORIENTED_EDGE('',*,*,#19423,.F.);
#27288=ORIENTED_EDGE('',*,*,#19309,.F.);
#27289=ORIENTED_EDGE('',*,*,#19307,.F.);
#27290=ORIENTED_EDGE('',*,*,#19426,.T.);
#27291=ORIENTED_EDGE('',*,*,#19427,.T.);
#27292=ORIENTED_EDGE('',*,*,#19424,.F.);
#27293=ORIENTED_EDGE('',*,*,#19428,.T.);
#27294=ORIENTED_EDGE('',*,*,#19429,.F.);
#27295=ORIENTED_EDGE('',*,*,#19426,.F.);
#27296=ORIENTED_EDGE('',*,*,#19332,.F.);
#27297=ORIENTED_EDGE('',*,*,#19405,.T.);
#27298=ORIENTED_EDGE('',*,*,#19430,.F.);
#27299=ORIENTED_EDGE('',*,*,#19431,.F.);
#27300=ORIENTED_EDGE('',*,*,#19428,.F.);
#27301=ORIENTED_EDGE('',*,*,#19288,.F.);
#27302=ORIENTED_EDGE('',*,*,#19333,.F.);
#27303=ORIENTED_EDGE('',*,*,#19329,.F.);
#27304=ORIENTED_EDGE('',*,*,#19432,.T.);
#27305=ORIENTED_EDGE('',*,*,#19430,.T.);
#27306=ORIENTED_EDGE('',*,*,#19433,.F.);
#27307=ORIENTED_EDGE('',*,*,#19434,.F.);
#27308=ORIENTED_EDGE('',*,*,#19429,.T.);
#27309=ORIENTED_EDGE('',*,*,#19431,.T.);
#27310=ORIENTED_EDGE('',*,*,#19432,.F.);
#27311=ORIENTED_EDGE('',*,*,#19435,.F.);
#27312=ORIENTED_EDGE('',*,*,#19435,.T.);
#27313=ORIENTED_EDGE('',*,*,#19436,.T.);
#27314=ORIENTED_EDGE('',*,*,#19427,.F.);
#27315=ORIENTED_EDGE('',*,*,#19422,.T.);
#27316=ORIENTED_EDGE('',*,*,#19425,.F.);
#27317=ORIENTED_EDGE('',*,*,#19436,.F.);
#27318=ORIENTED_EDGE('',*,*,#19434,.T.);
#27319=ORIENTED_EDGE('',*,*,#19437,.T.);
#27320=ORIENTED_EDGE('',*,*,#19438,.T.);
#27321=ORIENTED_EDGE('',*,*,#19439,.T.);
#27322=ORIENTED_EDGE('',*,*,#19419,.T.);
#27323=ORIENTED_EDGE('',*,*,#19433,.T.);
#27324=ORIENTED_EDGE('',*,*,#19404,.T.);
#27325=ORIENTED_EDGE('',*,*,#19440,.F.);
#27326=ORIENTED_EDGE('',*,*,#19437,.F.);
#27327=ORIENTED_EDGE('',*,*,#19440,.T.);
#27328=ORIENTED_EDGE('',*,*,#19408,.T.);
#27329=ORIENTED_EDGE('',*,*,#19441,.F.);
#27330=ORIENTED_EDGE('',*,*,#19438,.F.);
#27331=ORIENTED_EDGE('',*,*,#19441,.T.);
#27332=ORIENTED_EDGE('',*,*,#19407,.T.);
#27333=ORIENTED_EDGE('',*,*,#19340,.F.);
#27334=ORIENTED_EDGE('',*,*,#19442,.F.);
#27335=ORIENTED_EDGE('',*,*,#19442,.T.);
#27336=ORIENTED_EDGE('',*,*,#19343,.T.);
#27337=ORIENTED_EDGE('',*,*,#19352,.T.);
#27338=ORIENTED_EDGE('',*,*,#19350,.T.);
#27339=ORIENTED_EDGE('',*,*,#19357,.T.);
#27340=ORIENTED_EDGE('',*,*,#19415,.T.);
#27341=ORIENTED_EDGE('',*,*,#19417,.T.);
#27342=ORIENTED_EDGE('',*,*,#19439,.F.);
#32025=CONICAL_SURFACE('',#36201,0.781285626506967,0.663225115758);
#32874=ADVANCED_FACE('',(#4126),#138,.F.);
#32875=ADVANCED_FACE('',(#4127),#139,.F.);
#32876=ADVANCED_FACE('',(#4128),#140,.F.);
#32877=ADVANCED_FACE('',(#4129),#141,.F.);
#32878=ADVANCED_FACE('',(#4130),#142,.F.);
#32879=ADVANCED_FACE('',(#4131),#143,.T.);
#32880=ADVANCED_FACE('',(#4132),#2280,.F.);
#32881=ADVANCED_FACE('',(#4133),#2776,.T.);
#32882=ADVANCED_FACE('',(#4134),#2281,.F.);
#32883=ADVANCED_FACE('',(#4135),#2777,.F.);
#32884=ADVANCED_FACE('',(#4136),#2282,.F.);
#32885=ADVANCED_FACE('',(#4137),#736,.T.);
#32886=ADVANCED_FACE('',(#4138),#144,.T.);
#32887=ADVANCED_FACE('',(#4139),#1156,.T.);
#32888=ADVANCED_FACE('',(#4140,#1295),#737,.T.);
#32889=ADVANCED_FACE('',(#4141),#738,.T.);
#32890=ADVANCED_FACE('',(#4142),#145,.T.);
#32891=ADVANCED_FACE('',(#4143),#1157,.T.);
#32892=ADVANCED_FACE('',(#4144),#146,.T.);
#32893=ADVANCED_FACE('',(#4145),#2283,.T.);
#32894=ADVANCED_FACE('',(#4146),#2778,.F.);
#32895=ADVANCED_FACE('',(#4147,#1296),#2284,.T.);
#32896=ADVANCED_FACE('',(#4148),#2779,.F.);
#32897=ADVANCED_FACE('',(#4149),#147,.F.);
#32898=ADVANCED_FACE('',(#4150),#2780,.F.);
#32899=ADVANCED_FACE('',(#4151),#51,.T.);
#32900=ADVANCED_FACE('',(#4152),#2781,.F.);
#32901=ADVANCED_FACE('',(#4153),#52,.T.);
#32902=ADVANCED_FACE('',(#4154),#2782,.F.);
#32903=ADVANCED_FACE('',(#4155),#148,.T.);
#32904=ADVANCED_FACE('',(#4156),#2285,.F.);
#32905=ADVANCED_FACE('',(#4157),#1158,.F.);
#32906=ADVANCED_FACE('',(#4158),#2783,.T.);
#32907=ADVANCED_FACE('',(#4159),#2286,.F.);
#32908=ADVANCED_FACE('',(#4160),#2784,.F.);
#32909=ADVANCED_FACE('',(#4161),#2287,.F.);
#32910=ADVANCED_FACE('',(#4162),#2785,.F.);
#32911=ADVANCED_FACE('',(#4163),#1159,.T.);
#32912=ADVANCED_FACE('',(#4164),#2288,.T.);
#32913=ADVANCED_FACE('',(#4165),#1160,.F.);
#32914=ADVANCED_FACE('',(#4166),#1161,.F.);
#32915=ADVANCED_FACE('',(#4167),#53,.F.);
#32916=ADVANCED_FACE('',(#4168),#2786,.F.);
#32917=ADVANCED_FACE('',(#4169),#54,.F.);
#32918=ADVANCED_FACE('',(#4170),#2787,.T.);
#32919=ADVANCED_FACE('',(#4171),#2788,.F.);
#32920=ADVANCED_FACE('',(#4172),#149,.T.);
#32921=ADVANCED_FACE('',(#4173),#2789,.T.);
#32922=ADVANCED_FACE('',(#4174),#150,.T.);
#32923=ADVANCED_FACE('',(#4175),#2790,.T.);
#32924=ADVANCED_FACE('',(#4176),#151,.T.);
#32925=ADVANCED_FACE('',(#4177),#1162,.T.);
#32926=ADVANCED_FACE('',(#4178),#2791,.F.);
#32927=ADVANCED_FACE('',(#4179),#2792,.F.);
#32928=ADVANCED_FACE('',(#4180),#2793,.F.);
#32929=ADVANCED_FACE('',(#4181),#2794,.T.);
#32930=ADVANCED_FACE('',(#4182),#2289,.F.);
#32931=ADVANCED_FACE('',(#4183),#1163,.F.);
#32932=ADVANCED_FACE('',(#4184),#2795,.T.);
#32933=ADVANCED_FACE('',(#4185),#152,.F.);
#32934=ADVANCED_FACE('',(#4186),#2796,.T.);
#32935=ADVANCED_FACE('',(#4187),#153,.T.);
#32936=ADVANCED_FACE('',(#4188),#2290,.T.);
#32937=ADVANCED_FACE('',(#4189),#739,.F.);
#32938=ADVANCED_FACE('',(#4190),#154,.F.);
#32939=ADVANCED_FACE('',(#4191,#1297),#2291,.T.);
#32940=ADVANCED_FACE('',(#4192),#155,.F.);
#32941=ADVANCED_FACE('',(#4193),#2292,.T.);
#32942=ADVANCED_FACE('',(#4194),#156,.T.);
#32943=ADVANCED_FACE('',(#4195),#2797,.F.);
#32944=ADVANCED_FACE('',(#4196),#2798,.F.);
#32945=ADVANCED_FACE('',(#4197),#2799,.F.);
#32946=ADVANCED_FACE('',(#4198),#2800,.T.);
#32947=ADVANCED_FACE('',(#4199),#157,.F.);
#32948=ADVANCED_FACE('',(#4200),#158,.F.);
#32949=ADVANCED_FACE('',(#4201),#2801,.T.);
#32950=ADVANCED_FACE('',(#4202),#159,.T.);
#32951=ADVANCED_FACE('',(#4203),#2802,.T.);
#32952=ADVANCED_FACE('',(#4204),#160,.T.);
#32953=ADVANCED_FACE('',(#4205),#161,.T.);
#32954=ADVANCED_FACE('',(#4206),#2803,.T.);
#32955=ADVANCED_FACE('',(#4207),#162,.T.);
#32956=ADVANCED_FACE('',(#4208),#2804,.T.);
#32957=ADVANCED_FACE('',(#4209),#163,.T.);
#32958=ADVANCED_FACE('',(#4210),#2805,.T.);
#32959=ADVANCED_FACE('',(#4211),#164,.T.);
#32960=ADVANCED_FACE('',(#4212),#2806,.T.);
#32961=ADVANCED_FACE('',(#4213),#165,.T.);
#32962=ADVANCED_FACE('',(#4214),#166,.T.);
#32963=ADVANCED_FACE('',(#4215),#2807,.T.);
#32964=ADVANCED_FACE('',(#4216),#167,.T.);
#32965=ADVANCED_FACE('',(#4217),#2808,.T.);
#32966=ADVANCED_FACE('',(#4218),#168,.T.);
#32967=ADVANCED_FACE('',(#4219),#2809,.T.);
#32968=ADVANCED_FACE('',(#4220),#169,.T.);
#32969=ADVANCED_FACE('',(#4221),#2810,.T.);
#32970=ADVANCED_FACE('',(#4222),#170,.T.);
#32971=ADVANCED_FACE('',(#4223),#2811,.T.);
#32972=ADVANCED_FACE('',(#4224),#2812,.T.);
#32973=ADVANCED_FACE('',(#4225),#2813,.T.);
#32974=ADVANCED_FACE('',(#4226),#171,.T.);
#32975=ADVANCED_FACE('',(#4227),#2814,.T.);
#32976=ADVANCED_FACE('',(#4228),#2815,.T.);
#32977=ADVANCED_FACE('',(#4229),#2816,.T.);
#32978=ADVANCED_FACE('',(#4230),#172,.T.);
#32979=ADVANCED_FACE('',(#4231),#2817,.T.);
#32980=ADVANCED_FACE('',(#4232),#173,.F.);
#32981=ADVANCED_FACE('',(#4233),#174,.F.);
#32982=ADVANCED_FACE('',(#4234),#175,.F.);
#32983=ADVANCED_FACE('',(#4235),#2818,.F.);
#32984=ADVANCED_FACE('',(#4236),#176,.F.);
#32985=ADVANCED_FACE('',(#4237),#2819,.F.);
#32986=ADVANCED_FACE('',(#4238),#177,.F.);
#32987=ADVANCED_FACE('',(#4239),#2820,.F.);
#32988=ADVANCED_FACE('',(#4240),#178,.F.);
#32989=ADVANCED_FACE('',(#4241),#2821,.F.);
#32990=ADVANCED_FACE('',(#4242),#740,.F.);
#32991=ADVANCED_FACE('',(#4243),#2822,.F.);
#32992=ADVANCED_FACE('',(#4244),#741,.F.);
#32993=ADVANCED_FACE('',(#4245),#179,.F.);
#32994=ADVANCED_FACE('',(#4246),#2823,.F.);
#32995=ADVANCED_FACE('',(#4247),#1164,.T.);
#32996=ADVANCED_FACE('',(#4248),#2824,.T.);
#32997=ADVANCED_FACE('',(#4249),#742,.F.);
#32998=ADVANCED_FACE('',(#4250),#180,.F.);
#32999=ADVANCED_FACE('',(#4251),#2293,.F.);
#33000=ADVANCED_FACE('',(#4252),#2294,.F.);
#33001=ADVANCED_FACE('',(#4253),#2825,.T.);
#33002=ADVANCED_FACE('',(#4254),#181,.F.);
#33003=ADVANCED_FACE('',(#4255),#2295,.F.);
#33004=ADVANCED_FACE('',(#4256),#1165,.T.);
#33005=ADVANCED_FACE('',(#4257),#2826,.T.);
#33006=ADVANCED_FACE('',(#4258),#1166,.T.);
#33007=ADVANCED_FACE('',(#4259),#2827,.T.);
#33008=ADVANCED_FACE('',(#4260),#743,.T.);
#33009=ADVANCED_FACE('',(#4261),#2296,.T.);
#33010=ADVANCED_FACE('',(#4262),#1167,.T.);
#33011=ADVANCED_FACE('',(#4263),#2828,.T.);
#33012=ADVANCED_FACE('',(#4264),#2297,.T.);
#33013=ADVANCED_FACE('',(#4265),#744,.T.);
#33014=ADVANCED_FACE('',(#4266),#1168,.T.);
#33015=ADVANCED_FACE('',(#4267),#2829,.T.);
#33016=ADVANCED_FACE('',(#4268),#1169,.T.);
#33017=ADVANCED_FACE('',(#4269),#2830,.T.);
#33018=ADVANCED_FACE('',(#4270),#2298,.T.);
#33019=ADVANCED_FACE('',(#4271),#2831,.T.);
#33020=ADVANCED_FACE('',(#4272),#2299,.T.);
#33021=ADVANCED_FACE('',(#4273),#2832,.T.);
#33022=ADVANCED_FACE('',(#4274),#2300,.T.);
#33023=ADVANCED_FACE('',(#4275),#2833,.F.);
#33024=ADVANCED_FACE('',(#4276),#2301,.T.);
#33025=ADVANCED_FACE('',(#4277),#2834,.F.);
#33026=ADVANCED_FACE('',(#4278),#2302,.T.);
#33027=ADVANCED_FACE('',(#4279),#745,.T.);
#33028=ADVANCED_FACE('',(#4280),#2303,.T.);
#33029=ADVANCED_FACE('',(#4281),#746,.T.);
#33030=ADVANCED_FACE('',(#4282),#2304,.T.);
#33031=ADVANCED_FACE('',(#4283),#2835,.F.);
#33032=ADVANCED_FACE('',(#4284),#2305,.T.);
#33033=ADVANCED_FACE('',(#4285),#747,.T.);
#33034=ADVANCED_FACE('',(#4286),#2306,.T.);
#33035=ADVANCED_FACE('',(#4287),#748,.T.);
#33036=ADVANCED_FACE('',(#4288),#2307,.F.);
#33037=ADVANCED_FACE('',(#4289),#2836,.F.);
#33038=ADVANCED_FACE('',(#4290),#2308,.T.);
#33039=ADVANCED_FACE('',(#4291),#2837,.T.);
#33040=ADVANCED_FACE('',(#4292),#182,.T.);
#33041=ADVANCED_FACE('',(#4293),#1170,.T.);
#33042=ADVANCED_FACE('',(#4294),#2838,.T.);
#33043=ADVANCED_FACE('',(#4295),#183,.F.);
#33044=ADVANCED_FACE('',(#4296,#1298),#2309,.F.);
#33045=ADVANCED_FACE('',(#4297),#1171,.T.);
#33046=ADVANCED_FACE('',(#4298),#2839,.T.);
#33047=ADVANCED_FACE('',(#4299),#749,.F.);
#33048=ADVANCED_FACE('',(#4300),#1172,.T.);
#33049=ADVANCED_FACE('',(#4301),#2840,.T.);
#33050=ADVANCED_FACE('',(#4302),#1173,.T.);
#33051=ADVANCED_FACE('',(#4303),#2841,.T.);
#33052=ADVANCED_FACE('',(#4304),#2842,.T.);
#33053=ADVANCED_FACE('',(#4305),#184,.T.);
#33054=ADVANCED_FACE('',(#4306),#2843,.T.);
#33055=ADVANCED_FACE('',(#4307),#185,.T.);
#33056=ADVANCED_FACE('',(#4308),#186,.T.);
#33057=ADVANCED_FACE('',(#4309),#2844,.T.);
#33058=ADVANCED_FACE('',(#4310),#187,.T.);
#33059=ADVANCED_FACE('',(#4311),#2845,.T.);
#33060=ADVANCED_FACE('',(#4312),#188,.T.);
#33061=ADVANCED_FACE('',(#4313),#2846,.T.);
#33062=ADVANCED_FACE('',(#4314),#189,.T.);
#33063=ADVANCED_FACE('',(#4315),#2847,.T.);
#33064=ADVANCED_FACE('',(#4316),#190,.T.);
#33065=ADVANCED_FACE('',(#4317),#2848,.T.);
#33066=ADVANCED_FACE('',(#4318),#2849,.T.);
#33067=ADVANCED_FACE('',(#4319),#2850,.T.);
#33068=ADVANCED_FACE('',(#4320),#2851,.T.);
#33069=ADVANCED_FACE('',(#4321),#2852,.T.);
#33070=ADVANCED_FACE('',(#4322),#191,.T.);
#33071=ADVANCED_FACE('',(#4323),#2853,.T.);
#33072=ADVANCED_FACE('',(#4324),#2854,.T.);
#33073=ADVANCED_FACE('',(#4325),#2855,.T.);
#33074=ADVANCED_FACE('',(#4326),#2856,.T.);
#33075=ADVANCED_FACE('',(#4327),#2857,.T.);
#33076=ADVANCED_FACE('',(#4328),#192,.T.);
#33077=ADVANCED_FACE('',(#4329),#2858,.T.);
#33078=ADVANCED_FACE('',(#4330,#1299),#2310,.T.);
#33079=ADVANCED_FACE('',(#4331),#750,.T.);
#33080=ADVANCED_FACE('',(#4332),#32025,.T.);
#33081=ADVANCED_FACE('',(#4333),#2311,.F.);
#33082=ADVANCED_FACE('',(#4334),#193,.F.);
#33083=ADVANCED_FACE('',(#4335),#2859,.F.);
#33084=ADVANCED_FACE('',(#4336),#194,.F.);
#33085=ADVANCED_FACE('',(#4337),#195,.F.);
#33086=ADVANCED_FACE('',(#4338),#2860,.F.);
#33087=ADVANCED_FACE('',(#4339),#196,.F.);
#33088=ADVANCED_FACE('',(#4340),#751,.F.);
#33089=ADVANCED_FACE('',(#4341),#2861,.F.);
#33090=ADVANCED_FACE('',(#4342),#752,.F.);
#33091=ADVANCED_FACE('',(#4343),#197,.F.);
#33092=ADVANCED_FACE('',(#4344),#2862,.F.);
#33093=ADVANCED_FACE('',(#4345),#198,.F.);
#33094=ADVANCED_FACE('',(#4346),#199,.F.);
#33095=ADVANCED_FACE('',(#4347),#2312,.F.);
#33096=ADVANCED_FACE('',(#4348),#200,.T.);
#33097=ADVANCED_FACE('',(#4349),#753,.T.);
#33098=ADVANCED_FACE('',(#4350),#754,.T.);
#33099=ADVANCED_FACE('',(#4351),#755,.T.);
#33100=ADVANCED_FACE('',(#4352),#756,.T.);
#33101=ADVANCED_FACE('',(#4353),#2863,.F.);
#33102=ADVANCED_FACE('',(#4354),#2864,.T.);
#33103=ADVANCED_FACE('',(#4355),#201,.T.);
#33104=ADVANCED_FACE('',(#4356),#2865,.T.);
#33105=ADVANCED_FACE('',(#4357),#202,.T.);
#33106=ADVANCED_FACE('',(#4358),#2866,.T.);
#33107=ADVANCED_FACE('',(#4359),#757,.F.);
#33108=ADVANCED_FACE('',(#4360),#2867,.F.);
#33109=ADVANCED_FACE('',(#4361),#203,.F.);
#33110=ADVANCED_FACE('',(#4362),#2313,.F.);
#33111=ADVANCED_FACE('',(#4363),#204,.T.);
#33112=ADVANCED_FACE('',(#4364,#1300),#2314,.F.);
#33113=ADVANCED_FACE('',(#4365),#205,.F.);
#33114=ADVANCED_FACE('',(#4366),#2868,.F.);
#33115=ADVANCED_FACE('',(#4367),#55,.T.);
#33116=ADVANCED_FACE('',(#4368),#2869,.F.);
#33117=ADVANCED_FACE('',(#4369),#1174,.T.);
#33118=ADVANCED_FACE('',(#4370),#2870,.T.);
#33119=ADVANCED_FACE('',(#4371),#2871,.T.);
#33120=ADVANCED_FACE('',(#4372),#2872,.F.);
#33121=ADVANCED_FACE('',(#4373),#206,.T.);
#33122=ADVANCED_FACE('',(#4374),#2873,.T.);
#33123=ADVANCED_FACE('',(#4375),#2315,.F.);
#33124=ADVANCED_FACE('',(#4376),#207,.T.);
#33125=ADVANCED_FACE('',(#4377),#758,.T.);
#33126=ADVANCED_FACE('',(#4378),#2874,.T.);
#33127=ADVANCED_FACE('',(#4379),#208,.T.);
#33128=ADVANCED_FACE('',(#4380),#1175,.T.);
#33129=ADVANCED_FACE('',(#4381),#2875,.T.);
#33130=ADVANCED_FACE('',(#4382),#2316,.T.);
#33131=ADVANCED_FACE('',(#4383),#2876,.F.);
#33132=ADVANCED_FACE('',(#4384),#2317,.T.);
#33133=ADVANCED_FACE('',(#4385),#2877,.T.);
#33134=ADVANCED_FACE('',(#4386),#209,.T.);
#33135=ADVANCED_FACE('',(#4387),#2878,.T.);
#33136=ADVANCED_FACE('',(#4388),#210,.T.);
#33137=ADVANCED_FACE('',(#4389),#2879,.T.);
#33138=ADVANCED_FACE('',(#4390),#211,.T.);
#33139=ADVANCED_FACE('',(#4391),#2880,.T.);
#33140=ADVANCED_FACE('',(#4392),#212,.T.);
#33141=ADVANCED_FACE('',(#4393),#2881,.F.);
#33142=ADVANCED_FACE('',(#4394),#2318,.F.);
#33143=ADVANCED_FACE('',(#4395),#2882,.T.);
#33144=ADVANCED_FACE('',(#4396),#2319,.F.);
#33145=ADVANCED_FACE('',(#4397),#2883,.F.);
#33146=ADVANCED_FACE('',(#4398),#2320,.F.);
#33147=ADVANCED_FACE('',(#4399),#2884,.F.);
#33148=ADVANCED_FACE('',(#4400),#56,.T.);
#33149=ADVANCED_FACE('',(#4401),#2885,.F.);
#33150=ADVANCED_FACE('',(#4402),#1176,.F.);
#33151=ADVANCED_FACE('',(#4403),#1177,.F.);
#33152=ADVANCED_FACE('',(#4404),#57,.F.);
#33153=ADVANCED_FACE('',(#4405),#2886,.T.);
#33154=ADVANCED_FACE('',(#4406),#2887,.F.);
#33155=ADVANCED_FACE('',(#4407),#2888,.T.);
#33156=ADVANCED_FACE('',(#4408),#2889,.F.);
#33157=ADVANCED_FACE('',(#4409),#2321,.F.);
#33158=ADVANCED_FACE('',(#4410),#1178,.T.);
#33159=ADVANCED_FACE('',(#4411),#1179,.T.);
#33160=ADVANCED_FACE('',(#4412),#58,.F.);
#33161=ADVANCED_FACE('',(#4413),#213,.T.);
#33162=ADVANCED_FACE('',(#4414),#1180,.T.);
#33163=ADVANCED_FACE('',(#4415),#1181,.T.);
#33164=ADVANCED_FACE('',(#4416),#2890,.F.);
#33165=ADVANCED_FACE('',(#4417),#2322,.F.);
#34174=CLOSED_SHELL('',(#32874,#32875,#32876,#32877,#32878,#32879,#32880,
#32881,#32882,#32883,#32884,#32885,#32886,#32887,#32888,#32889,#32890,#32891,
#32892,#32893,#32894,#32895,#32896,#32897,#32898,#32899,#32900,#32901,#32902,
#32903,#32904,#32905,#32906,#32907,#32908,#32909,#32910,#32911,#32912,#32913,
#32914,#32915,#32916,#32917,#32918,#32919,#32920,#32921,#32922,#32923,#32924,
#32925,#32926,#32927,#32928,#32929,#32930,#32931,#32932,#32933,#32934,#32935,
#32936,#32937,#32938,#32939,#32940,#32941,#32942,#32943,#32944,#32945,#32946,
#32947,#32948,#32949,#32950,#32951,#32952,#32953,#32954,#32955,#32956,#32957,
#32958,#32959,#32960,#32961,#32962,#32963,#32964,#32965,#32966,#32967,#32968,
#32969,#32970,#32971,#32972,#32973,#32974,#32975,#32976,#32977,#32978,#32979,
#32980,#32981,#32982,#32983,#32984,#32985,#32986,#32987,#32988,#32989,#32990,
#32991,#32992,#32993,#32994,#32995,#32996,#32997,#32998,#32999,#33000,#33001,
#33002,#33003,#33004,#33005,#33006,#33007,#33008,#33009,#33010,#33011,#33012,
#33013,#33014,#33015,#33016,#33017,#33018,#33019,#33020,#33021,#33022,#33023,
#33024,#33025,#33026,#33027,#33028,#33029,#33030,#33031,#33032,#33033,#33034,
#33035,#33036,#33037,#33038,#33039,#33040,#33041,#33042,#33043,#33044,#33045,
#33046,#33047,#33048,#33049,#33050,#33051,#33052,#33053,#33054,#33055,#33056,
#33057,#33058,#33059,#33060,#33061,#33062,#33063,#33064,#33065,#33066,#33067,
#33068,#33069,#33070,#33071,#33072,#33073,#33074,#33075,#33076,#33077,#33078,
#33079,#33080,#33081,#33082,#33083,#33084,#33085,#33086,#33087,#33088,#33089,
#33090,#33091,#33092,#33093,#33094,#33095,#33096,#33097,#33098,#33099,#33100,
#33101,#33102,#33103,#33104,#33105,#33106,#33107,#33108,#33109,#33110,#33111,
#33112,#33113,#33114,#33115,#33116,#33117,#33118,#33119,#33120,#33121,#33122,
#33123,#33124,#33125,#33126,#33127,#33128,#33129,#33130,#33131,#33132,#33133,
#33134,#33135,#33136,#33137,#33138,#33139,#33140,#33141,#33142,#33143,#33144,
#33145,#33146,#33147,#33148,#33149,#33150,#33151,#33152,#33153,#33154,#33155,
#33156,#33157,#33158,#33159,#33160,#33161,#33162,#33163,#33164,#33165));
#35726=AXIS2_PLACEMENT_3D('',#78623,#42297,#42298);
#35727=AXIS2_PLACEMENT_3D('',#78624,#42299,#42300);
#35728=AXIS2_PLACEMENT_3D('',#78634,#42301,#42302);
#35729=AXIS2_PLACEMENT_3D('',#78636,#42303,#42304);
#35730=AXIS2_PLACEMENT_3D('',#78638,#42305,#42306);
#35731=AXIS2_PLACEMENT_3D('',#78646,#42307,#42308);
#35732=AXIS2_PLACEMENT_3D('',#78647,#42309,#42310);
#35733=AXIS2_PLACEMENT_3D('',#78650,#42311,#42312);
#35734=AXIS2_PLACEMENT_3D('',#78652,#42313,#42314);
#35735=AXIS2_PLACEMENT_3D('',#78654,#42315,#42316);
#35736=AXIS2_PLACEMENT_3D('',#78656,#42317,#42318);
#35737=AXIS2_PLACEMENT_3D('',#78658,#42319,#42320);
#35738=AXIS2_PLACEMENT_3D('',#78659,#42321,#42322);
#35739=AXIS2_PLACEMENT_3D('',#78660,#42323,#42324);
#35740=AXIS2_PLACEMENT_3D('',#78663,#42325,#42326);
#35741=AXIS2_PLACEMENT_3D('',#78665,#42327,#42328);
#35742=AXIS2_PLACEMENT_3D('',#78667,#42329,#42330);
#35743=AXIS2_PLACEMENT_3D('',#78669,#42331,#42332);
#35744=AXIS2_PLACEMENT_3D('',#78671,#42333,#42334);
#35745=AXIS2_PLACEMENT_3D('',#78672,#42335,#42336);
#35746=AXIS2_PLACEMENT_3D('',#78673,#42337,#42338);
#35747=AXIS2_PLACEMENT_3D('',#78676,#42339,#42340);
#35748=AXIS2_PLACEMENT_3D('',#78685,#42341,#42342);
#35749=AXIS2_PLACEMENT_3D('',#78687,#42343,#42344);
#35750=AXIS2_PLACEMENT_3D('',#78689,#42345,#42346);
#35751=AXIS2_PLACEMENT_3D('',#78690,#42347,#42348);
#35752=AXIS2_PLACEMENT_3D('',#78691,#42349,#42350);
#35753=AXIS2_PLACEMENT_3D('',#78694,#42351,#42352);
#35754=AXIS2_PLACEMENT_3D('',#78703,#42353,#42354);
#35755=AXIS2_PLACEMENT_3D('',#78712,#42355,#42356);
#35756=AXIS2_PLACEMENT_3D('',#78713,#42357,#42358);
#35757=AXIS2_PLACEMENT_3D('',#78714,#42359,#42360);
#35758=AXIS2_PLACEMENT_3D('',#78717,#42361,#42362);
#35759=AXIS2_PLACEMENT_3D('',#78726,#42363,#42364);
#35760=AXIS2_PLACEMENT_3D('',#78992,#42365,#42366);
#35761=AXIS2_PLACEMENT_3D('',#78993,#42367,#42368);
#35762=AXIS2_PLACEMENT_3D('',#78997,#42370,#42371);
#35763=AXIS2_PLACEMENT_3D('',#78998,#42372,#42373);
#35764=AXIS2_PLACEMENT_3D('',#79136,#42375,#42376);
#35765=AXIS2_PLACEMENT_3D('',#79140,#42378,#42379);
#35766=AXIS2_PLACEMENT_3D('',#79141,#42380,#42381);
#35767=AXIS2_PLACEMENT_3D('',#79142,#42382,#42383);
#35768=AXIS2_PLACEMENT_3D('',#79185,#42385,#42386);
#35769=AXIS2_PLACEMENT_3D('',#79186,#42387,#42388);
#35770=AXIS2_PLACEMENT_3D('',#79188,#42389,#42390);
#35771=AXIS2_PLACEMENT_3D('',#79189,#42391,#42392);
#35772=AXIS2_PLACEMENT_3D('',#79190,#42393,#42394);
#35773=AXIS2_PLACEMENT_3D('',#79192,#42395,#42396);
#35774=AXIS2_PLACEMENT_3D('',#79193,#42397,#42398);
#35775=AXIS2_PLACEMENT_3D('',#79252,#42399,#42400);
#35776=AXIS2_PLACEMENT_3D('',#79353,#42401,#42402);
#35777=AXIS2_PLACEMENT_3D('',#79377,#42403,#42404);
#35778=AXIS2_PLACEMENT_3D('',#79378,#42405,#42406);
#35779=AXIS2_PLACEMENT_3D('',#79381,#42407,#42408);
#35780=AXIS2_PLACEMENT_3D('',#79393,#42409,#42410);
#35781=AXIS2_PLACEMENT_3D('',#79430,#42411,#42412);
#35782=AXIS2_PLACEMENT_3D('',#79432,#42413,#42414);
#35783=AXIS2_PLACEMENT_3D('',#79503,#42415,#42416);
#35784=AXIS2_PLACEMENT_3D('',#79589,#42417,#42418);
#35785=AXIS2_PLACEMENT_3D('',#79660,#42419,#42420);
#35786=AXIS2_PLACEMENT_3D('',#79662,#42421,#42422);
#35787=AXIS2_PLACEMENT_3D('',#79699,#42423,#42424);
#35788=AXIS2_PLACEMENT_3D('',#79709,#42425,#42426);
#35789=AXIS2_PLACEMENT_3D('',#79710,#42427,#42428);
#35790=AXIS2_PLACEMENT_3D('',#79711,#42429,#42430);
#35791=AXIS2_PLACEMENT_3D('',#79712,#42431,#42432);
#35792=AXIS2_PLACEMENT_3D('',#79713,#42433,#42434);
#35793=AXIS2_PLACEMENT_3D('',#79750,#42435,#42436);
#35794=AXIS2_PLACEMENT_3D('',#79751,#42437,#42438);
#35795=AXIS2_PLACEMENT_3D('',#79753,#42439,#42440);
#35796=AXIS2_PLACEMENT_3D('',#79754,#42441,#42442);
#35797=AXIS2_PLACEMENT_3D('',#79757,#42444,#42445);
#35798=AXIS2_PLACEMENT_3D('',#79758,#42446,#42447);
#35799=AXIS2_PLACEMENT_3D('',#79761,#42448,#42449);
#35800=AXIS2_PLACEMENT_3D('',#79765,#42451,#42452);
#35801=AXIS2_PLACEMENT_3D('',#79769,#42454,#42455);
#35802=AXIS2_PLACEMENT_3D('',#79773,#42457,#42458);
#35803=AXIS2_PLACEMENT_3D('',#79775,#42460,#42461);
#35804=AXIS2_PLACEMENT_3D('',#79777,#42462,#42463);
#35805=AXIS2_PLACEMENT_3D('',#79780,#42465,#42466);
#35806=AXIS2_PLACEMENT_3D('',#79781,#42467,#42468);
#35807=AXIS2_PLACEMENT_3D('',#79783,#42469,#42470);
#35808=AXIS2_PLACEMENT_3D('',#79784,#42471,#42472);
#35809=AXIS2_PLACEMENT_3D('',#79785,#42473,#42474);
#35810=AXIS2_PLACEMENT_3D('',#79787,#42475,#42476);
#35811=AXIS2_PLACEMENT_3D('',#79799,#42478,#42479);
#35812=AXIS2_PLACEMENT_3D('',#79800,#42480,#42481);
#35813=AXIS2_PLACEMENT_3D('',#79801,#42482,#42483);
#35814=AXIS2_PLACEMENT_3D('',#79803,#42484,#42485);
#35815=AXIS2_PLACEMENT_3D('',#79815,#42487,#42488);
#35816=AXIS2_PLACEMENT_3D('',#79816,#42489,#42490);
#35817=AXIS2_PLACEMENT_3D('',#79817,#42491,#42492);
#35818=AXIS2_PLACEMENT_3D('',#79819,#42493,#42494);
#35819=AXIS2_PLACEMENT_3D('',#79821,#42496,#42497);
#35820=AXIS2_PLACEMENT_3D('',#79876,#42498,#42499);
#35821=AXIS2_PLACEMENT_3D('',#79878,#42500,#42501);
#35822=AXIS2_PLACEMENT_3D('',#79879,#42502,#42503);
#35823=AXIS2_PLACEMENT_3D('',#79880,#42504,#42505);
#35824=AXIS2_PLACEMENT_3D('',#79960,#42509,#42510);
#35825=AXIS2_PLACEMENT_3D('',#79961,#42511,#42512);
#35826=AXIS2_PLACEMENT_3D('',#79964,#42514,#42515);
#35827=AXIS2_PLACEMENT_3D('',#79965,#42516,#42517);
#35828=AXIS2_PLACEMENT_3D('',#79969,#42520,#42521);
#35829=AXIS2_PLACEMENT_3D('',#79971,#42522,#42523);
#35830=AXIS2_PLACEMENT_3D('',#79973,#42525,#42526);
#35831=AXIS2_PLACEMENT_3D('',#79977,#42529,#42530);
#35832=AXIS2_PLACEMENT_3D('',#79979,#42531,#42532);
#35833=AXIS2_PLACEMENT_3D('',#80018,#42534,#42535);
#35834=AXIS2_PLACEMENT_3D('',#80029,#42536,#42537);
#35835=AXIS2_PLACEMENT_3D('',#80130,#42542,#42543);
#35836=AXIS2_PLACEMENT_3D('',#80138,#42544,#42545);
#35837=AXIS2_PLACEMENT_3D('',#80198,#42546,#42547);
#35838=AXIS2_PLACEMENT_3D('',#80208,#42548,#42549);
#35839=AXIS2_PLACEMENT_3D('',#80211,#42550,#42551);
#35840=AXIS2_PLACEMENT_3D('',#80224,#42554,#42555);
#35841=AXIS2_PLACEMENT_3D('',#80234,#42556,#42557);
#35842=AXIS2_PLACEMENT_3D('',#80236,#42558,#42559);
#35843=AXIS2_PLACEMENT_3D('',#80239,#42561,#42562);
#35844=AXIS2_PLACEMENT_3D('',#80240,#42563,#42564);
#35845=AXIS2_PLACEMENT_3D('',#80242,#42565,#42566);
#35846=AXIS2_PLACEMENT_3D('',#80244,#42568,#42569);
#35847=AXIS2_PLACEMENT_3D('',#80246,#42570,#42571);
#35848=AXIS2_PLACEMENT_3D('',#80247,#42572,#42573);
#35849=AXIS2_PLACEMENT_3D('',#80248,#42574,#42575);
#35850=AXIS2_PLACEMENT_3D('',#80250,#42576,#42577);
#35851=AXIS2_PLACEMENT_3D('',#80252,#42579,#42580);
#35852=AXIS2_PLACEMENT_3D('',#80254,#42581,#42582);
#35853=AXIS2_PLACEMENT_3D('',#80255,#42583,#42584);
#35854=AXIS2_PLACEMENT_3D('',#80256,#42585,#42586);
#35855=AXIS2_PLACEMENT_3D('',#80258,#42587,#42588);
#35856=AXIS2_PLACEMENT_3D('',#80260,#42590,#42591);
#35857=AXIS2_PLACEMENT_3D('',#80262,#42592,#42593);
#35858=AXIS2_PLACEMENT_3D('',#80263,#42594,#42595);
#35859=AXIS2_PLACEMENT_3D('',#80318,#42596,#42597);
#35860=AXIS2_PLACEMENT_3D('',#80319,#42598,#42599);
#35861=AXIS2_PLACEMENT_3D('',#80321,#42600,#42601);
#35862=AXIS2_PLACEMENT_3D('',#80323,#42603,#42604);
#35863=AXIS2_PLACEMENT_3D('',#80327,#42606,#42607);
#35864=AXIS2_PLACEMENT_3D('',#80328,#42608,#42609);
#35865=AXIS2_PLACEMENT_3D('',#80329,#42610,#42611);
#35866=AXIS2_PLACEMENT_3D('',#80331,#42612,#42613);
#35867=AXIS2_PLACEMENT_3D('',#80333,#42614,#42615);
#35868=AXIS2_PLACEMENT_3D('',#80335,#42617,#42618);
#35869=AXIS2_PLACEMENT_3D('',#80337,#42619,#42620);
#35870=AXIS2_PLACEMENT_3D('',#80339,#42622,#42623);
#35871=AXIS2_PLACEMENT_3D('',#80457,#42628,#42629);
#35872=AXIS2_PLACEMENT_3D('',#80458,#42630,#42631);
#35873=AXIS2_PLACEMENT_3D('',#80461,#42633,#42634);
#35874=AXIS2_PLACEMENT_3D('',#80462,#42635,#42636);
#35875=AXIS2_PLACEMENT_3D('',#80465,#42637,#42638);
#35876=AXIS2_PLACEMENT_3D('',#80466,#42639,#42640);
#35877=AXIS2_PLACEMENT_3D('',#80467,#42641,#42642);
#35878=AXIS2_PLACEMENT_3D('',#80468,#42643,#42644);
#35879=AXIS2_PLACEMENT_3D('',#80469,#42645,#42646);
#35880=AXIS2_PLACEMENT_3D('',#80470,#42647,#42648);
#35881=AXIS2_PLACEMENT_3D('',#80472,#42649,#42650);
#35882=AXIS2_PLACEMENT_3D('',#80473,#42651,#42652);
#35883=AXIS2_PLACEMENT_3D('',#80474,#42653,#42654);
#35884=AXIS2_PLACEMENT_3D('',#80479,#42656,#42657);
#35885=AXIS2_PLACEMENT_3D('',#80487,#42661,#42662);
#35886=AXIS2_PLACEMENT_3D('',#80495,#42666,#42667);
#35887=AXIS2_PLACEMENT_3D('',#80499,#42669,#42670);
#35888=AXIS2_PLACEMENT_3D('',#80503,#42672,#42673);
#35889=AXIS2_PLACEMENT_3D('',#80507,#42675,#42676);
#35890=AXIS2_PLACEMENT_3D('',#80511,#42678,#42679);
#35891=AXIS2_PLACEMENT_3D('',#80513,#42680,#42681);
#35892=AXIS2_PLACEMENT_3D('',#80517,#42683,#42684);
#35893=AXIS2_PLACEMENT_3D('',#80521,#42686,#42687);
#35894=AXIS2_PLACEMENT_3D('',#80524,#42689,#42690);
#35895=AXIS2_PLACEMENT_3D('',#80528,#42692,#42693);
#35896=AXIS2_PLACEMENT_3D('',#80532,#42695,#42696);
#35897=AXIS2_PLACEMENT_3D('',#80534,#42697,#42698);
#35898=AXIS2_PLACEMENT_3D('',#80538,#42700,#42701);
#35899=AXIS2_PLACEMENT_3D('',#80540,#42703,#42704);
#35900=AXIS2_PLACEMENT_3D('',#80541,#42705,#42706);
#35901=AXIS2_PLACEMENT_3D('',#80542,#42707,#42708);
#35902=AXIS2_PLACEMENT_3D('',#80544,#42709,#42710);
#35903=AXIS2_PLACEMENT_3D('',#80546,#42711,#42712);
#35904=AXIS2_PLACEMENT_3D('',#80547,#42713,#42714);
#35905=AXIS2_PLACEMENT_3D('',#80548,#42715,#42716);
#35906=AXIS2_PLACEMENT_3D('',#80550,#42717,#42718);
#35907=AXIS2_PLACEMENT_3D('',#80553,#42720,#42721);
#35908=AXIS2_PLACEMENT_3D('',#80554,#42722,#42723);
#35909=AXIS2_PLACEMENT_3D('',#80556,#42724,#42725);
#35910=AXIS2_PLACEMENT_3D('',#80560,#42727,#42728);
#35911=AXIS2_PLACEMENT_3D('',#80563,#42730,#42731);
#35912=AXIS2_PLACEMENT_3D('',#80564,#42732,#42733);
#35913=AXIS2_PLACEMENT_3D('',#80565,#42734,#42735);
#35914=AXIS2_PLACEMENT_3D('',#80566,#42736,#42737);
#35915=AXIS2_PLACEMENT_3D('',#80572,#42741,#42742);
#35916=AXIS2_PLACEMENT_3D('',#80573,#42743,#42744);
#35917=AXIS2_PLACEMENT_3D('',#80574,#42745,#42746);
#35918=AXIS2_PLACEMENT_3D('',#80575,#42747,#42748);
#35919=AXIS2_PLACEMENT_3D('',#80576,#42749,#42750);
#35920=AXIS2_PLACEMENT_3D('',#80577,#42751,#42752);
#35921=AXIS2_PLACEMENT_3D('',#80578,#42753,#42754);
#35922=AXIS2_PLACEMENT_3D('',#80579,#42755,#42756);
#35923=AXIS2_PLACEMENT_3D('',#80581,#42757,#42758);
#35924=AXIS2_PLACEMENT_3D('',#80584,#42760,#42761);
#35925=AXIS2_PLACEMENT_3D('',#80585,#42762,#42763);
#35926=AXIS2_PLACEMENT_3D('',#80586,#42764,#42765);
#35927=AXIS2_PLACEMENT_3D('',#80587,#42766,#42767);
#35928=AXIS2_PLACEMENT_3D('',#80588,#42768,#42769);
#35929=AXIS2_PLACEMENT_3D('',#80589,#42770,#42771);
#35930=AXIS2_PLACEMENT_3D('',#80590,#42772,#42773);
#35931=AXIS2_PLACEMENT_3D('',#80592,#42774,#42775);
#35932=AXIS2_PLACEMENT_3D('',#80595,#42777,#42778);
#35933=AXIS2_PLACEMENT_3D('',#80596,#42779,#42780);
#35934=AXIS2_PLACEMENT_3D('',#80598,#42781,#42782);
#35935=AXIS2_PLACEMENT_3D('',#80599,#42783,#42784);
#35936=AXIS2_PLACEMENT_3D('',#80600,#42785,#42786);
#35937=AXIS2_PLACEMENT_3D('',#80602,#42787,#42788);
#35938=AXIS2_PLACEMENT_3D('',#80604,#42790,#42791);
#35939=AXIS2_PLACEMENT_3D('',#80606,#42792,#42793);
#35940=AXIS2_PLACEMENT_3D('',#80607,#42794,#42795);
#35941=AXIS2_PLACEMENT_3D('',#80608,#42796,#42797);
#35942=AXIS2_PLACEMENT_3D('',#80610,#42798,#42799);
#35943=AXIS2_PLACEMENT_3D('',#80611,#42800,#42801);
#35944=AXIS2_PLACEMENT_3D('',#80612,#42802,#42803);
#35945=AXIS2_PLACEMENT_3D('',#80614,#42804,#42805);
#35946=AXIS2_PLACEMENT_3D('',#80616,#42806,#42807);
#35947=AXIS2_PLACEMENT_3D('',#80618,#42809,#42810);
#35948=AXIS2_PLACEMENT_3D('',#80619,#42811,#42812);
#35949=AXIS2_PLACEMENT_3D('',#80620,#42813,#42814);
#35950=AXIS2_PLACEMENT_3D('',#80621,#42815,#42816);
#35951=AXIS2_PLACEMENT_3D('',#80622,#42817,#42818);
#35952=AXIS2_PLACEMENT_3D('',#80623,#42819,#42820);
#35953=AXIS2_PLACEMENT_3D('',#80624,#42821,#42822);
#35954=AXIS2_PLACEMENT_3D('',#80626,#42823,#42824);
#35955=AXIS2_PLACEMENT_3D('',#80628,#42826,#42827);
#35956=AXIS2_PLACEMENT_3D('',#80630,#42828,#42829);
#35957=AXIS2_PLACEMENT_3D('',#80631,#42830,#42831);
#35958=AXIS2_PLACEMENT_3D('',#80632,#42832,#42833);
#35959=AXIS2_PLACEMENT_3D('',#80634,#42834,#42835);
#35960=AXIS2_PLACEMENT_3D('',#80636,#42837,#42838);
#35961=AXIS2_PLACEMENT_3D('',#80638,#42839,#42840);
#35962=AXIS2_PLACEMENT_3D('',#80640,#42841,#42842);
#35963=AXIS2_PLACEMENT_3D('',#80641,#42843,#42844);
#35964=AXIS2_PLACEMENT_3D('',#80642,#42845,#42846);
#35965=AXIS2_PLACEMENT_3D('',#80644,#42847,#42848);
#35966=AXIS2_PLACEMENT_3D('',#80645,#42849,#42850);
#35967=AXIS2_PLACEMENT_3D('',#80646,#42851,#42852);
#35968=AXIS2_PLACEMENT_3D('',#80648,#42853,#42854);
#35969=AXIS2_PLACEMENT_3D('',#80650,#42856,#42857);
#35970=AXIS2_PLACEMENT_3D('',#80652,#42858,#42859);
#35971=AXIS2_PLACEMENT_3D('',#80653,#42860,#42861);
#35972=AXIS2_PLACEMENT_3D('',#80654,#42862,#42863);
#35973=AXIS2_PLACEMENT_3D('',#80656,#42864,#42865);
#35974=AXIS2_PLACEMENT_3D('',#80658,#42867,#42868);
#35975=AXIS2_PLACEMENT_3D('',#80660,#42869,#42870);
#35976=AXIS2_PLACEMENT_3D('',#80661,#42871,#42872);
#35977=AXIS2_PLACEMENT_3D('',#80662,#42873,#42874);
#35978=AXIS2_PLACEMENT_3D('',#80664,#42875,#42876);
#35979=AXIS2_PLACEMENT_3D('',#80666,#42878,#42879);
#35980=AXIS2_PLACEMENT_3D('',#80668,#42880,#42881);
#35981=AXIS2_PLACEMENT_3D('',#80669,#42882,#42883);
#35982=AXIS2_PLACEMENT_3D('',#80670,#42884,#42885);
#35983=AXIS2_PLACEMENT_3D('',#80672,#42886,#42887);
#35984=AXIS2_PLACEMENT_3D('',#80674,#42889,#42890);
#35985=AXIS2_PLACEMENT_3D('',#80676,#42891,#42892);
#35986=AXIS2_PLACEMENT_3D('',#80677,#42893,#42894);
#35987=AXIS2_PLACEMENT_3D('',#80678,#42895,#42896);
#35988=AXIS2_PLACEMENT_3D('',#80680,#42897,#42898);
#35989=AXIS2_PLACEMENT_3D('',#80682,#42900,#42901);
#35990=AXIS2_PLACEMENT_3D('',#80684,#42902,#42903);
#35991=AXIS2_PLACEMENT_3D('',#80686,#42904,#42905);
#35992=AXIS2_PLACEMENT_3D('',#80688,#42907,#42908);
#35993=AXIS2_PLACEMENT_3D('',#80690,#42909,#42910);
#35994=AXIS2_PLACEMENT_3D('',#80692,#42911,#42912);
#35995=AXIS2_PLACEMENT_3D('',#80694,#42914,#42915);
#35996=AXIS2_PLACEMENT_3D('',#80696,#42916,#42917);
#35997=AXIS2_PLACEMENT_3D('',#80697,#42918,#42919);
#35998=AXIS2_PLACEMENT_3D('',#80698,#42920,#42921);
#35999=AXIS2_PLACEMENT_3D('',#80700,#42922,#42923);
#36000=AXIS2_PLACEMENT_3D('',#80702,#42925,#42926);
#36001=AXIS2_PLACEMENT_3D('',#80704,#42927,#42928);
#36002=AXIS2_PLACEMENT_3D('',#80706,#42929,#42930);
#36003=AXIS2_PLACEMENT_3D('',#80708,#42932,#42933);
#36004=AXIS2_PLACEMENT_3D('',#80710,#42934,#42935);
#36005=AXIS2_PLACEMENT_3D('',#80712,#42936,#42937);
#36006=AXIS2_PLACEMENT_3D('',#80714,#42939,#42940);
#36007=AXIS2_PLACEMENT_3D('',#80716,#42941,#42942);
#36008=AXIS2_PLACEMENT_3D('',#80717,#42943,#42944);
#36009=AXIS2_PLACEMENT_3D('',#80718,#42945,#42946);
#36010=AXIS2_PLACEMENT_3D('',#80720,#42948,#42949);
#36011=AXIS2_PLACEMENT_3D('',#80723,#42950,#42951);
#36012=AXIS2_PLACEMENT_3D('',#80724,#42952,#42953);
#36013=AXIS2_PLACEMENT_3D('',#80725,#42954,#42955);
#36014=AXIS2_PLACEMENT_3D('',#80726,#42956,#42957);
#36015=AXIS2_PLACEMENT_3D('',#80727,#42958,#42959);
#36016=AXIS2_PLACEMENT_3D('',#80728,#42960,#42961);
#36017=AXIS2_PLACEMENT_3D('',#80730,#42962,#42963);
#36018=AXIS2_PLACEMENT_3D('',#80732,#42964,#42965);
#36019=AXIS2_PLACEMENT_3D('',#80733,#42966,#42967);
#36020=AXIS2_PLACEMENT_3D('',#80734,#42968,#42969);
#36021=AXIS2_PLACEMENT_3D('',#80737,#42972,#42973);
#36022=AXIS2_PLACEMENT_3D('',#80739,#42974,#42975);
#36023=AXIS2_PLACEMENT_3D('',#80741,#42976,#42977);
#36024=AXIS2_PLACEMENT_3D('',#80742,#42978,#42979);
#36025=AXIS2_PLACEMENT_3D('',#80743,#42980,#42981);
#36026=AXIS2_PLACEMENT_3D('',#80747,#42983,#42984);
#36027=AXIS2_PLACEMENT_3D('',#80749,#42986,#42987);
#36028=AXIS2_PLACEMENT_3D('',#80751,#42988,#42989);
#36029=AXIS2_PLACEMENT_3D('',#80753,#42990,#42991);
#36030=AXIS2_PLACEMENT_3D('',#80760,#42992,#42993);
#36031=AXIS2_PLACEMENT_3D('',#80763,#42996,#42997);
#36032=AXIS2_PLACEMENT_3D('',#80776,#42998,#42999);
#36033=AXIS2_PLACEMENT_3D('',#80777,#43000,#43001);
#36034=AXIS2_PLACEMENT_3D('',#80778,#43002,#43003);
#36035=AXIS2_PLACEMENT_3D('',#80782,#43005,#43006);
#36036=AXIS2_PLACEMENT_3D('',#80784,#43008,#43009);
#36037=AXIS2_PLACEMENT_3D('',#80786,#43010,#43011);
#36038=AXIS2_PLACEMENT_3D('',#80787,#43012,#43013);
#36039=AXIS2_PLACEMENT_3D('',#80788,#43014,#43015);
#36040=AXIS2_PLACEMENT_3D('',#80790,#43017,#43018);
#36041=AXIS2_PLACEMENT_3D('',#80823,#43019,#43020);
#36042=AXIS2_PLACEMENT_3D('',#80824,#43021,#43022);
#36043=AXIS2_PLACEMENT_3D('',#80825,#43023,#43024);
#36044=AXIS2_PLACEMENT_3D('',#80826,#43025,#43026);
#36045=AXIS2_PLACEMENT_3D('',#80827,#43027,#43028);
#36046=AXIS2_PLACEMENT_3D('',#80877,#43029,#43030);
#36047=AXIS2_PLACEMENT_3D('',#80879,#43032,#43033);
#36048=AXIS2_PLACEMENT_3D('',#80880,#43034,#43035);
#36049=AXIS2_PLACEMENT_3D('',#80882,#43036,#43037);
#36050=AXIS2_PLACEMENT_3D('',#80883,#43038,#43039);
#36051=AXIS2_PLACEMENT_3D('',#80884,#43040,#43041);
#36052=AXIS2_PLACEMENT_3D('',#80886,#43043,#43044);
#36053=AXIS2_PLACEMENT_3D('',#80892,#43048,#43049);
#36054=AXIS2_PLACEMENT_3D('',#80895,#43051,#43052);
#36055=AXIS2_PLACEMENT_3D('',#80896,#43053,#43054);
#36056=AXIS2_PLACEMENT_3D('',#80898,#43055,#43056);
#36057=AXIS2_PLACEMENT_3D('',#80900,#43057,#43058);
#36058=AXIS2_PLACEMENT_3D('',#80901,#43059,#43060);
#36059=AXIS2_PLACEMENT_3D('',#80902,#43061,#43062);
#36060=AXIS2_PLACEMENT_3D('',#81067,#43066,#43067);
#36061=AXIS2_PLACEMENT_3D('',#81068,#43068,#43069);
#36062=AXIS2_PLACEMENT_3D('',#81238,#43070,#43071);
#36063=AXIS2_PLACEMENT_3D('',#81239,#43072,#43073);
#36064=AXIS2_PLACEMENT_3D('',#81240,#43074,#43075);
#36065=AXIS2_PLACEMENT_3D('',#81241,#43076,#43077);
#36066=AXIS2_PLACEMENT_3D('',#81379,#43079,#43080);
#36067=AXIS2_PLACEMENT_3D('',#81381,#43082,#43083);
#36068=AXIS2_PLACEMENT_3D('',#81383,#43085,#43086);
#36069=AXIS2_PLACEMENT_3D('',#81384,#43087,#43088);
#36070=AXIS2_PLACEMENT_3D('',#81521,#43089,#43090);
#36071=AXIS2_PLACEMENT_3D('',#81647,#43092,#43093);
#36072=AXIS2_PLACEMENT_3D('',#81650,#43095,#43096);
#36073=AXIS2_PLACEMENT_3D('',#81651,#43097,#43098);
#36074=AXIS2_PLACEMENT_3D('',#81655,#43101,#43102);
#36075=AXIS2_PLACEMENT_3D('',#81658,#43104,#43105);
#36076=AXIS2_PLACEMENT_3D('',#81659,#43106,#43107);
#36077=AXIS2_PLACEMENT_3D('',#81663,#43110,#43111);
#36078=AXIS2_PLACEMENT_3D('',#81666,#43113,#43114);
#36079=AXIS2_PLACEMENT_3D('',#81667,#43115,#43116);
#36080=AXIS2_PLACEMENT_3D('',#81671,#43119,#43120);
#36081=AXIS2_PLACEMENT_3D('',#81674,#43122,#43123);
#36082=AXIS2_PLACEMENT_3D('',#81675,#43124,#43125);
#36083=AXIS2_PLACEMENT_3D('',#81679,#43128,#43129);
#36084=AXIS2_PLACEMENT_3D('',#81682,#43131,#43132);
#36085=AXIS2_PLACEMENT_3D('',#81683,#43133,#43134);
#36086=AXIS2_PLACEMENT_3D('',#81687,#43137,#43138);
#36087=AXIS2_PLACEMENT_3D('',#81688,#43139,#43140);
#36088=AXIS2_PLACEMENT_3D('',#81689,#43141,#43142);
#36089=AXIS2_PLACEMENT_3D('',#81695,#43146,#43147);
#36090=AXIS2_PLACEMENT_3D('',#81696,#43148,#43149);
#36091=AXIS2_PLACEMENT_3D('',#81697,#43150,#43151);
#36092=AXIS2_PLACEMENT_3D('',#81703,#43155,#43156);
#36093=AXIS2_PLACEMENT_3D('',#81706,#43158,#43159);
#36094=AXIS2_PLACEMENT_3D('',#81707,#43160,#43161);
#36095=AXIS2_PLACEMENT_3D('',#81711,#43164,#43165);
#36096=AXIS2_PLACEMENT_3D('',#81712,#43166,#43167);
#36097=AXIS2_PLACEMENT_3D('',#81713,#43168,#43169);
#36098=AXIS2_PLACEMENT_3D('',#81719,#43173,#43174);
#36099=AXIS2_PLACEMENT_3D('',#81720,#43175,#43176);
#36100=AXIS2_PLACEMENT_3D('',#81721,#43177,#43178);
#36101=AXIS2_PLACEMENT_3D('',#81727,#43182,#43183);
#36102=AXIS2_PLACEMENT_3D('',#81730,#43185,#43186);
#36103=AXIS2_PLACEMENT_3D('',#81731,#43187,#43188);
#36104=AXIS2_PLACEMENT_3D('',#81733,#43190,#43191);
#36105=AXIS2_PLACEMENT_3D('',#81735,#43192,#43193);
#36106=AXIS2_PLACEMENT_3D('',#81737,#43195,#43196);
#36107=AXIS2_PLACEMENT_3D('',#81739,#43197,#43198);
#36108=AXIS2_PLACEMENT_3D('',#81741,#43199,#43200);
#36109=AXIS2_PLACEMENT_3D('',#81742,#43201,#43202);
#36110=AXIS2_PLACEMENT_3D('',#81810,#43203,#43204);
#36111=AXIS2_PLACEMENT_3D('',#81812,#43205,#43206);
#36112=AXIS2_PLACEMENT_3D('',#81814,#43208,#43209);
#36113=AXIS2_PLACEMENT_3D('',#81816,#43210,#43211);
#36114=AXIS2_PLACEMENT_3D('',#81818,#43212,#43213);
#36115=AXIS2_PLACEMENT_3D('',#81819,#43214,#43215);
#36116=AXIS2_PLACEMENT_3D('',#81820,#43216,#43217);
#36117=AXIS2_PLACEMENT_3D('',#81824,#43219,#43220);
#36118=AXIS2_PLACEMENT_3D('',#81828,#43222,#43223);
#36119=AXIS2_PLACEMENT_3D('',#81830,#43224,#43225);
#36120=AXIS2_PLACEMENT_3D('',#81832,#43226,#43227);
#36121=AXIS2_PLACEMENT_3D('',#81836,#43229,#43230);
#36122=AXIS2_PLACEMENT_3D('',#81839,#43232,#43233);
#36123=AXIS2_PLACEMENT_3D('',#81841,#43234,#43235);
#36124=AXIS2_PLACEMENT_3D('',#81888,#43236,#43237);
#36125=AXIS2_PLACEMENT_3D('',#81891,#43239,#43240);
#36126=AXIS2_PLACEMENT_3D('',#81892,#43241,#43242);
#36127=AXIS2_PLACEMENT_3D('',#81894,#43243,#43244);
#36128=AXIS2_PLACEMENT_3D('',#81896,#43245,#43246);
#36129=AXIS2_PLACEMENT_3D('',#81897,#43247,#43248);
#36130=AXIS2_PLACEMENT_3D('',#81965,#43249,#43250);
#36131=AXIS2_PLACEMENT_3D('',#82012,#43251,#43252);
#36132=AXIS2_PLACEMENT_3D('',#82013,#43253,#43254);
#36133=AXIS2_PLACEMENT_3D('',#82015,#43255,#43256);
#36134=AXIS2_PLACEMENT_3D('',#82017,#43257,#43258);
#36135=AXIS2_PLACEMENT_3D('',#82019,#43260,#43261);
#36136=AXIS2_PLACEMENT_3D('',#82021,#43262,#43263);
#36137=AXIS2_PLACEMENT_3D('',#82022,#43264,#43265);
#36138=AXIS2_PLACEMENT_3D('',#82023,#43266,#43267);
#36139=AXIS2_PLACEMENT_3D('',#82025,#43268,#43269);
#36140=AXIS2_PLACEMENT_3D('',#82027,#43271,#43272);
#36141=AXIS2_PLACEMENT_3D('',#82029,#43273,#43274);
#36142=AXIS2_PLACEMENT_3D('',#82030,#43275,#43276);
#36143=AXIS2_PLACEMENT_3D('',#82031,#43277,#43278);
#36144=AXIS2_PLACEMENT_3D('',#82033,#43279,#43280);
#36145=AXIS2_PLACEMENT_3D('',#82034,#43281,#43282);
#36146=AXIS2_PLACEMENT_3D('',#82035,#43283,#43284);
#36147=AXIS2_PLACEMENT_3D('',#82037,#43285,#43286);
#36148=AXIS2_PLACEMENT_3D('',#82039,#43288,#43289);
#36149=AXIS2_PLACEMENT_3D('',#82041,#43290,#43291);
#36150=AXIS2_PLACEMENT_3D('',#82042,#43292,#43293);
#36151=AXIS2_PLACEMENT_3D('',#82043,#43294,#43295);
#36152=AXIS2_PLACEMENT_3D('',#82045,#43296,#43297);
#36153=AXIS2_PLACEMENT_3D('',#82047,#43299,#43300);
#36154=AXIS2_PLACEMENT_3D('',#82049,#43301,#43302);
#36155=AXIS2_PLACEMENT_3D('',#82050,#43303,#43304);
#36156=AXIS2_PLACEMENT_3D('',#82051,#43305,#43306);
#36157=AXIS2_PLACEMENT_3D('',#82053,#43307,#43308);
#36158=AXIS2_PLACEMENT_3D('',#82055,#43310,#43311);
#36159=AXIS2_PLACEMENT_3D('',#82057,#43312,#43313);
#36160=AXIS2_PLACEMENT_3D('',#82058,#43314,#43315);
#36161=AXIS2_PLACEMENT_3D('',#82059,#43316,#43317);
#36162=AXIS2_PLACEMENT_3D('',#82061,#43318,#43319);
#36163=AXIS2_PLACEMENT_3D('',#82063,#43321,#43322);
#36164=AXIS2_PLACEMENT_3D('',#82065,#43323,#43324);
#36165=AXIS2_PLACEMENT_3D('',#82066,#43325,#43326);
#36166=AXIS2_PLACEMENT_3D('',#82067,#43327,#43328);
#36167=AXIS2_PLACEMENT_3D('',#82069,#43329,#43330);
#36168=AXIS2_PLACEMENT_3D('',#82071,#43332,#43333);
#36169=AXIS2_PLACEMENT_3D('',#82072,#43334,#43335);
#36170=AXIS2_PLACEMENT_3D('',#82073,#43336,#43337);
#36171=AXIS2_PLACEMENT_3D('',#82075,#43338,#43339);
#36172=AXIS2_PLACEMENT_3D('',#82077,#43341,#43342);
#36173=AXIS2_PLACEMENT_3D('',#82078,#43343,#43344);
#36174=AXIS2_PLACEMENT_3D('',#82079,#43345,#43346);
#36175=AXIS2_PLACEMENT_3D('',#82080,#43347,#43348);
#36176=AXIS2_PLACEMENT_3D('',#82082,#43349,#43350);
#36177=AXIS2_PLACEMENT_3D('',#82084,#43352,#43353);
#36178=AXIS2_PLACEMENT_3D('',#82085,#43354,#43355);
#36179=AXIS2_PLACEMENT_3D('',#82087,#43356,#43357);
#36180=AXIS2_PLACEMENT_3D('',#82088,#43358,#43359);
#36181=AXIS2_PLACEMENT_3D('',#82089,#43360,#43361);
#36182=AXIS2_PLACEMENT_3D('',#82091,#43362,#43363);
#36183=AXIS2_PLACEMENT_3D('',#82093,#43365,#43366);
#36184=AXIS2_PLACEMENT_3D('',#82094,#43367,#43368);
#36185=AXIS2_PLACEMENT_3D('',#82095,#43369,#43370);
#36186=AXIS2_PLACEMENT_3D('',#82097,#43371,#43372);
#36187=AXIS2_PLACEMENT_3D('',#82099,#43374,#43375);
#36188=AXIS2_PLACEMENT_3D('',#82100,#43376,#43377);
#36189=AXIS2_PLACEMENT_3D('',#82101,#43378,#43379);
#36190=AXIS2_PLACEMENT_3D('',#82102,#43380,#43381);
#36191=AXIS2_PLACEMENT_3D('',#82104,#43382,#43383);
#36192=AXIS2_PLACEMENT_3D('',#82106,#43385,#43386);
#36193=AXIS2_PLACEMENT_3D('',#82107,#43387,#43388);
#36194=AXIS2_PLACEMENT_3D('',#82109,#43389,#43390);
#36195=AXIS2_PLACEMENT_3D('',#82110,#43391,#43392);
#36196=AXIS2_PLACEMENT_3D('',#82111,#43393,#43394);
#36197=AXIS2_PLACEMENT_3D('',#82113,#43396,#43397);
#36198=AXIS2_PLACEMENT_3D('',#82115,#43398,#43399);
#36199=AXIS2_PLACEMENT_3D('',#82116,#43400,#43401);
#36200=AXIS2_PLACEMENT_3D('',#82117,#43402,#43403);
#36201=AXIS2_PLACEMENT_3D('',#82118,#43404,#43405);
#36202=AXIS2_PLACEMENT_3D('',#82120,#43406,#43407);
#36203=AXIS2_PLACEMENT_3D('',#82124,#43409,#43410);
#36204=AXIS2_PLACEMENT_3D('',#82125,#43411,#43412);
#36205=AXIS2_PLACEMENT_3D('',#82126,#43413,#43414);
#36206=AXIS2_PLACEMENT_3D('',#82130,#43417,#43418);
#36207=AXIS2_PLACEMENT_3D('',#82132,#43419,#43420);
#36208=AXIS2_PLACEMENT_3D('',#82133,#43421,#43422);
#36209=AXIS2_PLACEMENT_3D('',#82134,#43423,#43424);
#36210=AXIS2_PLACEMENT_3D('',#82136,#43425,#43426);
#36211=AXIS2_PLACEMENT_3D('',#82139,#43428,#43429);
#36212=AXIS2_PLACEMENT_3D('',#82140,#43430,#43431);
#36213=AXIS2_PLACEMENT_3D('',#82142,#43432,#43433);
#36214=AXIS2_PLACEMENT_3D('',#82143,#43434,#43435);
#36215=AXIS2_PLACEMENT_3D('',#82144,#43436,#43437);
#36216=AXIS2_PLACEMENT_3D('',#82146,#43438,#43439);
#36217=AXIS2_PLACEMENT_3D('',#82148,#43440,#43441);
#36218=AXIS2_PLACEMENT_3D('',#82149,#43442,#43443);
#36219=AXIS2_PLACEMENT_3D('',#82150,#43444,#43445);
#36220=AXIS2_PLACEMENT_3D('',#82152,#43447,#43448);
#36221=AXIS2_PLACEMENT_3D('',#82154,#43449,#43450);
#36222=AXIS2_PLACEMENT_3D('',#82155,#43451,#43452);
#36223=AXIS2_PLACEMENT_3D('',#82156,#43453,#43454);
#36224=AXIS2_PLACEMENT_3D('',#82158,#43455,#43456);
#36225=AXIS2_PLACEMENT_3D('',#82159,#43457,#43458);
#36226=AXIS2_PLACEMENT_3D('',#82160,#43459,#43460);
#36227=AXIS2_PLACEMENT_3D('',#82162,#43462,#43463);
#36228=AXIS2_PLACEMENT_3D('',#82164,#43464,#43465);
#36229=AXIS2_PLACEMENT_3D('',#82196,#43466,#43467);
#36230=AXIS2_PLACEMENT_3D('',#82198,#43468,#43469);
#36231=AXIS2_PLACEMENT_3D('',#82199,#43470,#43471);
#36232=AXIS2_PLACEMENT_3D('',#82200,#43472,#43473);
#36233=AXIS2_PLACEMENT_3D('',#82202,#43475,#43476);
#36234=AXIS2_PLACEMENT_3D('',#82204,#43477,#43478);
#36235=AXIS2_PLACEMENT_3D('',#82206,#43479,#43480);
#36236=AXIS2_PLACEMENT_3D('',#82207,#43481,#43482);
#36237=AXIS2_PLACEMENT_3D('',#82208,#43483,#43484);
#36238=AXIS2_PLACEMENT_3D('',#82209,#43485,#43486);
#36239=AXIS2_PLACEMENT_3D('',#82210,#43487,#43488);
#36240=AXIS2_PLACEMENT_3D('',#82214,#43491,#43492);
#36241=AXIS2_PLACEMENT_3D('',#82216,#43493,#43494);
#36242=AXIS2_PLACEMENT_3D('',#82218,#43495,#43496);
#36243=AXIS2_PLACEMENT_3D('',#82220,#43497,#43498);
#36244=AXIS2_PLACEMENT_3D('',#82221,#43499,#43500);
#36245=AXIS2_PLACEMENT_3D('',#82222,#43501,#43502);
#36246=AXIS2_PLACEMENT_3D('',#82223,#43503,#43504);
#36247=AXIS2_PLACEMENT_3D('',#82224,#43505,#43506);
#36248=AXIS2_PLACEMENT_3D('',#82225,#43507,#43508);
#36249=AXIS2_PLACEMENT_3D('',#82226,#43509,#43510);
#36250=AXIS2_PLACEMENT_3D('',#82228,#43511,#43512);
#36251=AXIS2_PLACEMENT_3D('',#82230,#43514,#43515);
#36252=AXIS2_PLACEMENT_3D('',#82233,#43517,#43518);
#36253=AXIS2_PLACEMENT_3D('',#82234,#43519,#43520);
#36254=AXIS2_PLACEMENT_3D('',#82236,#43521,#43522);
#36255=AXIS2_PLACEMENT_3D('',#82238,#43523,#43524);
#36256=AXIS2_PLACEMENT_3D('',#82239,#43525,#43526);
#36257=AXIS2_PLACEMENT_3D('',#82240,#43527,#43528);
#36258=AXIS2_PLACEMENT_3D('',#82245,#43531,#43532);
#36259=AXIS2_PLACEMENT_3D('',#82246,#43533,#43534);
#36260=AXIS2_PLACEMENT_3D('',#82248,#43535,#43536);
#36261=AXIS2_PLACEMENT_3D('',#82250,#43537,#43538);
#36262=AXIS2_PLACEMENT_3D('',#82251,#43539,#43540);
#36263=AXIS2_PLACEMENT_3D('',#82252,#43541,#43542);
#36264=AXIS2_PLACEMENT_3D('',#82257,#43545,#43546);
#36265=AXIS2_PLACEMENT_3D('',#82258,#43547,#43548);
#36266=AXIS2_PLACEMENT_3D('',#82259,#43549,#43550);
#36267=AXIS2_PLACEMENT_3D('',#82260,#43551,#43552);
#36268=AXIS2_PLACEMENT_3D('',#82263,#43555,#43556);
#36269=AXIS2_PLACEMENT_3D('',#82265,#43557,#43558);
#36270=AXIS2_PLACEMENT_3D('',#82266,#43559,#43560);
#36271=AXIS2_PLACEMENT_3D('',#82267,#43561,#43562);
#36272=AXIS2_PLACEMENT_3D('',#82269,#43564,#43565);
#36273=AXIS2_PLACEMENT_3D('',#82271,#43566,#43567);
#36274=AXIS2_PLACEMENT_3D('',#82272,#43568,#43569);
#36275=AXIS2_PLACEMENT_3D('',#82273,#43570,#43571);
#36276=AXIS2_PLACEMENT_3D('',#82274,#43572,#43573);
#36277=AXIS2_PLACEMENT_3D('',#82277,#43574,#43575);
#36278=AXIS2_PLACEMENT_3D('',#82279,#43576,#43577);
#36279=AXIS2_PLACEMENT_3D('',#82281,#43578,#43579);
#36280=AXIS2_PLACEMENT_3D('',#82282,#43580,#43581);
#36281=AXIS2_PLACEMENT_3D('',#82283,#43582,#43583);
#36282=AXIS2_PLACEMENT_3D('',#82287,#43585,#43586);
#36283=AXIS2_PLACEMENT_3D('',#82300,#43588,#43589);
#36284=AXIS2_PLACEMENT_3D('',#82302,#43590,#43591);
#36285=AXIS2_PLACEMENT_3D('',#82304,#43592,#43593);
#36286=AXIS2_PLACEMENT_3D('',#82305,#43594,#43595);
#36287=AXIS2_PLACEMENT_3D('',#82306,#43596,#43597);
#36288=AXIS2_PLACEMENT_3D('',#82436,#43600,#43601);
#36289=AXIS2_PLACEMENT_3D('',#82437,#43602,#43603);
#36290=AXIS2_PLACEMENT_3D('',#82439,#43605,#43606);
#36291=AXIS2_PLACEMENT_3D('',#82443,#43608,#43609);
#36292=AXIS2_PLACEMENT_3D('',#82445,#43611,#43612);
#36293=AXIS2_PLACEMENT_3D('',#82448,#43613,#43614);
#36294=AXIS2_PLACEMENT_3D('',#82450,#43615,#43616);
#36295=AXIS2_PLACEMENT_3D('',#82452,#43617,#43618);
#36296=AXIS2_PLACEMENT_3D('',#82453,#43619,#43620);
#36297=AXIS2_PLACEMENT_3D('',#82454,#43621,#43622);
#36298=AXIS2_PLACEMENT_3D('',#82459,#43625,#43626);
#36299=AXIS2_PLACEMENT_3D('',#82460,#43627,#43628);
#36300=AXIS2_PLACEMENT_3D('',#82462,#43629,#43630);
#36301=AXIS2_PLACEMENT_3D('',#82465,#43632,#43633);
#36302=AXIS2_PLACEMENT_3D('',#82469,#43635,#43636);
#36303=AXIS2_PLACEMENT_3D('',#82473,#43638,#43639);
#36304=AXIS2_PLACEMENT_3D('',#82477,#43641,#43642);
#36305=AXIS2_PLACEMENT_3D('',#82480,#43644,#43645);
#36306=AXIS2_PLACEMENT_3D('',#82481,#43646,#43647);
#36307=AXIS2_PLACEMENT_3D('',#82482,#43648,#43649);
#36308=AXIS2_PLACEMENT_3D('',#82483,#43650,#43651);
#36309=AXIS2_PLACEMENT_3D('',#82484,#43652,#43653);
#36310=AXIS2_PLACEMENT_3D('',#82485,#43654,#43655);
#36311=AXIS2_PLACEMENT_3D('',#82486,#43656,#43657);
#36312=AXIS2_PLACEMENT_3D('',#82487,#43658,#43659);
#36313=AXIS2_PLACEMENT_3D('',#82488,#43660,#43661);
#36314=AXIS2_PLACEMENT_3D('',#82538,#43662,#43663);
#36315=AXIS2_PLACEMENT_3D('',#82540,#43665,#43666);
#36316=AXIS2_PLACEMENT_3D('',#82542,#43668,#43669);
#36317=AXIS2_PLACEMENT_3D('',#82544,#43671,#43672);
#36318=AXIS2_PLACEMENT_3D('',#82617,#43676,#43677);
#36319=AXIS2_PLACEMENT_3D('',#82618,#43678,#43679);
#36320=AXIS2_PLACEMENT_3D('',#82619,#43680,#43681);
#36321=AXIS2_PLACEMENT_3D('',#82621,#43682,#43683);
#36322=AXIS2_PLACEMENT_3D('',#82622,#43684,#43685);
#36323=AXIS2_PLACEMENT_3D('',#82623,#43686,#43687);
#36324=AXIS2_PLACEMENT_3D('',#82626,#43689,#43690);
#36325=AXIS2_PLACEMENT_3D('',#82627,#43691,#43692);
#36326=AXIS2_PLACEMENT_3D('',#82629,#43693,#43694);
#36327=AXIS2_PLACEMENT_3D('',#82630,#43695,#43696);
#36328=AXIS2_PLACEMENT_3D('',#82631,#43697,#43698);
#36329=AXIS2_PLACEMENT_3D('',#82634,#43700,#43701);
#36330=AXIS2_PLACEMENT_3D('',#82635,#43702,#43703);
#36331=AXIS2_PLACEMENT_3D('',#82637,#43704,#43705);
#36332=AXIS2_PLACEMENT_3D('',#82638,#43706,#43707);
#36333=AXIS2_PLACEMENT_3D('',#82639,#43708,#43709);
#36334=AXIS2_PLACEMENT_3D('',#82642,#43711,#43712);
#36335=AXIS2_PLACEMENT_3D('',#82643,#43713,#43714);
#36336=AXIS2_PLACEMENT_3D('',#82644,#43715,#43716);
#36337=AXIS2_PLACEMENT_3D('',#82645,#43717,#43718);
#36338=AXIS2_PLACEMENT_3D('',#82666,#43721,#43722);
#36339=AXIS2_PLACEMENT_3D('',#82707,#43725,#43726);
#36340=AXIS2_PLACEMENT_3D('',#82709,#43728,#43729);
#36341=AXIS2_PLACEMENT_3D('',#82711,#43731,#43732);
#36342=AXIS2_PLACEMENT_3D('',#82713,#43734,#43735);
#36343=AXIS2_PLACEMENT_3D('',#82715,#43737,#43738);
#36344=AXIS2_PLACEMENT_3D('',#82716,#43739,#43740);
#36345=AXIS2_PLACEMENT_3D('',#82727,#43741,#43742);
#36346=AXIS2_PLACEMENT_3D('',#82728,#43743,#43744);
#36347=AXIS2_PLACEMENT_3D('',#82729,#43745,#43746);
#36348=AXIS2_PLACEMENT_3D('',#82731,#43747,#43748);
#36349=AXIS2_PLACEMENT_3D('',#82770,#43750,#43751);
#36350=AXIS2_PLACEMENT_3D('',#82912,#43752,#43753);
#36351=AXIS2_PLACEMENT_3D('',#82913,#43754,#43755);
#36352=AXIS2_PLACEMENT_3D('',#82914,#43756,#43757);
#36353=AXIS2_PLACEMENT_3D('',#82916,#43759,#43760);
#36354=AXIS2_PLACEMENT_3D('',#82919,#43762,#43763);
#36355=AXIS2_PLACEMENT_3D('',#82920,#43764,#43765);
#36356=AXIS2_PLACEMENT_3D('',#82923,#43767,#43768);
#36357=AXIS2_PLACEMENT_3D('',#82924,#43769,#43770);
#36358=AXIS2_PLACEMENT_3D('',#82927,#43772,#43773);
#36359=AXIS2_PLACEMENT_3D('',#82928,#43774,#43775);
#36360=AXIS2_PLACEMENT_3D('',#83028,#43776,#43777);
#36361=AXIS2_PLACEMENT_3D('',#83030,#43778,#43779);
#36362=AXIS2_PLACEMENT_3D('',#83165,#43780,#43781);
#36363=AXIS2_PLACEMENT_3D('',#83166,#43782,#43783);
#36364=AXIS2_PLACEMENT_3D('',#83203,#43784,#43785);
#36365=AXIS2_PLACEMENT_3D('',#83240,#43786,#43787);
#36366=AXIS2_PLACEMENT_3D('',#83277,#43788,#43789);
#36367=AXIS2_PLACEMENT_3D('',#83278,#43790,#43791);
#36368=AXIS2_PLACEMENT_3D('',#83280,#43793,#43794);
#42297=DIRECTION('axis',(0.,0.,1.));
#42298=DIRECTION('refdir',(1.,0.,0.));
#42299=DIRECTION('center_axis',(6.63470718431993E-14,0.227955838450084,
-0.973671472169396));
#42300=DIRECTION('ref_axis',(-0.992732772338003,0.117171330149,0.0274321365777));
#42301=DIRECTION('center_axis',(0.406548496485063,0.889574707517134,0.208267039522679));
#42302=DIRECTION('ref_axis',(0.874920124951576,-0.444723758704906,0.191665211757637));
#42303=DIRECTION('center_axis',(2.91433543964118E-16,0.227955838450093,
-0.973671472169394));
#42304=DIRECTION('ref_axis',(1.,-6.06006121796129E-18,2.9789526130602E-16));
#42305=DIRECTION('center_axis',(0.749524872976688,0.644544805048453,0.150912090550531));
#42306=DIRECTION('ref_axis',(-0.160087197730326,-0.0447191178841713,0.986089392306049));
#42307=DIRECTION('center_axis',(6.30625906570168E-14,0.227955838450087,
-0.973671472169396));
#42308=DIRECTION('ref_axis',(-0.662066919314815,0.729712947738079,0.170840300434043));
#42309=DIRECTION('center_axis',(-9.09138157376714E-14,0.502994068288049,
0.864289862989864));
#42310=DIRECTION('ref_axis',(-0.633334126643349,0.668855315522369,-0.389256279238214));
#42311=DIRECTION('center_axis',(-0.596844579943065,-0.693468570092834,0.403581329704418));
#42312=DIRECTION('ref_axis',(0.437619919908321,-0.702944182108675,-0.560676629207069));
#42313=DIRECTION('center_axis',(-0.59683034801759,-0.69347971696906,0.403583222938857));
#42314=DIRECTION('ref_axis',(0.802367306415891,-0.515527629471871,0.300729062190571));
#42315=DIRECTION('center_axis',(0.,0.502994068287953,0.86428986298992));
#42316=DIRECTION('ref_axis',(1.,0.,0.));
#42317=DIRECTION('center_axis',(-0.483245158280883,-0.756672875743816,0.440363799728893));
#42318=DIRECTION('ref_axis',(0.875485075257188,-0.417663891641161,0.243069448144098));
#42319=DIRECTION('center_axis',(-0.483245158280883,-0.756672875743816,0.440363799728893));
#42320=DIRECTION('ref_axis',(0.875485075257188,-0.417663891641161,0.243069448144098));
#42321=DIRECTION('center_axis',(2.41831516884545E-10,0.50299406814986,0.864289863070286));
#42322=DIRECTION('ref_axis',(-0.875472610430908,0.417683408812711,-0.243080806292652));
#42323=DIRECTION('center_axis',(-2.46296037642308E-13,-0.687200931805762,
0.726467397289991));
#42324=DIRECTION('ref_axis',(0.402304300130036,0.66508526660206,0.629136581551056));
#42325=DIRECTION('center_axis',(0.648015366812002,-0.553297373850002,-0.523390963302002));
#42326=DIRECTION('ref_axis',(0.761627260788049,0.470762036932009,0.445316763897474));
#42327=DIRECTION('center_axis',(0.648015366812002,-0.553297373850002,-0.523390963302002));
#42328=DIRECTION('ref_axis',(0.761627260788049,0.470762036932009,0.445316763897474));
#42329=DIRECTION('center_axis',(0.,0.687200931805355,-0.726467397290375));
#42330=DIRECTION('ref_axis',(1.,0.,0.));
#42331=DIRECTION('center_axis',(0.648015366812002,0.553297373850002,0.523390963302002));
#42332=DIRECTION('ref_axis',(0.761627260788049,-0.470762036932009,-0.445316763897474));
#42333=DIRECTION('center_axis',(0.648015366812002,0.553297373850002,0.523390963302002));
#42334=DIRECTION('ref_axis',(0.761627260788049,-0.470762036932009,-0.445316763897474));
#42335=DIRECTION('center_axis',(2.63677968348136E-16,0.687200931805355,
-0.726467397290375));
#42336=DIRECTION('ref_axis',(1.,-8.33708823855768E-17,2.84094538938874E-16));
#42337=DIRECTION('center_axis',(-2.04246620832741E-13,-0.502994068288093,
-0.864289862989838));
#42338=DIRECTION('ref_axis',(0.784944791291048,0.535484366527033,-0.311637879325019));
#42339=DIRECTION('center_axis',(-0.596850310252312,0.693464160284547,-0.403580432568982));
#42340=DIRECTION('ref_axis',(-0.802352586377076,-0.51573478711129,0.300412976579389));
#42341=DIRECTION('center_axis',(-2.4182864330415E-10,0.502994068149861,
0.864289863070286));
#42342=DIRECTION('ref_axis',(0.802371434083077,0.515829798451751,-0.300199435037263));
#42343=DIRECTION('center_axis',(-0.483245250027863,0.756673054355651,-0.440363392140626));
#42344=DIRECTION('ref_axis',(3.76091608502762E-6,0.50299542602652,0.864289072812016));
#42345=DIRECTION('center_axis',(-0.483247714733613,0.756671625250094,-0.440363143037791));
#42346=DIRECTION('ref_axis',(-0.8754836638776,-0.417653389614233,0.243092575837265));
#42347=DIRECTION('center_axis',(1.38777878077987E-16,0.502994068287953,
0.86428986298992));
#42348=DIRECTION('ref_axis',(1.,-2.40819858205088E-17,-1.46553589810128E-16));
#42349=DIRECTION('center_axis',(7.08949205856751E-14,-0.227955838450084,
0.973671472169396));
#42350=DIRECTION('ref_axis',(0.992732772337252,0.117171330155029,0.027432136579107));
#42351=DIRECTION('center_axis',(0.406568830313121,-0.889565491389124,-0.20826671060793));
#42352=DIRECTION('ref_axis',(-0.220907270377139,0.125476294051318,-0.967189576828488));
#42353=DIRECTION('center_axis',(-8.35086727472959E-14,0.227955838450079,
-0.973671472169397));
#42354=DIRECTION('ref_axis',(0.913629160773151,0.395844764797068,0.0926751248593784));
#42355=DIRECTION('center_axis',(0.749427187004001,-0.644656140376395,-0.150921675230167));
#42356=DIRECTION('ref_axis',(0.634043326955048,0.764428974922688,-0.116779286872384));
#42357=DIRECTION('center_axis',(3.46944695195141E-16,0.227955838450093,
-0.973671472169394));
#42358=DIRECTION('ref_axis',(1.,-6.63936891038671E-18,3.54771832349934E-16));
#42359=DIRECTION('center_axis',(-2.12030478187416E-14,0.950202644287033,
-0.311632692107118));
#42360=DIRECTION('ref_axis',(0.198472765334091,0.305433196953141,0.93129969591943));
#42361=DIRECTION('center_axis',(-5.55111512313038E-16,0.950202644287065,
-0.311632692107021));
#42362=DIRECTION('ref_axis',(1.,5.54555085240923E-16,-9.04006692102742E-17));
#42363=DIRECTION('center_axis',(-5.55111512313038E-16,0.950202644287065,
-0.311632692107021));
#42364=DIRECTION('ref_axis',(1.,5.52729018384727E-16,-9.59685496007145E-17));
#42365=DIRECTION('center_axis',(-0.206241528410022,0.304933168374568,0.929774270876617));
#42366=DIRECTION('ref_axis',(2.47601291321785E-8,-0.950202565004139,0.311632933849352));
#42367=DIRECTION('center_axis',(0.,1.,-7.7733519678E-16));
#42368=DIRECTION('ref_axis',(0.,-7.7733519678E-16,-1.));
#42369=DIRECTION('',(-1.,0.,0.));
#42370=DIRECTION('center_axis',(3.58723488914E-17,1.,-1.34708140773E-15));
#42371=DIRECTION('ref_axis',(1.,-3.58723488914E-17,4.83229742432088E-32));
#42372=DIRECTION('center_axis',(-1.,0.,0.));
#42373=DIRECTION('ref_axis',(0.,-1.,1.0842021724855E-15));
#42374=DIRECTION('',(-1.,0.,0.));
#42375=DIRECTION('center_axis',(0.,0.284628947689001,-0.958637763776001));
#42376=DIRECTION('ref_axis',(-1.,0.,0.));
#42377=DIRECTION('',(1.,0.,0.));
#42378=DIRECTION('center_axis',(1.05471187339E-15,0.284628947689001,-0.958637763776001));
#42379=DIRECTION('ref_axis',(1.,-2.4268872593874E-17,1.09301374232827E-15));
#42380=DIRECTION('center_axis',(-3.33066907388001E-16,0.284628947689001,
-0.958637763776001));
#42381=DIRECTION('ref_axis',(1.,7.90711700759394E-18,-3.45090007399474E-16));
#42382=DIRECTION('center_axis',(-1.,0.,0.));
#42383=DIRECTION('ref_axis',(0.,0.950202644287065,-0.31163269210702));
#42384=DIRECTION('',(1.,0.,0.));
#42385=DIRECTION('center_axis',(0.,0.950202644287065,-0.311632692107021));
#42386=DIRECTION('ref_axis',(-1.,0.,0.));
#42387=DIRECTION('center_axis',(-0.296636433707077,-0.948406798699881,0.111943603557285));
#42388=DIRECTION('ref_axis',(0.387977737402026,-0.0125716202918961,0.921583002037061));
#42389=DIRECTION('center_axis',(-0.424818360062199,-0.867834261877406,-0.257668498008121));
#42390=DIRECTION('ref_axis',(0.90527860957501,-0.407246922701095,-0.1209156027832));
#42391=DIRECTION('center_axis',(-0.391875379580097,-1.2252820670103E-15,
-0.920018307904226));
#42392=DIRECTION('ref_axis',(0.920018307904226,-1.05621218979234E-31,-0.391875379580097));
#42393=DIRECTION('center_axis',(-6.84827429158807E-14,0.284628947688994,
-0.958637763776003));
#42394=DIRECTION('ref_axis',(0.996284914443996,0.0825562971465005,0.0245117737583));
#42395=DIRECTION('center_axis',(-0.193028156853976,-0.94060906825824,-0.279275332551807));
#42396=DIRECTION('ref_axis',(1.51496469073372E-7,-0.284628303088786,0.958637955163875));
#42397=DIRECTION('center_axis',(-4.98308895405631E-6,0.284630761188568,
-0.958637225315388));
#42398=DIRECTION('ref_axis',(0.905278651982129,-0.407245323311114,-0.120920671957466));
#42399=DIRECTION('center_axis',(0.877582561890373,-0.479425538604203,0.));
#42400=DIRECTION('ref_axis',(0.479425538604203,0.877582561890373,0.));
#42401=DIRECTION('center_axis',(3.15330923650249E-6,0.28462980062271,-0.958637510526024));
#42402=DIRECTION('ref_axis',(-0.981193104700328,-0.185043702214525,-0.0549446954607343));
#42403=DIRECTION('center_axis',(5.98055361294049E-17,1.09473299575306E-16,
-1.));
#42404=DIRECTION('ref_axis',(-0.479425538604203,-0.877582561890373,-1.24744160070242E-16));
#42405=DIRECTION('center_axis',(3.58723488914E-17,1.,-1.34708140773E-15));
#42406=DIRECTION('ref_axis',(1.,-3.58723488914E-17,4.83229742432088E-32));
#42407=DIRECTION('center_axis',(8.32667268468611E-17,0.419820362992804,
0.907607218358575));
#42408=DIRECTION('ref_axis',(1.,-5.3020129034611E-18,-8.92906449242453E-17));
#42409=DIRECTION('center_axis',(-1.,-6.06243811038E-15,2.950331972E-15));
#42410=DIRECTION('ref_axis',(6.06243811038E-15,-1.,1.52149577650908E-31));
#42411=DIRECTION('center_axis',(-1.,0.,0.));
#42412=DIRECTION('ref_axis',(0.,1.,0.));
#42413=DIRECTION('center_axis',(3.88578058619201E-16,-0.687200931805355,
0.726467397290375));
#42414=DIRECTION('ref_axis',(1.,1.21921474786958E-16,-4.19555658898608E-16));
#42415=DIRECTION('center_axis',(-1.,3.92975632019E-15,5.94636008283E-15));
#42416=DIRECTION('ref_axis',(-3.92975632019E-15,-1.,5.15343103553154E-31));
#42417=DIRECTION('center_axis',(1.,-8.01620055713E-15,-2.35928728678E-15));
#42418=DIRECTION('ref_axis',(8.01620055713E-15,1.,4.56601977004064E-32));
#42419=DIRECTION('center_axis',(0.,-0.687200931805355,0.726467397290375));
#42420=DIRECTION('ref_axis',(1.,0.,0.));
#42421=DIRECTION('center_axis',(1.,0.,0.));
#42422=DIRECTION('ref_axis',(0.,1.,0.));
#42423=DIRECTION('center_axis',(1.,0.,0.));
#42424=DIRECTION('ref_axis',(0.,1.,0.));
#42425=DIRECTION('center_axis',(0.,0.,1.));
#42426=DIRECTION('ref_axis',(1.,0.,0.));
#42427=DIRECTION('center_axis',(-0.391875379580097,1.25339704769031E-15,
0.920018307904226));
#42428=DIRECTION('ref_axis',(0.920018307904226,2.69771308214058E-31,0.391875379580097));
#42429=DIRECTION('center_axis',(-0.424818360062199,0.867834261877406,0.257668498008121));
#42430=DIRECTION('ref_axis',(0.90527860957501,0.407246922701095,0.1209156027832));
#42431=DIRECTION('center_axis',(2.92163435282501E-13,0.284628947689245,
-0.958637763775929));
#42432=DIRECTION('ref_axis',(-0.752005368733267,-0.631892774094225,-0.187615157820067));
#42433=DIRECTION('center_axis',(-0.193028626051129,0.940608766817842,0.279276023514787));
#42434=DIRECTION('ref_axis',(1.14724600190167E-8,-0.284629003337217,0.958637747253498));
#42435=DIRECTION('center_axis',(-3.34855995114163E-16,1.,-1.24757595645316E-15));
#42436=DIRECTION('ref_axis',(0.965815610620677,0.,-0.259230025809914));
#42437=DIRECTION('center_axis',(1.,0.,0.));
#42438=DIRECTION('ref_axis',(0.,1.,0.));
#42439=DIRECTION('center_axis',(-1.,0.,0.));
#42440=DIRECTION('ref_axis',(0.,1.,0.));
#42441=DIRECTION('center_axis',(1.,0.,0.));
#42442=DIRECTION('ref_axis',(0.,1.,0.));
#42443=DIRECTION('',(1.,0.,0.));
#42444=DIRECTION('center_axis',(1.,0.,0.));
#42445=DIRECTION('ref_axis',(0.,1.,0.));
#42446=DIRECTION('center_axis',(1.,0.,0.));
#42447=DIRECTION('ref_axis',(0.,1.,0.));
#42448=DIRECTION('center_axis',(-1.,0.,0.));
#42449=DIRECTION('ref_axis',(0.,1.,0.));
#42450=DIRECTION('',(0.,-1.,0.));
#42451=DIRECTION('center_axis',(-1.,0.,0.));
#42452=DIRECTION('ref_axis',(0.,1.,0.));
#42453=DIRECTION('',(0.,0.,-1.));
#42454=DIRECTION('center_axis',(-1.,0.,0.));
#42455=DIRECTION('ref_axis',(0.,1.,0.));
#42456=DIRECTION('',(0.,1.,0.));
#42457=DIRECTION('center_axis',(1.,0.,0.));
#42458=DIRECTION('ref_axis',(0.,1.,0.));
#42459=DIRECTION('',(0.,0.901003410349976,-0.433812003680988));
#42460=DIRECTION('center_axis',(8.58451173878204E-29,0.901003410349976,
-0.433812003680988));
#42461=DIRECTION('ref_axis',(-1.,7.73467435283202E-29,-3.724064238024E-29));
#42462=DIRECTION('center_axis',(0.,0.901003410349976,-0.433812003680988));
#42463=DIRECTION('ref_axis',(1.,0.,0.));
#42464=DIRECTION('',(0.,0.901003410349976,-0.433812003680988));
#42465=DIRECTION('center_axis',(-3.70762016608926E-8,0.901003426429784,
-0.433811970284118));
#42466=DIRECTION('ref_axis',(0.707106729560538,0.306751431965231,0.637105667842847));
#42467=DIRECTION('center_axis',(1.,0.,0.));
#42468=DIRECTION('ref_axis',(0.,-0.433812003680988,-0.901003410349975));
#42469=DIRECTION('center_axis',(0.,1.,0.));
#42470=DIRECTION('ref_axis',(1.,0.,0.));
#42471=DIRECTION('center_axis',(1.,0.,0.));
#42472=DIRECTION('ref_axis',(0.,1.,0.));
#42473=DIRECTION('center_axis',(0.,1.,0.));
#42474=DIRECTION('ref_axis',(-1.,0.,0.));
#42475=DIRECTION('center_axis',(0.,1.,-6.12323399574E-17));
#42476=DIRECTION('ref_axis',(1.,0.,0.));
#42477=DIRECTION('',(0.,1.,0.));
#42478=DIRECTION('center_axis',(0.,0.,-1.));
#42479=DIRECTION('ref_axis',(1.,0.,0.));
#42480=DIRECTION('center_axis',(-1.,0.,0.));
#42481=DIRECTION('ref_axis',(0.,1.,0.));
#42482=DIRECTION('center_axis',(0.,0.,-1.));
#42483=DIRECTION('ref_axis',(-1.,0.,0.));
#42484=DIRECTION('center_axis',(0.,-6.12323399574E-17,-1.));
#42485=DIRECTION('ref_axis',(1.,0.,0.));
#42486=DIRECTION('',(0.,0.,-1.));
#42487=DIRECTION('center_axis',(0.,-1.,0.));
#42488=DIRECTION('ref_axis',(1.,0.,0.));
#42489=DIRECTION('center_axis',(-1.,0.,0.));
#42490=DIRECTION('ref_axis',(0.,1.,0.));
#42491=DIRECTION('center_axis',(0.,-1.,0.));
#42492=DIRECTION('ref_axis',(-1.,0.,0.));
#42493=DIRECTION('center_axis',(0.,-1.,0.));
#42494=DIRECTION('ref_axis',(0.,0.,-1.));
#42495=DIRECTION('',(0.,-1.,0.));
#42496=DIRECTION('center_axis',(1.,0.,0.));
#42497=DIRECTION('ref_axis',(0.,0.107526881719979,-0.994202177480807));
#42498=DIRECTION('center_axis',(0.,0.994202177480807,-0.107526881719979));
#42499=DIRECTION('ref_axis',(1.,0.,0.));
#42500=DIRECTION('center_axis',(-1.,0.,0.));
#42501=DIRECTION('ref_axis',(0.,1.,0.));
#42502=DIRECTION('center_axis',(0.,-0.994202177480807,-0.107526881719979));
#42503=DIRECTION('ref_axis',(1.,0.,0.));
#42504=DIRECTION('center_axis',(0.,0.433812003680988,0.901003410349976));
#42505=DIRECTION('ref_axis',(1.,0.,0.));
#42506=DIRECTION('',(0.,-0.901003410349976,0.433812003680988));
#42507=DIRECTION('',(-1.,0.,0.));
#42508=DIRECTION('',(1.,0.,0.));
#42509=DIRECTION('center_axis',(-0.0103217669355549,0.900955491125921,-0.433788732146629));
#42510=DIRECTION('ref_axis',(0.72659105028404,0.304799044389358,0.615762119804774));
#42511=DIRECTION('center_axis',(1.,0.,0.));
#42512=DIRECTION('ref_axis',(0.,-0.433812003680988,-0.901003410349976));
#42513=DIRECTION('',(1.,0.,0.));
#42514=DIRECTION('center_axis',(-1.,0.,0.));
#42515=DIRECTION('ref_axis',(0.,1.,0.));
#42516=DIRECTION('center_axis',(0.,0.,1.));
#42517=DIRECTION('ref_axis',(1.,0.,0.));
#42518=DIRECTION('',(0.,-1.,0.));
#42519=DIRECTION('',(-1.,0.,0.));
#42520=DIRECTION('center_axis',(1.,0.,0.));
#42521=DIRECTION('ref_axis',(0.,1.,0.));
#42522=DIRECTION('center_axis',(1.,0.,0.));
#42523=DIRECTION('ref_axis',(0.,1.,0.));
#42524=DIRECTION('',(-1.,0.,0.));
#42525=DIRECTION('center_axis',(0.,1.,0.));
#42526=DIRECTION('ref_axis',(1.,0.,0.));
#42527=DIRECTION('',(0.,0.,1.));
#42528=DIRECTION('',(-1.,0.,0.));
#42529=DIRECTION('center_axis',(1.,0.,0.));
#42530=DIRECTION('ref_axis',(0.,0.,-1.));
#42531=DIRECTION('center_axis',(1.,0.,0.));
#42532=DIRECTION('ref_axis',(0.,1.,0.));
#42533=DIRECTION('',(-1.,0.,0.));
#42534=DIRECTION('center_axis',(-0.0173651268263312,-0.999849214817067,
1.68859670582999E-8));
#42535=DIRECTION('ref_axis',(0.760990240424013,-0.0132166958731909,-0.648628686483722));
#42536=DIRECTION('center_axis',(0.,0.,1.));
#42537=DIRECTION('ref_axis',(1.,0.,0.));
#42538=DIRECTION('',(-1.,0.,0.));
#42539=DIRECTION('',(0.,-1.,0.));
#42540=DIRECTION('',(-1.,0.,0.));
#42541=DIRECTION('',(0.,1.,0.));
#42542=DIRECTION('center_axis',(0.0118198477658594,0.999930143159405,-6.38623129917418E-8));
#42543=DIRECTION('ref_axis',(0.727757019739868,-0.00860253433416321,0.685781099639218));
#42544=DIRECTION('center_axis',(0.0173638215992654,0.999849237484397,1.1573889087489E-6));
#42545=DIRECTION('ref_axis',(0.761020343050589,-0.0132169647677628,0.64859336205784));
#42546=DIRECTION('center_axis',(1.,0.,0.));
#42547=DIRECTION('ref_axis',(0.,-1.,0.));
#42548=DIRECTION('center_axis',(1.,0.,0.));
#42549=DIRECTION('ref_axis',(0.,-2.09002828430941E-15,-1.));
#42550=DIRECTION('center_axis',(-1.,0.,0.));
#42551=DIRECTION('ref_axis',(0.,1.,0.));
#42552=DIRECTION('',(1.,0.,0.));
#42553=DIRECTION('',(1.,0.,0.));
#42554=DIRECTION('center_axis',(1.,0.,0.));
#42555=DIRECTION('ref_axis',(0.,-1.,0.));
#42556=DIRECTION('center_axis',(-9.62964972193618E-33,-0.901003410349976,
0.433812003680988));
#42557=DIRECTION('ref_axis',(-6.43494414306736E-48,-0.433812003680988,-0.901003410349976));
#42558=DIRECTION('center_axis',(0.,-0.901003410349976,0.433812003680988));
#42559=DIRECTION('ref_axis',(1.,0.,0.));
#42560=DIRECTION('',(0.,-0.901003410349976,0.433812003680988));
#42561=DIRECTION('center_axis',(0.,-0.901003410349976,0.433812003680988));
#42562=DIRECTION('ref_axis',(1.,0.,0.));
#42563=DIRECTION('center_axis',(1.,0.,0.));
#42564=DIRECTION('ref_axis',(0.,0.433812003680988,0.901003410349976));
#42565=DIRECTION('center_axis',(1.,0.,0.));
#42566=DIRECTION('ref_axis',(0.,1.,0.));
#42567=DIRECTION('',(-1.,0.,0.));
#42568=DIRECTION('center_axis',(1.,0.,0.));
#42569=DIRECTION('ref_axis',(0.,-0.433812003680988,-0.901003410349975));
#42570=DIRECTION('center_axis',(0.,-1.,0.));
#42571=DIRECTION('ref_axis',(1.,0.,0.));
#42572=DIRECTION('center_axis',(-1.,0.,0.));
#42573=DIRECTION('ref_axis',(0.,1.,0.));
#42574=DIRECTION('center_axis',(0.,-1.,0.));
#42575=DIRECTION('ref_axis',(0.,0.,-1.));
#42576=DIRECTION('center_axis',(0.,-1.,-2.50640329593E-15));
#42577=DIRECTION('ref_axis',(1.,0.,0.));
#42578=DIRECTION('',(0.,-1.,0.));
#42579=DIRECTION('center_axis',(1.,0.,0.));
#42580=DIRECTION('ref_axis',(0.,1.,-1.26882631385732E-15));
#42581=DIRECTION('center_axis',(0.,0.,1.));
#42582=DIRECTION('ref_axis',(1.,0.,0.));
#42583=DIRECTION('center_axis',(1.,0.,0.));
#42584=DIRECTION('ref_axis',(0.,1.,0.));
#42585=DIRECTION('center_axis',(0.,0.,1.));
#42586=DIRECTION('ref_axis',(0.,-1.,0.));
#42587=DIRECTION('center_axis',(0.,6.53351286424E-16,1.));
#42588=DIRECTION('ref_axis',(1.,0.,0.));
#42589=DIRECTION('',(0.,0.,1.));
#42590=DIRECTION('center_axis',(1.,0.,0.));
#42591=DIRECTION('ref_axis',(0.,6.34413156928661E-16,-1.));
#42592=DIRECTION('center_axis',(0.,1.,0.));
#42593=DIRECTION('ref_axis',(1.,0.,0.));
#42594=DIRECTION('center_axis',(1.,0.,0.));
#42595=DIRECTION('ref_axis',(0.,1.,0.));
#42596=DIRECTION('center_axis',(-1.,1.38625597078213E-8,-8.47275514856299E-9));
#42597=DIRECTION('ref_axis',(8.4755411535573E-9,0.000200933695293934,-0.999999979812825));
#42598=DIRECTION('center_axis',(1.,0.,0.));
#42599=DIRECTION('ref_axis',(0.,0.,-1.));
#42600=DIRECTION('center_axis',(-1.,0.,0.));
#42601=DIRECTION('ref_axis',(0.,-1.,0.));
#42602=DIRECTION('',(-1.,0.,0.));
#42603=DIRECTION('center_axis',(0.,1.,0.));
#42604=DIRECTION('ref_axis',(0.,0.,-1.));
#42605=DIRECTION('',(0.,-1.,0.));
#42606=DIRECTION('center_axis',(0.,-1.,1.11022302463E-16));
#42607=DIRECTION('ref_axis',(1.,0.,0.));
#42608=DIRECTION('center_axis',(0.,-1.,-9.25185853854E-17));
#42609=DIRECTION('ref_axis',(1.,0.,0.));
#42610=DIRECTION('center_axis',(1.,0.,0.));
#42611=DIRECTION('ref_axis',(0.,-0.419820362992804,-0.907607218358575));
#42612=DIRECTION('center_axis',(1.,0.,0.));
#42613=DIRECTION('ref_axis',(0.,1.,0.));
#42614=DIRECTION('center_axis',(-1.,0.,0.));
#42615=DIRECTION('ref_axis',(0.,1.,0.));
#42616=DIRECTION('',(-1.,0.,0.));
#42617=DIRECTION('center_axis',(0.,-1.,0.));
#42618=DIRECTION('ref_axis',(1.,0.,0.));
#42619=DIRECTION('center_axis',(0.,1.,-5.55111512313E-17));
#42620=DIRECTION('ref_axis',(1.,0.,0.));
#42621=DIRECTION('',(0.,1.,0.));
#42622=DIRECTION('center_axis',(0.,0.,1.));
#42623=DIRECTION('ref_axis',(1.,0.,0.));
#42624=DIRECTION('',(0.,-1.,0.));
#42625=DIRECTION('',(-1.,0.,0.));
#42626=DIRECTION('',(0.,1.,0.));
#42627=DIRECTION('',(1.,0.,0.));
#42628=DIRECTION('center_axis',(1.,-1.76684878881754E-8,-1.39105393592899E-8));
#42629=DIRECTION('ref_axis',(1.39140895830399E-8,0.00020093320508201,0.999999979812923));
#42630=DIRECTION('center_axis',(-1.,0.,0.));
#42631=DIRECTION('ref_axis',(0.,-0.107526881719978,-0.994202177480807));
#42632=DIRECTION('',(1.,0.,0.));
#42633=DIRECTION('center_axis',(1.,0.,0.));
#42634=DIRECTION('ref_axis',(0.,1.,0.));
#42635=DIRECTION('center_axis',(1.,0.,0.));
#42636=DIRECTION('ref_axis',(0.,0.107526881719979,-0.994202177480807));
#42637=DIRECTION('center_axis',(-1.,0.,0.));
#42638=DIRECTION('ref_axis',(0.,1.,0.));
#42639=DIRECTION('center_axis',(0.,-0.994202177480807,-0.107526881719979));
#42640=DIRECTION('ref_axis',(1.,0.,0.));
#42641=DIRECTION('center_axis',(0.,0.994202177480807,-0.107526881719979));
#42642=DIRECTION('ref_axis',(1.,0.,0.));
#42643=DIRECTION('center_axis',(-1.,0.,0.));
#42644=DIRECTION('ref_axis',(0.,-1.,0.));
#42645=DIRECTION('center_axis',(1.,0.,0.));
#42646=DIRECTION('ref_axis',(0.,1.,0.));
#42647=DIRECTION('center_axis',(1.,0.,0.));
#42648=DIRECTION('ref_axis',(0.,0.433812003680988,0.901003410349976));
#42649=DIRECTION('center_axis',(1.,0.,0.));
#42650=DIRECTION('ref_axis',(0.,1.,0.));
#42651=DIRECTION('center_axis',(0.,-1.,0.));
#42652=DIRECTION('ref_axis',(1.,0.,0.));
#42653=DIRECTION('center_axis',(1.,0.,0.));
#42654=DIRECTION('ref_axis',(0.,1.,0.));
#42655=DIRECTION('',(0.,0.,-1.));
#42656=DIRECTION('center_axis',(1.,0.,0.));
#42657=DIRECTION('ref_axis',(0.,1.,0.));
#42658=DIRECTION('',(0.,-1.,0.));
#42659=DIRECTION('',(0.,0.,-1.));
#42660=DIRECTION('',(0.,1.,0.));
#42661=DIRECTION('center_axis',(1.,0.,0.));
#42662=DIRECTION('ref_axis',(0.,1.,0.));
#42663=DIRECTION('',(0.,0.,-1.));
#42664=DIRECTION('',(0.,1.,0.));
#42665=DIRECTION('',(0.,0.57980236498199,0.814757152506986));
#42666=DIRECTION('center_axis',(1.,0.,0.));
#42667=DIRECTION('ref_axis',(0.,1.,0.));
#42668=DIRECTION('',(0.,1.,0.));
#42669=DIRECTION('center_axis',(1.,0.,0.));
#42670=DIRECTION('ref_axis',(0.,1.,0.));
#42671=DIRECTION('',(0.,0.908754086213215,-0.417332015056099));
#42672=DIRECTION('center_axis',(-1.,0.,0.));
#42673=DIRECTION('ref_axis',(0.,1.,0.));
#42674=DIRECTION('',(0.,1.,0.));
#42675=DIRECTION('center_axis',(-1.,0.,0.));
#42676=DIRECTION('ref_axis',(0.,1.,0.));
#42677=DIRECTION('',(0.,0.726467397290375,0.687200931805355));
#42678=DIRECTION('center_axis',(-1.,0.,0.));
#42679=DIRECTION('ref_axis',(0.,1.,0.));
#42680=DIRECTION('center_axis',(1.,0.,0.));
#42681=DIRECTION('ref_axis',(0.,1.,0.));
#42682=DIRECTION('',(0.,-0.86428986298992,0.502994068287953));
#42683=DIRECTION('center_axis',(-1.,0.,0.));
#42684=DIRECTION('ref_axis',(0.,1.,0.));
#42685=DIRECTION('',(0.,-0.726467397290375,-0.687200931805355));
#42686=DIRECTION('center_axis',(1.,0.,0.));
#42687=DIRECTION('ref_axis',(0.,1.,0.));
#42688=DIRECTION('',(0.,-1.,0.));
#42689=DIRECTION('center_axis',(1.,0.,0.));
#42690=DIRECTION('ref_axis',(0.,1.,0.));
#42691=DIRECTION('',(0.,0.907607218358575,-0.419820362992804));
#42692=DIRECTION('center_axis',(-1.,0.,0.));
#42693=DIRECTION('ref_axis',(0.,1.,0.));
#42694=DIRECTION('',(0.,0.973671472169394,0.227955838450093));
#42695=DIRECTION('center_axis',(1.,0.,0.));
#42696=DIRECTION('ref_axis',(0.,1.,0.));
#42697=DIRECTION('center_axis',(-1.,0.,0.));
#42698=DIRECTION('ref_axis',(0.,1.,0.));
#42699=DIRECTION('',(0.,-0.907607218358575,0.419820362992804));
#42700=DIRECTION('center_axis',(-1.,0.,0.));
#42701=DIRECTION('ref_axis',(0.,1.,0.));
#42702=DIRECTION('',(0.,-1.,0.));
#42703=DIRECTION('center_axis',(0.,0.,1.));
#42704=DIRECTION('ref_axis',(1.,0.,0.));
#42705=DIRECTION('center_axis',(0.,-0.367447999014073,-0.930044067784185));
#42706=DIRECTION('ref_axis',(1.,0.,0.));
#42707=DIRECTION('center_axis',(1.,0.,0.));
#42708=DIRECTION('ref_axis',(0.,0.925572441975634,-0.37857054118785));
#42709=DIRECTION('center_axis',(-4.71844785466072E-16,-0.319261680225049,
-0.947666597248145));
#42710=DIRECTION('ref_axis',(1.,-4.12988579863361E-17,-4.83988402678584E-16));
#42711=DIRECTION('center_axis',(-1.,0.,0.));
#42712=DIRECTION('ref_axis',(0.,1.,0.));
#42713=DIRECTION('center_axis',(1.11022302463028E-15,0.0845895878810212,
-0.996415877845249));
#42714=DIRECTION('ref_axis',(1.,2.79313681155602E-17,1.11658771431272E-15));
#42715=DIRECTION('center_axis',(1.,0.,0.));
#42716=DIRECTION('ref_axis',(0.,1.,0.));
#42717=DIRECTION('center_axis',(1.,0.,0.));
#42718=DIRECTION('ref_axis',(0.,1.,0.));
#42719=DIRECTION('',(0.,-0.907607218358575,0.419820362992804));
#42720=DIRECTION('center_axis',(-1.,0.,0.));
#42721=DIRECTION('ref_axis',(0.,1.,0.));
#42722=DIRECTION('center_axis',(1.,0.,0.));
#42723=DIRECTION('ref_axis',(0.,1.,0.));
#42724=DIRECTION('center_axis',(1.,0.,0.));
#42725=DIRECTION('ref_axis',(0.,1.,0.));
#42726=DIRECTION('',(0.,1.,0.));
#42727=DIRECTION('center_axis',(-1.,0.,0.));
#42728=DIRECTION('ref_axis',(0.,1.,0.));
#42729=DIRECTION('',(0.,0.726467397290375,0.687200931805355));
#42730=DIRECTION('center_axis',(-1.,0.,0.));
#42731=DIRECTION('ref_axis',(0.,1.,0.));
#42732=DIRECTION('center_axis',(1.,0.,0.));
#42733=DIRECTION('ref_axis',(0.,-0.419820362992804,-0.907607218358575));
#42734=DIRECTION('center_axis',(0.,-0.907607218358575,0.419820362992804));
#42735=DIRECTION('ref_axis',(1.,0.,0.));
#42736=DIRECTION('center_axis',(0.,0.419820362992804,0.907607218358575));
#42737=DIRECTION('ref_axis',(1.,0.,0.));
#42738=DIRECTION('',(0.,-0.907607218358575,0.419820362992804));
#42739=DIRECTION('',(-1.,0.,0.));
#42740=DIRECTION('',(0.,0.907607218358575,-0.419820362992804));
#42741=DIRECTION('center_axis',(1.,0.,0.));
#42742=DIRECTION('ref_axis',(0.,-0.419820362992804,-0.907607218358575));
#42743=DIRECTION('center_axis',(0.,0.907607218358575,-0.419820362992804));
#42744=DIRECTION('ref_axis',(1.,0.,0.));
#42745=DIRECTION('center_axis',(0.,-1.,0.));
#42746=DIRECTION('ref_axis',(0.,0.,1.));
#42747=DIRECTION('center_axis',(0.,1.,6.36065274525E-16));
#42748=DIRECTION('ref_axis',(1.,0.,0.));
#42749=DIRECTION('center_axis',(0.,1.,1.7763568394E-15));
#42750=DIRECTION('ref_axis',(1.,0.,0.));
#42751=DIRECTION('center_axis',(1.,0.,0.));
#42752=DIRECTION('ref_axis',(0.,0.930044067784185,0.367447999014073));
#42753=DIRECTION('center_axis',(-1.,0.,0.));
#42754=DIRECTION('ref_axis',(0.,-1.,0.));
#42755=DIRECTION('center_axis',(1.,0.,0.));
#42756=DIRECTION('ref_axis',(0.,0.,1.));
#42757=DIRECTION('center_axis',(1.,0.,0.));
#42758=DIRECTION('ref_axis',(0.,1.,0.));
#42759=DIRECTION('',(-1.,0.,0.));
#42760=DIRECTION('center_axis',(-1.,0.,0.));
#42761=DIRECTION('ref_axis',(0.,1.,0.));
#42762=DIRECTION('center_axis',(0.,-1.,0.));
#42763=DIRECTION('ref_axis',(0.,0.,-1.));
#42764=DIRECTION('center_axis',(0.,-1.,-1.614869854E-15));
#42765=DIRECTION('ref_axis',(1.,0.,0.));
#42766=DIRECTION('center_axis',(1.,0.,0.));
#42767=DIRECTION('ref_axis',(0.,-0.930044067784185,-0.367447999014073));
#42768=DIRECTION('center_axis',(0.,0.367447999014073,-0.930044067784185));
#42769=DIRECTION('ref_axis',(1.,0.,0.));
#42770=DIRECTION('center_axis',(1.,0.,0.));
#42771=DIRECTION('ref_axis',(0.,-0.107526881719979,0.994202177480807));
#42772=DIRECTION('center_axis',(0.,-1.,0.));
#42773=DIRECTION('ref_axis',(0.,0.,-1.));
#42774=DIRECTION('center_axis',(0.,-1.,-3.99680288865E-15));
#42775=DIRECTION('ref_axis',(1.,0.,0.));
#42776=DIRECTION('',(0.,-1.,0.));
#42777=DIRECTION('center_axis',(0.,0.707106781186548,0.707106781186548));
#42778=DIRECTION('ref_axis',(0.,0.707106781186548,-0.707106781186548));
#42779=DIRECTION('center_axis',(1.,0.,0.));
#42780=DIRECTION('ref_axis',(0.,-0.419820362992805,-0.907607218358575));
#42781=DIRECTION('center_axis',(0.,-0.907607218358575,0.419820362992804));
#42782=DIRECTION('ref_axis',(1.,0.,0.));
#42783=DIRECTION('center_axis',(-1.,0.,0.));
#42784=DIRECTION('ref_axis',(0.,1.,0.));
#42785=DIRECTION('center_axis',(1.92592994438724E-32,-0.907607218358575,
0.419820362992804));
#42786=DIRECTION('ref_axis',(2.4880840830811E-46,-0.419820362992804,-0.907607218358575));
#42787=DIRECTION('center_axis',(0.,-0.907607218358575,0.419820362992804));
#42788=DIRECTION('ref_axis',(1.,0.,0.));
#42789=DIRECTION('',(0.,-0.907607218358575,0.419820362992804));
#42790=DIRECTION('center_axis',(1.,0.,0.));
#42791=DIRECTION('ref_axis',(0.,-0.72739643298632,0.686217479578288));
#42792=DIRECTION('center_axis',(0.,0.686217479578295,0.727396432986313));
#42793=DIRECTION('ref_axis',(1.,0.,0.));
#42794=DIRECTION('center_axis',(-1.,0.,0.));
#42795=DIRECTION('ref_axis',(0.,-1.,0.));
#42796=DIRECTION('center_axis',(1.,0.,0.));
#42797=DIRECTION('ref_axis',(0.,0.727396432986313,-0.686217479578295));
#42798=DIRECTION('center_axis',(0.,0.672677186066802,0.739936080580782));
#42799=DIRECTION('ref_axis',(1.,0.,0.));
#42800=DIRECTION('center_axis',(1.,0.,0.));
#42801=DIRECTION('ref_axis',(0.,1.,0.));
#42802=DIRECTION('center_axis',(0.,0.973671472169394,0.227955838450093));
#42803=DIRECTION('ref_axis',(0.,-0.227955838450093,0.973671472169394));
#42804=DIRECTION('center_axis',(0.,0.973671472169394,0.227955838450093));
#42805=DIRECTION('ref_axis',(1.,0.,0.));
#42806=DIRECTION('center_axis',(0.,0.973671472169394,0.227955838450093));
#42807=DIRECTION('ref_axis',(1.,0.,0.));
#42808=DIRECTION('',(0.,0.973671472169394,0.227955838450093));
#42809=DIRECTION('center_axis',(1.,0.,0.));
#42810=DIRECTION('ref_axis',(0.,0.419820362992802,0.907607218358576));
#42811=DIRECTION('center_axis',(0.,0.907607218358575,-0.419820362992804));
#42812=DIRECTION('ref_axis',(1.,0.,0.));
#42813=DIRECTION('center_axis',(-1.,0.,0.));
#42814=DIRECTION('ref_axis',(0.,-1.,0.));
#42815=DIRECTION('center_axis',(0.,-0.907607218358575,0.419820362992804));
#42816=DIRECTION('ref_axis',(1.,0.,0.));
#42817=DIRECTION('center_axis',(1.,0.,0.));
#42818=DIRECTION('ref_axis',(0.,0.,1.));
#42819=DIRECTION('center_axis',(0.,-0.726467397290375,-0.687200931805355));
#42820=DIRECTION('ref_axis',(1.,0.,0.));
#42821=DIRECTION('center_axis',(1.92592994438724E-32,-0.726467397290375,
-0.687200931805355));
#42822=DIRECTION('ref_axis',(-2.06468201548131E-46,0.687200931805355,-0.726467397290375));
#42823=DIRECTION('center_axis',(0.,-0.726467397290375,-0.687200931805355));
#42824=DIRECTION('ref_axis',(1.,0.,0.));
#42825=DIRECTION('',(0.,-0.726467397290375,-0.687200931805355));
#42826=DIRECTION('center_axis',(1.,0.,0.));
#42827=DIRECTION('ref_axis',(0.,-0.502994068287954,-0.864289862989919));
#42828=DIRECTION('center_axis',(0.,-0.86428986298992,0.502994068287953));
#42829=DIRECTION('ref_axis',(1.,0.,0.));
#42830=DIRECTION('center_axis',(-1.,0.,0.));
#42831=DIRECTION('ref_axis',(0.,-1.,0.));
#42832=DIRECTION('center_axis',(-9.62964972193618E-33,-0.86428986298992,
0.502994068287953));
#42833=DIRECTION('ref_axis',(-4.62384107026404E-47,-0.502994068287953,-0.86428986298992));
#42834=DIRECTION('center_axis',(0.,-0.86428986298992,0.502994068287953));
#42835=DIRECTION('ref_axis',(1.,0.,0.));
#42836=DIRECTION('',(0.,-0.86428986298992,0.502994068287953));
#42837=DIRECTION('center_axis',(1.,0.,0.));
#42838=DIRECTION('ref_axis',(0.,0.96323191500603,0.268671319485009));
#42839=DIRECTION('center_axis',(0.,-0.268671319485009,0.96323191500603));
#42840=DIRECTION('ref_axis',(1.,0.,0.));
#42841=DIRECTION('center_axis',(0.,-0.403636513060188,0.914919431056425));
#42842=DIRECTION('ref_axis',(1.,0.,0.));
#42843=DIRECTION('center_axis',(1.,0.,0.));
#42844=DIRECTION('ref_axis',(0.,1.,0.));
#42845=DIRECTION('center_axis',(1.,0.,0.));
#42846=DIRECTION('ref_axis',(0.,-0.687200931805354,0.726467397290377));
#42847=DIRECTION('center_axis',(0.,0.726467397290375,0.687200931805355));
#42848=DIRECTION('ref_axis',(1.,0.,0.));
#42849=DIRECTION('center_axis',(-1.,0.,0.));
#42850=DIRECTION('ref_axis',(0.,1.,0.));
#42851=DIRECTION('center_axis',(0.,-0.726467397290375,-0.687200931805355));
#42852=DIRECTION('ref_axis',(1.,0.,0.));
#42853=DIRECTION('center_axis',(0.,0.726467397290375,0.687200931805355));
#42854=DIRECTION('ref_axis',(1.,0.,0.));
#42855=DIRECTION('',(0.,0.726467397290375,0.687200931805355));
#42856=DIRECTION('center_axis',(1.,0.,0.));
#42857=DIRECTION('ref_axis',(0.,-3.5527136788005E-15,1.));
#42858=DIRECTION('center_axis',(0.,1.,0.));
#42859=DIRECTION('ref_axis',(1.,0.,0.));
#42860=DIRECTION('center_axis',(-1.,0.,0.));
#42861=DIRECTION('ref_axis',(0.,1.,0.));
#42862=DIRECTION('center_axis',(0.,-1.,0.));
#42863=DIRECTION('ref_axis',(1.,0.,0.));
#42864=DIRECTION('center_axis',(0.,1.,-4.99600361081E-16));
#42865=DIRECTION('ref_axis',(1.,0.,0.));
#42866=DIRECTION('',(0.,1.,0.));
#42867=DIRECTION('center_axis',(1.,0.,0.));
#42868=DIRECTION('ref_axis',(0.,0.417332015056099,0.908754086213215));
#42869=DIRECTION('center_axis',(0.,0.908754086213215,-0.417332015056099));
#42870=DIRECTION('ref_axis',(1.,0.,0.));
#42871=DIRECTION('center_axis',(-1.,0.,0.));
#42872=DIRECTION('ref_axis',(0.,1.,0.));
#42873=DIRECTION('center_axis',(0.,-0.908754086213215,0.417332015056099));
#42874=DIRECTION('ref_axis',(1.,0.,0.));
#42875=DIRECTION('center_axis',(0.,0.908754086213215,-0.417332015056099));
#42876=DIRECTION('ref_axis',(1.,0.,0.));
#42877=DIRECTION('',(0.,0.908754086213215,-0.417332015056099));
#42878=DIRECTION('center_axis',(1.,0.,0.));
#42879=DIRECTION('ref_axis',(0.,-0.417332015056099,-0.908754086213215));
#42880=DIRECTION('center_axis',(0.,1.,0.));
#42881=DIRECTION('ref_axis',(1.,0.,0.));
#42882=DIRECTION('center_axis',(1.,0.,0.));
#42883=DIRECTION('ref_axis',(0.,1.,0.));
#42884=DIRECTION('center_axis',(0.,-1.,0.));
#42885=DIRECTION('ref_axis',(1.,0.,0.));
#42886=DIRECTION('center_axis',(0.,1.,7.40148683083E-16));
#42887=DIRECTION('ref_axis',(1.,0.,0.));
#42888=DIRECTION('',(0.,1.,0.));
#42889=DIRECTION('center_axis',(1.,0.,0.));
#42890=DIRECTION('ref_axis',(0.,-2.53765262771464E-15,-1.));
#42891=DIRECTION('center_axis',(0.,0.57980236498199,0.814757152506986));
#42892=DIRECTION('ref_axis',(1.,0.,0.));
#42893=DIRECTION('center_axis',(1.,0.,0.));
#42894=DIRECTION('ref_axis',(0.,1.,0.));
#42895=DIRECTION('center_axis',(0.,-0.57980236498199,-0.814757152506986));
#42896=DIRECTION('ref_axis',(1.,0.,0.));
#42897=DIRECTION('center_axis',(0.,0.57980236498199,0.814757152506986));
#42898=DIRECTION('ref_axis',(1.,0.,0.));
#42899=DIRECTION('',(0.,0.57980236498199,0.814757152506986));
#42900=DIRECTION('center_axis',(0.,-1.,0.));
#42901=DIRECTION('ref_axis',(1.,0.,0.));
#42902=DIRECTION('center_axis',(0.,1.,-1.38777878078E-16));
#42903=DIRECTION('ref_axis',(1.,0.,0.));
#42904=DIRECTION('center_axis',(0.,1.,6.93889390391E-17));
#42905=DIRECTION('ref_axis',(1.,0.,0.));
#42906=DIRECTION('',(0.,1.,0.));
#42907=DIRECTION('center_axis',(0.,0.,1.));
#42908=DIRECTION('ref_axis',(1.,0.,0.));
#42909=DIRECTION('center_axis',(0.,3.46944695195E-17,-1.));
#42910=DIRECTION('ref_axis',(1.,0.,0.));
#42911=DIRECTION('center_axis',(0.,-4.4408920985E-15,-1.));
#42912=DIRECTION('ref_axis',(1.,0.,0.));
#42913=DIRECTION('',(0.,0.,-1.));
#42914=DIRECTION('center_axis',(1.,0.,0.));
#42915=DIRECTION('ref_axis',(0.,-1.,-3.5527136788005E-14));
#42916=DIRECTION('center_axis',(0.,1.,0.));
#42917=DIRECTION('ref_axis',(1.,0.,0.));
#42918=DIRECTION('center_axis',(1.,0.,0.));
#42919=DIRECTION('ref_axis',(0.,1.,0.));
#42920=DIRECTION('center_axis',(0.,-1.,0.));
#42921=DIRECTION('ref_axis',(1.,0.,0.));
#42922=DIRECTION('center_axis',(0.,1.,6.93889390391E-17));
#42923=DIRECTION('ref_axis',(1.,0.,0.));
#42924=DIRECTION('',(0.,1.,0.));
#42925=DIRECTION('center_axis',(0.,0.,1.));
#42926=DIRECTION('ref_axis',(1.,0.,0.));
#42927=DIRECTION('center_axis',(0.,3.46944695195E-17,-1.));
#42928=DIRECTION('ref_axis',(1.,0.,0.));
#42929=DIRECTION('center_axis',(0.,6.93889390391E-17,-1.));
#42930=DIRECTION('ref_axis',(1.,0.,0.));
#42931=DIRECTION('',(0.,0.,-1.));
#42932=DIRECTION('center_axis',(0.,-1.,0.));
#42933=DIRECTION('ref_axis',(0.,0.,-1.));
#42934=DIRECTION('center_axis',(0.,-1.,-3.46944695195E-17));
#42935=DIRECTION('ref_axis',(1.,0.,0.));
#42936=DIRECTION('center_axis',(0.,-1.,4.4408920985E-15));
#42937=DIRECTION('ref_axis',(1.,0.,0.));
#42938=DIRECTION('',(0.,-1.,0.));
#42939=DIRECTION('center_axis',(1.,0.,0.));
#42940=DIRECTION('ref_axis',(0.,7.10542735760101E-14,1.));
#42941=DIRECTION('center_axis',(0.,0.,-1.));
#42942=DIRECTION('ref_axis',(1.,0.,0.));
#42943=DIRECTION('center_axis',(1.,0.,0.));
#42944=DIRECTION('ref_axis',(0.,1.,0.));
#42945=DIRECTION('center_axis',(0.,0.,1.));
#42946=DIRECTION('ref_axis',(1.,0.,0.));
#42947=DIRECTION('',(0.,0.,-1.));
#42948=DIRECTION('center_axis',(1.,0.,0.));
#42949=DIRECTION('ref_axis',(0.,-1.,-2.39124959150034E-16));
#42950=DIRECTION('center_axis',(-1.,0.,0.));
#42951=DIRECTION('ref_axis',(0.,1.,0.));
#42952=DIRECTION('center_axis',(-1.,0.,0.));
#42953=DIRECTION('ref_axis',(0.,1.,0.));
#42954=DIRECTION('center_axis',(0.,3.62957527281301E-16,-1.));
#42955=DIRECTION('ref_axis',(0.,1.,3.62957527281301E-16));
#42956=DIRECTION('center_axis',(1.,0.,0.));
#42957=DIRECTION('ref_axis',(0.,0.,1.));
#42958=DIRECTION('center_axis',(0.,0.726467397290375,0.687200931805355));
#42959=DIRECTION('ref_axis',(1.,0.,0.));
#42960=DIRECTION('center_axis',(-1.,3.93147962979832E-15,5.94795371774818E-15));
#42961=DIRECTION('ref_axis',(6.92478089935691E-15,0.734190003119643,0.678944061995669));
#42962=DIRECTION('center_axis',(-5.73224391576859E-9,0.268671312840191,
-0.963231916859449));
#42963=DIRECTION('ref_axis',(-5.18104078158404E-14,0.963231916859449,0.268671312840191));
#42964=DIRECTION('center_axis',(-1.,0.,0.));
#42965=DIRECTION('ref_axis',(0.,1.,0.));
#42966=DIRECTION('center_axis',(2.73676276537777E-8,0.403636572488003,-0.914919404838556));
#42967=DIRECTION('ref_axis',(-6.96173815432251E-8,0.914919404838555,0.403636572487999));
#42968=DIRECTION('center_axis',(1.,0.,0.));
#42969=DIRECTION('ref_axis',(0.,-0.985518026541958,0.169570691337993));
#42970=DIRECTION('',(-1.,0.,0.));
#42971=DIRECTION('',(-1.,0.,0.));
#42972=DIRECTION('center_axis',(1.,-8.02179867202313E-15,-2.35887717715673E-15));
#42973=DIRECTION('ref_axis',(7.82801319057738E-15,0.997327347392217,-0.0730627274580159));
#42974=DIRECTION('center_axis',(5.57830379642003E-8,-0.403636428026677,
0.914919468570793));
#42975=DIRECTION('ref_axis',(-7.95659834314697E-14,0.914919468570794,0.403636428026678));
#42976=DIRECTION('center_axis',(1.,0.,0.));
#42977=DIRECTION('ref_axis',(0.,1.,0.));
#42978=DIRECTION('center_axis',(1.05822780461189E-7,-0.268671045025511,
0.963231991560127));
#42979=DIRECTION('ref_axis',(2.79567437663786E-7,0.963231991560103,0.268671045025474));
#42980=DIRECTION('center_axis',(1.,0.,0.));
#42981=DIRECTION('ref_axis',(0.,-0.985518026541958,0.169570691337993));
#42982=DIRECTION('',(-1.,0.,0.));
#42983=DIRECTION('center_axis',(1.,0.,0.));
#42984=DIRECTION('ref_axis',(0.,1.,0.));
#42985=DIRECTION('',(1.,0.,0.));
#42986=DIRECTION('center_axis',(-1.,-6.091226037548E-15,2.96434183740151E-15));
#42987=DIRECTION('ref_axis',(-6.77424218415349E-15,0.899174530813553,-0.437590177147782));
#42988=DIRECTION('center_axis',(-9.0860756207758E-13,-0.686217479581265,
-0.727396432983511));
#42989=DIRECTION('ref_axis',(5.73615229389664E-14,0.727396432983511,-0.686217479581266));
#42990=DIRECTION('center_axis',(-1.,0.,0.));
#42991=DIRECTION('ref_axis',(0.,1.,0.));
#42992=DIRECTION('center_axis',(1.,0.,0.));
#42993=DIRECTION('ref_axis',(0.,-0.985518026541958,0.169570691337993));
#42994=DIRECTION('',(-1.,0.,0.));
#42995=DIRECTION('',(-1.,0.,0.));
#42996=DIRECTION('center_axis',(1.,0.,0.));
#42997=DIRECTION('ref_axis',(0.,0.509059777782153,-0.860731167464259));
#42998=DIRECTION('center_axis',(1.,0.,0.));
#42999=DIRECTION('ref_axis',(0.,1.,0.));
#43000=DIRECTION('center_axis',(-1.19474117133794E-8,0.686217506760235,
0.727396407343181));
#43001=DIRECTION('ref_axis',(5.90198613961689E-8,0.727396407343179,-0.686217506760235));
#43002=DIRECTION('center_axis',(1.,0.,0.));
#43003=DIRECTION('ref_axis',(0.,-0.985518026541958,0.169570691337993));
#43004=DIRECTION('',(1.,0.,0.));
#43005=DIRECTION('center_axis',(1.,0.,0.));
#43006=DIRECTION('ref_axis',(0.,1.,0.));
#43007=DIRECTION('',(-1.,0.,0.));
#43008=DIRECTION('center_axis',(-0.72158910718404,0.350067294611212,0.597295613274472));
#43009=DIRECTION('ref_axis',(0.494822520302078,-0.342622923784054,0.798598901514125));
#43010=DIRECTION('center_axis',(0.,-0.726467397290375,-0.687200931805355));
#43011=DIRECTION('ref_axis',(1.,0.,0.));
#43012=DIRECTION('center_axis',(-0.816269637465565,0.41965920741329,0.396976105811274));
#43013=DIRECTION('ref_axis',(0.577671081976444,0.592993279016696,0.560941255470831));
#43014=DIRECTION('center_axis',(0.,-0.726467397290375,-0.687200931805355));
#43015=DIRECTION('ref_axis',(0.,-0.687200931805355,0.726467397290375));
#43016=DIRECTION('',(0.,0.726467397290375,0.687200931805355));
#43017=DIRECTION('center_axis',(-0.258644806000509,-0.1693466143229,-0.951012401888814));
#43018=DIRECTION('ref_axis',(-0.0704066837757783,-0.978589379636601,0.193405596977311));
#43019=DIRECTION('center_axis',(0.,-0.977144298741099,0.212577090576022));
#43020=DIRECTION('ref_axis',(1.,0.,0.));
#43021=DIRECTION('center_axis',(1.,0.,0.));
#43022=DIRECTION('ref_axis',(0.,0.419820362992805,0.907607218358575));
#43023=DIRECTION('center_axis',(1.,0.,0.));
#43024=DIRECTION('ref_axis',(0.,-1.,0.));
#43025=DIRECTION('center_axis',(0.,-0.907607218358575,0.419820362992804));
#43026=DIRECTION('ref_axis',(1.,0.,0.));
#43027=DIRECTION('center_axis',(5.29416742490447E-29,-0.907607218358575,
0.419820362992804));
#43028=DIRECTION('ref_axis',(-1.,-4.80502457004213E-29,2.22259929006807E-29));
#43029=DIRECTION('center_axis',(-1.,0.,0.));
#43030=DIRECTION('ref_axis',(0.,-0.227955838450089,0.973671472169395));
#43031=DIRECTION('',(-1.,0.,0.));
#43032=DIRECTION('center_axis',(0.,0.,1.));
#43033=DIRECTION('ref_axis',(1.,0.,0.));
#43034=DIRECTION('center_axis',(-1.97947233792048E-13,-0.68720093180552,
0.726467397290219));
#43035=DIRECTION('ref_axis',(0.657142409811958,0.547586747279966,0.517989003193967));
#43036=DIRECTION('center_axis',(0.,-0.687200931805355,0.726467397290375));
#43037=DIRECTION('ref_axis',(1.,0.,0.));
#43038=DIRECTION('center_axis',(-0.809300823598924,0.426722876366013,0.403657978625494));
#43039=DIRECTION('ref_axis',(1.04962473897651E-8,-0.687200924844299,0.726467403875177));
#43040=DIRECTION('center_axis',(0.,-0.687200931805355,0.726467397290375));
#43041=DIRECTION('ref_axis',(-1.,0.,0.));
#43042=DIRECTION('',(-1.,0.,0.));
#43043=DIRECTION('center_axis',(0.,0.,1.));
#43044=DIRECTION('ref_axis',(1.,0.,0.));
#43045=DIRECTION('',(-1.,0.,0.));
#43046=DIRECTION('',(0.,-1.,0.));
#43047=DIRECTION('',(-1.,0.,0.));
#43048=DIRECTION('center_axis',(1.,0.,0.));
#43049=DIRECTION('ref_axis',(0.,-0.419820362992804,-0.907607218358575));
#43050=DIRECTION('',(-1.,0.,0.));
#43051=DIRECTION('center_axis',(-1.,0.,0.));
#43052=DIRECTION('ref_axis',(0.,1.,0.));
#43053=DIRECTION('center_axis',(-1.07495723694558E-13,0.419820362992774,
0.907607218358589));
#43054=DIRECTION('ref_axis',(0.958193364102501,0.259685881990864,-0.120119605745937));
#43055=DIRECTION('center_axis',(-0.690862062643962,-0.656187848545089,0.303524492950896));
#43056=DIRECTION('ref_axis',(-1.09708538548473E-11,0.419820362981223,0.907607218363932));
#43057=DIRECTION('center_axis',(0.,0.419820362992804,0.907607218358575));
#43058=DIRECTION('ref_axis',(1.,0.,0.));
#43059=DIRECTION('center_axis',(-0.690862033103006,0.656187879687057,-0.303524492864391));
#43060=DIRECTION('ref_axis',(1.47203652509396E-7,0.419820474127234,0.907607166952511));
#43061=DIRECTION('center_axis',(0.,0.419820362992804,0.907607218358575));
#43062=DIRECTION('ref_axis',(1.,0.,0.));
#43063=DIRECTION('',(-1.,0.,0.));
#43064=DIRECTION('',(0.,-0.907607218358575,0.419820362992804));
#43065=DIRECTION('',(-1.,0.,0.));
#43066=DIRECTION('center_axis',(-1.,0.,0.));
#43067=DIRECTION('ref_axis',(0.,-0.419820362992802,-0.907607218358576));
#43068=DIRECTION('center_axis',(-1.,0.,0.));
#43069=DIRECTION('ref_axis',(0.,1.,0.));
#43070=DIRECTION('center_axis',(-1.,0.,0.));
#43071=DIRECTION('ref_axis',(0.,-0.419820362992802,-0.907607218358576));
#43072=DIRECTION('center_axis',(0.,-0.86993736790158,0.493162220702754));
#43073=DIRECTION('ref_axis',(0.,0.493162220702747,0.869937367901583));
#43074=DIRECTION('center_axis',(-1.,0.,0.));
#43075=DIRECTION('ref_axis',(0.,-1.,0.));
#43076=DIRECTION('center_axis',(0.,-0.227955838450092,0.973671472169394));
#43077=DIRECTION('ref_axis',(-1.,0.,0.));
#43078=DIRECTION('',(-1.,0.,0.));
#43079=DIRECTION('center_axis',(-1.,0.,0.));
#43080=DIRECTION('ref_axis',(0.,0.687200931805355,-0.726467397290376));
#43081=DIRECTION('',(-1.,0.,0.));
#43082=DIRECTION('center_axis',(0.,-0.502994068287953,-0.86428986298992));
#43083=DIRECTION('ref_axis',(0.,-0.86428986298992,0.502994068287953));
#43084=DIRECTION('',(-1.,0.,0.));
#43085=DIRECTION('center_axis',(0.,-0.379561655995102,-0.925166444105198));
#43086=DIRECTION('ref_axis',(0.,-0.925166444105201,0.379561655995094));
#43087=DIRECTION('center_axis',(-1.,0.,0.));
#43088=DIRECTION('ref_axis',(0.,-1.,0.));
#43089=DIRECTION('center_axis',(1.,0.,0.));
#43090=DIRECTION('ref_axis',(0.,-0.687200931805354,0.726467397290376));
#43091=DIRECTION('',(-1.,0.,0.));
#43092=DIRECTION('center_axis',(1.,0.,0.));
#43093=DIRECTION('ref_axis',(0.,-0.687200931805354,0.726467397290376));
#43094=DIRECTION('',(-1.,0.,0.));
#43095=DIRECTION('center_axis',(-1.,0.,0.));
#43096=DIRECTION('ref_axis',(0.,1.,0.));
#43097=DIRECTION('center_axis',(0.,-0.687200931805355,0.726467397290375));
#43098=DIRECTION('ref_axis',(-1.,0.,0.));
#43099=DIRECTION('',(-1.,0.,0.));
#43100=DIRECTION('',(0.,0.726467397290375,0.687200931805355));
#43101=DIRECTION('center_axis',(1.,0.,0.));
#43102=DIRECTION('ref_axis',(0.,0.,1.));
#43103=DIRECTION('',(-1.,0.,0.));
#43104=DIRECTION('center_axis',(-1.,0.,0.));
#43105=DIRECTION('ref_axis',(0.,1.,0.));
#43106=DIRECTION('center_axis',(0.,0.,1.));
#43107=DIRECTION('ref_axis',(1.,0.,0.));
#43108=DIRECTION('',(-1.,0.,0.));
#43109=DIRECTION('',(0.,1.,0.));
#43110=DIRECTION('center_axis',(1.,0.,0.));
#43111=DIRECTION('ref_axis',(0.,0.417332015056099,0.908754086213216));
#43112=DIRECTION('',(-1.,0.,0.));
#43113=DIRECTION('center_axis',(-1.,0.,0.));
#43114=DIRECTION('ref_axis',(0.,1.,0.));
#43115=DIRECTION('center_axis',(0.,0.417332015056099,0.908754086213215));
#43116=DIRECTION('ref_axis',(1.,0.,0.));
#43117=DIRECTION('',(1.,0.,0.));
#43118=DIRECTION('',(0.,0.908754086213215,-0.417332015056099));
#43119=DIRECTION('center_axis',(1.,0.,0.));
#43120=DIRECTION('ref_axis',(0.,-0.417332015056099,-0.908754086213215));
#43121=DIRECTION('',(1.,0.,0.));
#43122=DIRECTION('center_axis',(1.,0.,0.));
#43123=DIRECTION('ref_axis',(0.,1.,0.));
#43124=DIRECTION('center_axis',(0.,0.,1.));
#43125=DIRECTION('ref_axis',(1.,0.,0.));
#43126=DIRECTION('',(1.,0.,0.));
#43127=DIRECTION('',(0.,1.,0.));
#43128=DIRECTION('center_axis',(1.,0.,0.));
#43129=DIRECTION('ref_axis',(0.,0.,-1.));
#43130=DIRECTION('',(1.,0.,0.));
#43131=DIRECTION('center_axis',(1.,0.,0.));
#43132=DIRECTION('ref_axis',(0.,1.,0.));
#43133=DIRECTION('center_axis',(0.,-0.814757152506986,0.57980236498199));
#43134=DIRECTION('ref_axis',(-1.,0.,0.));
#43135=DIRECTION('',(-1.,0.,0.));
#43136=DIRECTION('',(0.,0.57980236498199,0.814757152506986));
#43137=DIRECTION('center_axis',(0.,0.,1.));
#43138=DIRECTION('ref_axis',(1.,0.,0.));
#43139=DIRECTION('center_axis',(-1.,0.,0.));
#43140=DIRECTION('ref_axis',(0.,1.,0.));
#43141=DIRECTION('center_axis',(0.,0.,1.));
#43142=DIRECTION('ref_axis',(1.,0.,0.));
#43143=DIRECTION('',(-1.,0.,0.));
#43144=DIRECTION('',(0.,1.,0.));
#43145=DIRECTION('',(-1.,0.,0.));
#43146=DIRECTION('center_axis',(0.,0.,1.));
#43147=DIRECTION('ref_axis',(1.,0.,0.));
#43148=DIRECTION('center_axis',(-1.,0.,0.));
#43149=DIRECTION('ref_axis',(0.,1.,0.));
#43150=DIRECTION('center_axis',(0.,1.,0.));
#43151=DIRECTION('ref_axis',(1.,0.,0.));
#43152=DIRECTION('',(1.,0.,0.));
#43153=DIRECTION('',(0.,0.,-1.));
#43154=DIRECTION('',(-1.,0.,0.));
#43155=DIRECTION('center_axis',(1.,0.,0.));
#43156=DIRECTION('ref_axis',(0.,-1.,0.));
#43157=DIRECTION('',(1.,0.,0.));
#43158=DIRECTION('center_axis',(1.,0.,0.));
#43159=DIRECTION('ref_axis',(0.,1.,0.));
#43160=DIRECTION('center_axis',(0.,0.,1.));
#43161=DIRECTION('ref_axis',(1.,0.,0.));
#43162=DIRECTION('',(-1.,0.,0.));
#43163=DIRECTION('',(0.,1.,0.));
#43164=DIRECTION('center_axis',(0.,0.,1.));
#43165=DIRECTION('ref_axis',(1.,0.,0.));
#43166=DIRECTION('center_axis',(-1.,0.,0.));
#43167=DIRECTION('ref_axis',(0.,1.,0.));
#43168=DIRECTION('center_axis',(0.,1.,0.));
#43169=DIRECTION('ref_axis',(1.,0.,0.));
#43170=DIRECTION('',(-1.,0.,0.));
#43171=DIRECTION('',(0.,0.,-1.));
#43172=DIRECTION('',(-1.,0.,0.));
#43173=DIRECTION('center_axis',(0.,0.,1.));
#43174=DIRECTION('ref_axis',(1.,0.,0.));
#43175=DIRECTION('center_axis',(-1.,0.,0.));
#43176=DIRECTION('ref_axis',(0.,1.,0.));
#43177=DIRECTION('center_axis',(0.,0.,1.));
#43178=DIRECTION('ref_axis',(1.,0.,0.));
#43179=DIRECTION('',(1.,0.,0.));
#43180=DIRECTION('',(0.,-1.,0.));
#43181=DIRECTION('',(-1.,0.,0.));
#43182=DIRECTION('center_axis',(1.,0.,0.));
#43183=DIRECTION('ref_axis',(0.,0.,1.));
#43184=DIRECTION('',(1.,0.,0.));
#43185=DIRECTION('center_axis',(1.,0.,0.));
#43186=DIRECTION('ref_axis',(0.,1.,0.));
#43187=DIRECTION('center_axis',(0.,1.,0.));
#43188=DIRECTION('ref_axis',(1.,0.,0.));
#43189=DIRECTION('',(0.,0.,-1.));
#43190=DIRECTION('center_axis',(1.,0.,0.));
#43191=DIRECTION('ref_axis',(0.,1.,0.));
#43192=DIRECTION('center_axis',(-1.,0.,0.));
#43193=DIRECTION('ref_axis',(0.,-1.,1.30922526488816E-16));
#43194=DIRECTION('',(-1.,0.,0.));
#43195=DIRECTION('center_axis',(-1.,0.,0.));
#43196=DIRECTION('ref_axis',(0.,0.96323191500603,0.268671319485009));
#43197=DIRECTION('center_axis',(0.,0.403636513060188,-0.914919431056425));
#43198=DIRECTION('ref_axis',(1.,0.,0.));
#43199=DIRECTION('center_axis',(1.,0.,0.));
#43200=DIRECTION('ref_axis',(0.,1.,0.));
#43201=DIRECTION('center_axis',(0.,0.268671319485009,-0.96323191500603));
#43202=DIRECTION('ref_axis',(1.,0.,0.));
#43203=DIRECTION('center_axis',(-1.,0.,0.));
#43204=DIRECTION('ref_axis',(0.,-0.502994068287962,-0.864289862989915));
#43205=DIRECTION('center_axis',(-1.,0.,0.));
#43206=DIRECTION('ref_axis',(0.,1.,0.));
#43207=DIRECTION('',(1.,0.,0.));
#43208=DIRECTION('center_axis',(1.,0.,0.));
#43209=DIRECTION('ref_axis',(0.,0.925572659293396,-0.378570009864162));
#43210=DIRECTION('center_axis',(2.08166817117052E-15,-0.0845895878810212,
0.996415877845249));
#43211=DIRECTION('ref_axis',(1.,-6.67956163323103E-18,-2.08972301509199E-15));
#43212=DIRECTION('center_axis',(1.,0.,0.));
#43213=DIRECTION('ref_axis',(0.,1.,0.));
#43214=DIRECTION('center_axis',(-6.10622663544094E-16,0.319261680225049,
0.947666597248145));
#43215=DIRECTION('ref_axis',(1.,-2.37377845073976E-17,6.52340422576772E-16));
#43216=DIRECTION('center_axis',(1.,0.,0.));
#43217=DIRECTION('ref_axis',(0.,1.,0.));
#43218=DIRECTION('',(0.,0.726467397290375,0.687200931805355));
#43219=DIRECTION('center_axis',(-1.,0.,0.));
#43220=DIRECTION('ref_axis',(0.,1.,0.));
#43221=DIRECTION('',(0.,1.,0.));
#43222=DIRECTION('center_axis',(1.,0.,0.));
#43223=DIRECTION('ref_axis',(0.,1.,0.));
#43224=DIRECTION('center_axis',(-1.,0.,0.));
#43225=DIRECTION('ref_axis',(0.,1.,0.));
#43226=DIRECTION('center_axis',(1.,0.,0.));
#43227=DIRECTION('ref_axis',(0.,1.,0.));
#43228=DIRECTION('',(0.,-1.,0.));
#43229=DIRECTION('center_axis',(-1.,0.,0.));
#43230=DIRECTION('ref_axis',(0.,1.,0.));
#43231=DIRECTION('',(0.,-0.907607218358575,0.419820362992804));
#43232=DIRECTION('center_axis',(1.,0.,0.));
#43233=DIRECTION('ref_axis',(0.,1.,0.));
#43234=DIRECTION('center_axis',(-1.,0.,0.));
#43235=DIRECTION('ref_axis',(0.,1.,0.));
#43236=DIRECTION('center_axis',(-1.,0.,0.));
#43237=DIRECTION('ref_axis',(0.,-0.739936080580779,0.672677186066805));
#43238=DIRECTION('',(1.,0.,0.));
#43239=DIRECTION('center_axis',(-1.,0.,0.));
#43240=DIRECTION('ref_axis',(0.,1.,0.));
#43241=DIRECTION('center_axis',(0.,0.,1.));
#43242=DIRECTION('ref_axis',(1.,0.,0.));
#43243=DIRECTION('center_axis',(0.,0.367447999014073,0.930044067784185));
#43244=DIRECTION('ref_axis',(1.,0.,0.));
#43245=DIRECTION('center_axis',(-1.,0.,0.));
#43246=DIRECTION('ref_axis',(0.,1.,0.));
#43247=DIRECTION('center_axis',(0.,1.,0.));
#43248=DIRECTION('ref_axis',(1.,0.,0.));
#43249=DIRECTION('center_axis',(-1.,0.,0.));
#43250=DIRECTION('ref_axis',(0.,-0.502994068287962,-0.864289862989915));
#43251=DIRECTION('center_axis',(-1.,0.,0.));
#43252=DIRECTION('ref_axis',(0.,-0.739936080580779,0.672677186066805));
#43253=DIRECTION('center_axis',(0.,1.,0.));
#43254=DIRECTION('ref_axis',(0.,0.,-1.));
#43255=DIRECTION('center_axis',(0.,-0.707106781186548,-0.707106781186548));
#43256=DIRECTION('ref_axis',(0.,0.707106781186548,-0.707106781186548));
#43257=DIRECTION('center_axis',(0.,1.,3.99680288865E-15));
#43258=DIRECTION('ref_axis',(1.,0.,0.));
#43259=DIRECTION('',(0.,-1.,0.));
#43260=DIRECTION('center_axis',(-1.,0.,0.));
#43261=DIRECTION('ref_axis',(0.,-0.419820362992805,-0.907607218358575));
#43262=DIRECTION('center_axis',(0.,0.907607218358575,-0.419820362992804));
#43263=DIRECTION('ref_axis',(1.,0.,0.));
#43264=DIRECTION('center_axis',(-1.,0.,0.));
#43265=DIRECTION('ref_axis',(0.,1.,0.));
#43266=DIRECTION('center_axis',(1.92592994438724E-32,0.907607218358575,
-0.419820362992804));
#43267=DIRECTION('ref_axis',(-2.4880840830811E-46,-0.419820362992804,-0.907607218358575));
#43268=DIRECTION('center_axis',(0.,0.907607218358575,-0.419820362992804));
#43269=DIRECTION('ref_axis',(1.,0.,0.));
#43270=DIRECTION('',(0.,-0.907607218358575,0.419820362992804));
#43271=DIRECTION('center_axis',(-1.,0.,0.));
#43272=DIRECTION('ref_axis',(0.,-0.72739643298632,0.686217479578288));
#43273=DIRECTION('center_axis',(0.,-0.686217479578295,-0.727396432986313));
#43274=DIRECTION('ref_axis',(1.,0.,0.));
#43275=DIRECTION('center_axis',(-1.,0.,0.));
#43276=DIRECTION('ref_axis',(0.,1.,0.));
#43277=DIRECTION('center_axis',(-1.,0.,0.));
#43278=DIRECTION('ref_axis',(0.,-0.687200931805354,0.726467397290377));
#43279=DIRECTION('center_axis',(0.,-0.726467397290375,-0.687200931805355));
#43280=DIRECTION('ref_axis',(1.,0.,0.));
#43281=DIRECTION('center_axis',(-1.,0.,0.));
#43282=DIRECTION('ref_axis',(0.,1.,0.));
#43283=DIRECTION('center_axis',(0.,0.726467397290375,0.687200931805355));
#43284=DIRECTION('ref_axis',(-1.,0.,0.));
#43285=DIRECTION('center_axis',(0.,-0.726467397290375,-0.687200931805355));
#43286=DIRECTION('ref_axis',(1.,0.,0.));
#43287=DIRECTION('',(0.,0.726467397290375,0.687200931805355));
#43288=DIRECTION('center_axis',(-1.,0.,0.));
#43289=DIRECTION('ref_axis',(0.,-3.5527136788005E-15,1.));
#43290=DIRECTION('center_axis',(0.,-1.,0.));
#43291=DIRECTION('ref_axis',(1.,0.,0.));
#43292=DIRECTION('center_axis',(-1.,0.,0.));
#43293=DIRECTION('ref_axis',(0.,1.,0.));
#43294=DIRECTION('center_axis',(0.,1.,0.));
#43295=DIRECTION('ref_axis',(-1.,0.,0.));
#43296=DIRECTION('center_axis',(0.,-1.,4.99600361081E-16));
#43297=DIRECTION('ref_axis',(1.,0.,0.));
#43298=DIRECTION('',(0.,1.,0.));
#43299=DIRECTION('center_axis',(-1.,0.,0.));
#43300=DIRECTION('ref_axis',(0.,0.417332015056099,0.908754086213215));
#43301=DIRECTION('center_axis',(0.,-0.908754086213215,0.417332015056099));
#43302=DIRECTION('ref_axis',(1.,0.,0.));
#43303=DIRECTION('center_axis',(-1.,0.,0.));
#43304=DIRECTION('ref_axis',(0.,1.,0.));
#43305=DIRECTION('center_axis',(0.,0.908754086213215,-0.417332015056099));
#43306=DIRECTION('ref_axis',(-1.,0.,0.));
#43307=DIRECTION('center_axis',(0.,-0.908754086213215,0.417332015056099));
#43308=DIRECTION('ref_axis',(1.,0.,0.));
#43309=DIRECTION('',(0.,0.908754086213215,-0.417332015056099));
#43310=DIRECTION('center_axis',(-1.,0.,0.));
#43311=DIRECTION('ref_axis',(0.,-0.417332015056099,-0.908754086213215));
#43312=DIRECTION('center_axis',(0.,-1.,0.));
#43313=DIRECTION('ref_axis',(1.,0.,0.));
#43314=DIRECTION('center_axis',(1.,0.,0.));
#43315=DIRECTION('ref_axis',(0.,1.,0.));
#43316=DIRECTION('center_axis',(0.,1.,0.));
#43317=DIRECTION('ref_axis',(-1.,0.,0.));
#43318=DIRECTION('center_axis',(0.,-1.,-7.40148683083E-16));
#43319=DIRECTION('ref_axis',(1.,0.,0.));
#43320=DIRECTION('',(0.,1.,0.));
#43321=DIRECTION('center_axis',(-1.,0.,0.));
#43322=DIRECTION('ref_axis',(0.,-2.53765262771464E-15,-1.));
#43323=DIRECTION('center_axis',(0.,-0.57980236498199,-0.814757152506986));
#43324=DIRECTION('ref_axis',(1.,0.,0.));
#43325=DIRECTION('center_axis',(1.,0.,0.));
#43326=DIRECTION('ref_axis',(0.,1.,0.));
#43327=DIRECTION('center_axis',(0.,0.57980236498199,0.814757152506986));
#43328=DIRECTION('ref_axis',(-1.,0.,0.));
#43329=DIRECTION('center_axis',(0.,-0.57980236498199,-0.814757152506986));
#43330=DIRECTION('ref_axis',(1.,0.,0.));
#43331=DIRECTION('',(0.,0.57980236498199,0.814757152506986));
#43332=DIRECTION('center_axis',(1.,0.,0.));
#43333=DIRECTION('ref_axis',(0.,0.,1.));
#43334=DIRECTION('center_axis',(-1.,0.,0.));
#43335=DIRECTION('ref_axis',(0.,1.,0.));
#43336=DIRECTION('center_axis',(0.,1.,0.));
#43337=DIRECTION('ref_axis',(-1.,0.,0.));
#43338=DIRECTION('center_axis',(0.,-1.,-6.93889390391E-17));
#43339=DIRECTION('ref_axis',(1.,0.,0.));
#43340=DIRECTION('',(0.,1.,0.));
#43341=DIRECTION('center_axis',(0.,-1.,1.38777878078E-16));
#43342=DIRECTION('ref_axis',(1.,0.,0.));
#43343=DIRECTION('center_axis',(1.,0.,0.));
#43344=DIRECTION('ref_axis',(0.,1.,0.));
#43345=DIRECTION('center_axis',(-1.,0.,0.));
#43346=DIRECTION('ref_axis',(0.,1.,0.));
#43347=DIRECTION('center_axis',(0.,0.,-1.));
#43348=DIRECTION('ref_axis',(-1.,0.,0.));
#43349=DIRECTION('center_axis',(0.,4.4408920985E-15,1.));
#43350=DIRECTION('ref_axis',(1.,0.,0.));
#43351=DIRECTION('',(0.,0.,-1.));
#43352=DIRECTION('center_axis',(0.,-3.46944695195E-17,1.));
#43353=DIRECTION('ref_axis',(1.,0.,0.));
#43354=DIRECTION('center_axis',(-1.,0.,0.));
#43355=DIRECTION('ref_axis',(0.,-1.,-3.5527136788005E-14));
#43356=DIRECTION('center_axis',(0.,-1.,0.));
#43357=DIRECTION('ref_axis',(1.,0.,0.));
#43358=DIRECTION('center_axis',(1.,0.,0.));
#43359=DIRECTION('ref_axis',(0.,1.,0.));
#43360=DIRECTION('center_axis',(0.,1.,0.));
#43361=DIRECTION('ref_axis',(-1.,0.,0.));
#43362=DIRECTION('center_axis',(0.,-1.,-6.93889390391E-17));
#43363=DIRECTION('ref_axis',(1.,0.,0.));
#43364=DIRECTION('',(0.,1.,0.));
#43365=DIRECTION('center_axis',(1.,0.,0.));
#43366=DIRECTION('ref_axis',(0.,1.,0.));
#43367=DIRECTION('center_axis',(-1.,0.,0.));
#43368=DIRECTION('ref_axis',(0.,1.,0.));
#43369=DIRECTION('center_axis',(0.,0.,-1.));
#43370=DIRECTION('ref_axis',(-1.,0.,0.));
#43371=DIRECTION('center_axis',(0.,-6.93889390391E-17,1.));
#43372=DIRECTION('ref_axis',(1.,0.,0.));
#43373=DIRECTION('',(0.,0.,-1.));
#43374=DIRECTION('center_axis',(0.,-3.46944695195E-17,1.));
#43375=DIRECTION('ref_axis',(1.,0.,0.));
#43376=DIRECTION('center_axis',(1.,0.,0.));
#43377=DIRECTION('ref_axis',(0.,0.,-1.));
#43378=DIRECTION('center_axis',(-1.,0.,0.));
#43379=DIRECTION('ref_axis',(0.,1.,0.));
#43380=DIRECTION('center_axis',(0.,1.,0.));
#43381=DIRECTION('ref_axis',(0.,0.,-1.));
#43382=DIRECTION('center_axis',(0.,1.,-4.4408920985E-15));
#43383=DIRECTION('ref_axis',(1.,0.,0.));
#43384=DIRECTION('',(0.,-1.,0.));
#43385=DIRECTION('center_axis',(0.,1.,3.46944695195E-17));
#43386=DIRECTION('ref_axis',(1.,0.,0.));
#43387=DIRECTION('center_axis',(-1.,0.,0.));
#43388=DIRECTION('ref_axis',(0.,7.10542735760101E-14,1.));
#43389=DIRECTION('center_axis',(0.,0.,1.));
#43390=DIRECTION('ref_axis',(1.,0.,0.));
#43391=DIRECTION('center_axis',(1.,0.,0.));
#43392=DIRECTION('ref_axis',(0.,1.,0.));
#43393=DIRECTION('center_axis',(0.,0.,-1.));
#43394=DIRECTION('ref_axis',(-1.,0.,0.));
#43395=DIRECTION('',(0.,0.,-1.));
#43396=DIRECTION('center_axis',(1.,0.,0.));
#43397=DIRECTION('ref_axis',(0.,1.,0.));
#43398=DIRECTION('center_axis',(1.,0.,0.));
#43399=DIRECTION('ref_axis',(0.,1.,0.));
#43400=DIRECTION('center_axis',(0.,-0.379561655995102,-0.925166444105198));
#43401=DIRECTION('ref_axis',(0.,-0.925166444105201,0.379561655995094));
#43402=DIRECTION('center_axis',(0.,0.86428986298992,-0.502994068287953));
#43403=DIRECTION('ref_axis',(1.,0.,0.));
#43404=DIRECTION('center_axis',(1.,1.76988078022002E-14,4.55191440096E-13));
#43405=DIRECTION('ref_axis',(-1.76988078022E-14,1.,-4.16314649483351E-16));
#43406=DIRECTION('center_axis',(-1.,0.,0.));
#43407=DIRECTION('ref_axis',(0.,-1.,0.));
#43408=DIRECTION('',(-0.788010753606638,0.615661475325766,-3.58876661851124E-13));
#43409=DIRECTION('center_axis',(-1.,2.05025983117E-16,1.75613383407E-16));
#43410=DIRECTION('ref_axis',(2.05025983117E-16,1.,2.62770395016422E-32));
#43411=DIRECTION('center_axis',(-1.,2.05025983117E-16,1.75613383407E-16));
#43412=DIRECTION('ref_axis',(2.05025983117E-16,1.,2.62770395016422E-32));
#43413=DIRECTION('center_axis',(0.,0.502994068287953,0.86428986298992));
#43414=DIRECTION('ref_axis',(1.,0.,0.));
#43415=DIRECTION('',(0.,-0.86428986298992,0.502994068287953));
#43416=DIRECTION('',(1.,0.,0.));
#43417=DIRECTION('center_axis',(-1.,0.,0.));
#43418=DIRECTION('ref_axis',(0.,1.,0.));
#43419=DIRECTION('center_axis',(-1.,0.,0.));
#43420=DIRECTION('ref_axis',(0.,1.,0.));
#43421=DIRECTION('center_axis',(0.,-1.28102656687518E-16,-1.));
#43422=DIRECTION('ref_axis',(0.,-1.,1.28102656687518E-16));
#43423=DIRECTION('center_axis',(0.,1.,0.));
#43424=DIRECTION('ref_axis',(0.,0.,1.));
#43425=DIRECTION('center_axis',(0.,-1.,-1.7763568394E-15));
#43426=DIRECTION('ref_axis',(1.,0.,0.));
#43427=DIRECTION('',(0.,1.,0.));
#43428=DIRECTION('center_axis',(0.,-1.,-6.36065274525E-16));
#43429=DIRECTION('ref_axis',(1.,0.,0.));
#43430=DIRECTION('center_axis',(-1.,0.,0.));
#43431=DIRECTION('ref_axis',(0.,0.,1.));
#43432=DIRECTION('center_axis',(0.,-0.726467397290375,-0.687200931805355));
#43433=DIRECTION('ref_axis',(1.,0.,0.));
#43434=DIRECTION('center_axis',(-1.,0.,0.));
#43435=DIRECTION('ref_axis',(0.,1.,0.));
#43436=DIRECTION('center_axis',(-1.,0.,0.));
#43437=DIRECTION('ref_axis',(0.,-0.419820362992804,-0.907607218358575));
#43438=DIRECTION('center_axis',(0.,1.,0.));
#43439=DIRECTION('ref_axis',(1.,0.,0.));
#43440=DIRECTION('center_axis',(-1.,0.,0.));
#43441=DIRECTION('ref_axis',(0.,1.,0.));
#43442=DIRECTION('center_axis',(0.,0.907607218358575,-0.419820362992804));
#43443=DIRECTION('ref_axis',(1.,0.,0.));
#43444=DIRECTION('center_axis',(0.,-1.,0.));
#43445=DIRECTION('ref_axis',(0.,0.,-1.));
#43446=DIRECTION('',(0.,-1.,0.));
#43447=DIRECTION('center_axis',(-1.,0.,0.));
#43448=DIRECTION('ref_axis',(0.,-0.107526881719979,0.994202177480807));
#43449=DIRECTION('center_axis',(0.,0.994202177480807,0.107526881719979));
#43450=DIRECTION('ref_axis',(1.,0.,0.));
#43451=DIRECTION('center_axis',(1.,0.,0.));
#43452=DIRECTION('ref_axis',(0.,-1.,0.));
#43453=DIRECTION('center_axis',(0.187357668294215,0.0206872986033109,0.982073897325376));
#43454=DIRECTION('ref_axis',(0.854656229332195,0.48939719485811,-0.17335834369504));
#43455=DIRECTION('center_axis',(-0.816269637465565,-0.41965920741329,-0.396976105811274));
#43456=DIRECTION('ref_axis',(0.577671081976444,-0.592993279016696,-0.560941255470831));
#43457=DIRECTION('center_axis',(0.,-0.726467397290375,-0.687200931805355));
#43458=DIRECTION('ref_axis',(1.,0.,0.));
#43459=DIRECTION('center_axis',(0.,0.726467397290375,0.687200931805355));
#43460=DIRECTION('ref_axis',(0.,-0.687200931805355,0.726467397290375));
#43461=DIRECTION('',(0.,0.726467397290375,0.687200931805355));
#43462=DIRECTION('center_axis',(0.860803892811723,0.39426976223081,-0.321819845116245));
#43463=DIRECTION('ref_axis',(-0.15670617194301,-0.396284218850021,-0.904655732069054));
#43464=DIRECTION('center_axis',(0.,-0.977144298741099,0.212577090576022));
#43465=DIRECTION('ref_axis',(1.,0.,0.));
#43466=DIRECTION('center_axis',(-1.,0.,0.));
#43467=DIRECTION('ref_axis',(0.,0.419820362992805,0.907607218358575));
#43468=DIRECTION('center_axis',(0.,0.907607218358575,-0.419820362992804));
#43469=DIRECTION('ref_axis',(1.,0.,0.));
#43470=DIRECTION('center_axis',(1.,0.,0.));
#43471=DIRECTION('ref_axis',(0.,-1.,0.));
#43472=DIRECTION('center_axis',(5.29416742490447E-29,0.907607218358575,
-0.419820362992804));
#43473=DIRECTION('ref_axis',(1.,-4.80502457004213E-29,2.22259929006807E-29));
#43474=DIRECTION('',(0.,-0.907607218358575,0.419820362992804));
#43475=DIRECTION('center_axis',(-1.,0.,0.));
#43476=DIRECTION('ref_axis',(0.,-0.930044067784185,-0.367447999014073));
#43477=DIRECTION('center_axis',(0.,-0.367447999014073,0.930044067784185));
#43478=DIRECTION('ref_axis',(1.,0.,0.));
#43479=DIRECTION('center_axis',(1.,0.,0.));
#43480=DIRECTION('ref_axis',(0.,-1.,0.));
#43481=DIRECTION('center_axis',(0.,-0.994202177480807,0.107526881719979));
#43482=DIRECTION('ref_axis',(1.,0.,0.));
#43483=DIRECTION('center_axis',(-1.,0.,0.));
#43484=DIRECTION('ref_axis',(0.,0.107526881719979,-0.994202177480807));
#43485=DIRECTION('center_axis',(-1.,0.,0.));
#43486=DIRECTION('ref_axis',(0.,1.,0.));
#43487=DIRECTION('center_axis',(0.,0.227955838450092,-0.973671472169394));
#43488=DIRECTION('ref_axis',(-1.,0.,0.));
#43489=DIRECTION('',(1.,0.,0.));
#43490=DIRECTION('',(0.,0.973671472169394,0.227955838450093));
#43491=DIRECTION('center_axis',(1.,-3.93687335395956E-16,-1.5579751070446E-16));
#43492=DIRECTION('ref_axis',(-3.60046877990609E-16,-0.994529145503541,0.104459459810952));
#43493=DIRECTION('center_axis',(1.9606953158236E-16,0.104459459810952,0.994529145503541));
#43494=DIRECTION('ref_axis',(4.50058597488261E-16,0.994529145503542,-0.104459459810952));
#43495=DIRECTION('center_axis',(-1.,4.69073756832726E-16,-2.82798301772873E-22));
#43496=DIRECTION('ref_axis',(-4.69073756826505E-16,-0.999999999999273,1.20579937603916E-6));
#43497=DIRECTION('center_axis',(-1.,-4.69075046723531E-16,4.6907432243473E-16));
#43498=DIRECTION('ref_axis',(-4.69073756826505E-16,0.999999999977518,6.70552506222274E-6));
#43499=DIRECTION('center_axis',(-1.,4.69073756832726E-16,-2.82798301772873E-22));
#43500=DIRECTION('ref_axis',(-4.69073756826505E-16,-0.999999999999273,1.20579937603916E-6));
#43501=DIRECTION('center_axis',(0.,0.,1.));
#43502=DIRECTION('ref_axis',(1.,0.,0.));
#43503=DIRECTION('center_axis',(0.,0.,1.));
#43504=DIRECTION('ref_axis',(1.,0.,0.));
#43505=DIRECTION('center_axis',(0.,0.,1.));
#43506=DIRECTION('ref_axis',(1.,0.,0.));
#43507=DIRECTION('center_axis',(0.,0.,1.));
#43508=DIRECTION('ref_axis',(1.,0.,0.));
#43509=DIRECTION('center_axis',(1.,0.,0.));
#43510=DIRECTION('ref_axis',(0.,1.,-1.1229236786457E-15));
#43511=DIRECTION('center_axis',(-1.,0.,0.));
#43512=DIRECTION('ref_axis',(0.,1.,3.46944695195361E-16));
#43513=DIRECTION('',(1.,0.,0.));
#43514=DIRECTION('center_axis',(-9.62964972193618E-33,0.86428986298992,
-0.502994068287953));
#43515=DIRECTION('ref_axis',(4.62384107026404E-47,-0.502994068287953,-0.86428986298992));
#43516=DIRECTION('',(0.,-0.86428986298992,0.502994068287953));
#43517=DIRECTION('center_axis',(0.,0.86428986298992,-0.502994068287953));
#43518=DIRECTION('ref_axis',(1.,0.,0.));
#43519=DIRECTION('center_axis',(-1.,0.,0.));
#43520=DIRECTION('ref_axis',(0.,-0.502994068287954,-0.864289862989919));
#43521=DIRECTION('center_axis',(-1.,0.,0.));
#43522=DIRECTION('ref_axis',(0.,-1.,0.));
#43523=DIRECTION('center_axis',(-1.,0.,0.));
#43524=DIRECTION('ref_axis',(0.,1.,0.));
#43525=DIRECTION('center_axis',(0.,0.726467397290375,0.687200931805355));
#43526=DIRECTION('ref_axis',(1.,0.,0.));
#43527=DIRECTION('center_axis',(1.92592994438724E-32,0.726467397290375,
0.687200931805355));
#43528=DIRECTION('ref_axis',(2.06468201548131E-46,0.687200931805355,-0.726467397290375));
#43529=DIRECTION('',(0.,-0.726467397290375,-0.687200931805355));
#43530=DIRECTION('',(0.,-0.726467397290375,-0.687200931805355));
#43531=DIRECTION('center_axis',(0.,0.726467397290375,0.687200931805355));
#43532=DIRECTION('ref_axis',(1.,0.,0.));
#43533=DIRECTION('center_axis',(-1.,0.,0.));
#43534=DIRECTION('ref_axis',(0.,0.,1.));
#43535=DIRECTION('center_axis',(1.,0.,0.));
#43536=DIRECTION('ref_axis',(0.,1.,0.));
#43537=DIRECTION('center_axis',(1.,0.,0.));
#43538=DIRECTION('ref_axis',(0.,1.,0.));
#43539=DIRECTION('center_axis',(0.,1.,0.));
#43540=DIRECTION('ref_axis',(1.,0.,0.));
#43541=DIRECTION('center_axis',(0.,1.,0.));
#43542=DIRECTION('ref_axis',(0.,0.,-1.));
#43543=DIRECTION('',(0.,-1.,0.));
#43544=DIRECTION('',(0.,-1.,0.));
#43545=DIRECTION('center_axis',(0.,1.,-4.82947015712E-15));
#43546=DIRECTION('ref_axis',(1.,0.,0.));
#43547=DIRECTION('center_axis',(0.,0.,1.));
#43548=DIRECTION('ref_axis',(1.,0.,0.));
#43549=DIRECTION('center_axis',(-1.,0.,0.));
#43550=DIRECTION('ref_axis',(0.,1.,0.));
#43551=DIRECTION('center_axis',(1.,0.,0.));
#43552=DIRECTION('ref_axis',(0.,0.,1.));
#43553=DIRECTION('',(1.,0.,0.));
#43554=DIRECTION('',(1.,0.,0.));
#43555=DIRECTION('center_axis',(1.53432918126103E-13,-0.687200931805562,
0.72646739729018));
#43556=DIRECTION('ref_axis',(-0.474694932580992,0.63940056798499,0.60484017280799));
#43557=DIRECTION('center_axis',(-0.809300828659765,-0.426722873335083,-0.403657971683043));
#43558=DIRECTION('ref_axis',(4.78167372553401E-5,-0.687248789804423,0.726422121514699));
#43559=DIRECTION('center_axis',(0.,-0.687200931805355,0.726467397290375));
#43560=DIRECTION('ref_axis',(1.,0.,0.));
#43561=DIRECTION('center_axis',(0.,-0.687200931805355,0.726467397290375));
#43562=DIRECTION('ref_axis',(-1.,0.,0.));
#43563=DIRECTION('',(1.,0.,0.));
#43564=DIRECTION('center_axis',(-1.,0.,0.));
#43565=DIRECTION('ref_axis',(0.,1.,0.));
#43566=DIRECTION('center_axis',(0.,1.30922526488816E-16,1.));
#43567=DIRECTION('ref_axis',(0.,-1.,1.30922526488816E-16));
#43568=DIRECTION('center_axis',(-1.,0.,0.));
#43569=DIRECTION('ref_axis',(0.,1.,0.));
#43570=DIRECTION('center_axis',(1.,0.,0.));
#43571=DIRECTION('ref_axis',(0.,1.,0.));
#43572=DIRECTION('center_axis',(-1.,0.,0.));
#43573=DIRECTION('ref_axis',(0.,-0.433812003680988,-0.901003410349975));
#43574=DIRECTION('center_axis',(0.,-0.901003410349976,0.433812003680988));
#43575=DIRECTION('ref_axis',(1.,0.,0.));
#43576=DIRECTION('center_axis',(1.,0.,0.));
#43577=DIRECTION('ref_axis',(0.,1.,0.));
#43578=DIRECTION('center_axis',(0.,-1.,0.));
#43579=DIRECTION('ref_axis',(1.,0.,0.));
#43580=DIRECTION('center_axis',(1.,0.,0.));
#43581=DIRECTION('ref_axis',(0.,1.,0.));
#43582=DIRECTION('center_axis',(1.,0.,0.));
#43583=DIRECTION('ref_axis',(0.,0.,-1.));
#43584=DIRECTION('',(1.,0.,0.));
#43585=DIRECTION('center_axis',(-1.,-5.53814966532964E-9,-3.76666845086606E-9));
#43586=DIRECTION('ref_axis',(3.76666845861945E-9,-1.40000233628258E-9,-1.));
#43587=DIRECTION('',(1.,0.,0.));
#43588=DIRECTION('center_axis',(0.,-1.,0.));
#43589=DIRECTION('ref_axis',(1.,0.,0.));
#43590=DIRECTION('center_axis',(-1.,0.,0.));
#43591=DIRECTION('ref_axis',(0.,1.,0.));
#43592=DIRECTION('center_axis',(0.,0.,1.));
#43593=DIRECTION('ref_axis',(1.,0.,0.));
#43594=DIRECTION('center_axis',(-1.,0.,0.));
#43595=DIRECTION('ref_axis',(0.,1.,0.));
#43596=DIRECTION('center_axis',(0.,-1.,0.));
#43597=DIRECTION('ref_axis',(1.,0.,0.));
#43598=DIRECTION('',(0.,1.,0.));
#43599=DIRECTION('',(0.,1.,0.));
#43600=DIRECTION('center_axis',(-1.,0.,0.));
#43601=DIRECTION('ref_axis',(0.,0.687200931805355,-0.726467397290376));
#43602=DIRECTION('center_axis',(1.,0.,0.));
#43603=DIRECTION('ref_axis',(0.,1.,0.));
#43604=DIRECTION('',(-1.,0.,0.));
#43605=DIRECTION('center_axis',(0.,0.,1.));
#43606=DIRECTION('ref_axis',(1.,0.,0.));
#43607=DIRECTION('',(0.,0.,-1.));
#43608=DIRECTION('center_axis',(0.,6.12323399574E-17,1.));
#43609=DIRECTION('ref_axis',(1.,0.,0.));
#43610=DIRECTION('',(0.,0.,-1.));
#43611=DIRECTION('center_axis',(-1.,0.,0.));
#43612=DIRECTION('ref_axis',(0.,-0.419820362992804,-0.907607218358575));
#43613=DIRECTION('center_axis',(1.,0.,0.));
#43614=DIRECTION('ref_axis',(0.,1.,0.));
#43615=DIRECTION('center_axis',(0.,-1.,0.));
#43616=DIRECTION('ref_axis',(1.,0.,0.));
#43617=DIRECTION('center_axis',(1.,0.,0.));
#43618=DIRECTION('ref_axis',(0.,1.,0.));
#43619=DIRECTION('center_axis',(0.,-0.907607218358575,0.419820362992804));
#43620=DIRECTION('ref_axis',(1.,0.,0.));
#43621=DIRECTION('center_axis',(0.,0.907607218358575,-0.419820362992804));
#43622=DIRECTION('ref_axis',(-1.,0.,0.));
#43623=DIRECTION('',(0.,0.907607218358575,-0.419820362992804));
#43624=DIRECTION('',(0.,0.907607218358575,-0.419820362992804));
#43625=DIRECTION('center_axis',(0.,-0.907607218358575,0.419820362992804));
#43626=DIRECTION('ref_axis',(1.,0.,0.));
#43627=DIRECTION('center_axis',(1.,0.,0.));
#43628=DIRECTION('ref_axis',(0.,1.,0.));
#43629=DIRECTION('center_axis',(1.,0.,0.));
#43630=DIRECTION('ref_axis',(0.,1.,0.));
#43631=DIRECTION('',(0.,0.973671472169394,0.227955838450093));
#43632=DIRECTION('center_axis',(-1.,0.,0.));
#43633=DIRECTION('ref_axis',(0.,1.,0.));
#43634=DIRECTION('',(0.,1.,0.));
#43635=DIRECTION('center_axis',(1.,0.,0.));
#43636=DIRECTION('ref_axis',(0.,1.,0.));
#43637=DIRECTION('',(0.,0.,1.));
#43638=DIRECTION('center_axis',(1.,0.,0.));
#43639=DIRECTION('ref_axis',(0.,1.,0.));
#43640=DIRECTION('',(0.,-1.,0.));
#43641=DIRECTION('center_axis',(-1.,0.,0.));
#43642=DIRECTION('ref_axis',(0.,1.,0.));
#43643=DIRECTION('',(0.,-0.901003410349976,0.433812003680988));
#43644=DIRECTION('center_axis',(1.,0.,0.));
#43645=DIRECTION('ref_axis',(0.,1.,0.));
#43646=DIRECTION('center_axis',(-1.,0.,0.));
#43647=DIRECTION('ref_axis',(0.,0.727396432986313,-0.686217479578295));
#43648=DIRECTION('center_axis',(0.,-0.672677186066802,-0.739936080580782));
#43649=DIRECTION('ref_axis',(1.,0.,0.));
#43650=DIRECTION('center_axis',(0.,-0.86993736790158,0.493162220702754));
#43651=DIRECTION('ref_axis',(0.,0.493162220702747,0.869937367901583));
#43652=DIRECTION('center_axis',(0.,-0.973671472169394,-0.227955838450093));
#43653=DIRECTION('ref_axis',(1.,0.,0.));
#43654=DIRECTION('center_axis',(0.,-0.973671472169394,-0.227955838450093));
#43655=DIRECTION('ref_axis',(0.,-0.227955838450093,0.973671472169394));
#43656=DIRECTION('center_axis',(0.,-0.973671472169394,-0.227955838450093));
#43657=DIRECTION('ref_axis',(1.,0.,0.));
#43658=DIRECTION('center_axis',(-1.,0.,0.));
#43659=DIRECTION('ref_axis',(0.,0.419820362992802,0.907607218358576));
#43660=DIRECTION('center_axis',(-1.,0.,0.));
#43661=DIRECTION('ref_axis',(0.,-1.,0.));
#43662=DIRECTION('center_axis',(-1.,0.,0.));
#43663=DIRECTION('ref_axis',(0.,-0.227955838450089,0.973671472169395));
#43664=DIRECTION('',(1.,0.,0.));
#43665=DIRECTION('center_axis',(0.,0.419820362992804,0.907607218358575));
#43666=DIRECTION('ref_axis',(1.,0.,0.));
#43667=DIRECTION('',(1.,0.,0.));
#43668=DIRECTION('center_axis',(1.,0.,0.));
#43669=DIRECTION('ref_axis',(0.,-0.419820362992804,-0.907607218358575));
#43670=DIRECTION('',(1.,0.,0.));
#43671=DIRECTION('center_axis',(0.,0.,1.));
#43672=DIRECTION('ref_axis',(1.,0.,0.));
#43673=DIRECTION('',(0.,1.,0.));
#43674=DIRECTION('',(0.,-1.,0.));
#43675=DIRECTION('',(1.,0.,0.));
#43676=DIRECTION('center_axis',(0.,1.,0.));
#43677=DIRECTION('ref_axis',(-1.,0.,0.));
#43678=DIRECTION('center_axis',(0.,-1.,-1.48029736617E-15));
#43679=DIRECTION('ref_axis',(1.,0.,0.));
#43680=DIRECTION('center_axis',(-1.,0.,0.));
#43681=DIRECTION('ref_axis',(0.,6.34413156928661E-16,-1.));
#43682=DIRECTION('center_axis',(1.,0.,0.));
#43683=DIRECTION('ref_axis',(0.,1.,0.));
#43684=DIRECTION('center_axis',(0.,0.,-1.));
#43685=DIRECTION('ref_axis',(1.,0.,0.));
#43686=DIRECTION('center_axis',(0.,0.,-1.));
#43687=DIRECTION('ref_axis',(0.,-1.,0.));
#43688=DIRECTION('',(0.,0.,1.));
#43689=DIRECTION('center_axis',(0.,1.67945721619E-15,-1.));
#43690=DIRECTION('ref_axis',(1.,0.,0.));
#43691=DIRECTION('center_axis',(-1.,0.,0.));
#43692=DIRECTION('ref_axis',(0.,1.,-1.26882631385732E-15));
#43693=DIRECTION('center_axis',(1.,0.,0.));
#43694=DIRECTION('ref_axis',(0.,1.,0.));
#43695=DIRECTION('center_axis',(0.,1.,0.));
#43696=DIRECTION('ref_axis',(1.,0.,0.));
#43697=DIRECTION('center_axis',(0.,1.,0.));
#43698=DIRECTION('ref_axis',(0.,0.,-1.));
#43699=DIRECTION('',(0.,-1.,0.));
#43700=DIRECTION('center_axis',(0.,1.,-4.99600361081E-16));
#43701=DIRECTION('ref_axis',(1.,0.,0.));
#43702=DIRECTION('center_axis',(-1.,0.,0.));
#43703=DIRECTION('ref_axis',(0.,-0.433812003680988,-0.901003410349975));
#43704=DIRECTION('center_axis',(-1.,0.,0.));
#43705=DIRECTION('ref_axis',(0.,1.,0.));
#43706=DIRECTION('center_axis',(0.,0.901003410349976,-0.433812003680988));
#43707=DIRECTION('ref_axis',(1.,0.,0.));
#43708=DIRECTION('center_axis',(-9.62964972193618E-33,0.901003410349976,
-0.433812003680988));
#43709=DIRECTION('ref_axis',(6.43494414306736E-48,-0.433812003680988,-0.901003410349976));
#43710=DIRECTION('',(0.,-0.901003410349976,0.433812003680988));
#43711=DIRECTION('center_axis',(0.,0.901003410349976,-0.433812003680988));
#43712=DIRECTION('ref_axis',(1.,0.,0.));
#43713=DIRECTION('center_axis',(-1.,0.,0.));
#43714=DIRECTION('ref_axis',(0.,0.433812003680988,0.901003410349976));
#43715=DIRECTION('center_axis',(1.,0.,0.));
#43716=DIRECTION('ref_axis',(0.,1.,0.));
#43717=DIRECTION('center_axis',(1.,0.,0.));
#43718=DIRECTION('ref_axis',(0.,0.433812003680988,0.901003410349976));
#43719=DIRECTION('',(1.,0.,0.));
#43720=DIRECTION('',(1.,0.,0.));
#43721=DIRECTION('center_axis',(0.,0.433812003680988,0.901003410349976));
#43722=DIRECTION('ref_axis',(1.,0.,0.));
#43723=DIRECTION('',(-1.,0.,0.));
#43724=DIRECTION('',(0.,0.901003410349976,-0.433812003680988));
#43725=DIRECTION('center_axis',(1.,0.,0.));
#43726=DIRECTION('ref_axis',(0.,-0.433812003680988,-0.901003410349976));
#43727=DIRECTION('',(-1.,0.,0.));
#43728=DIRECTION('center_axis',(0.,0.,1.));
#43729=DIRECTION('ref_axis',(1.,0.,0.));
#43730=DIRECTION('',(1.,0.,0.));
#43731=DIRECTION('center_axis',(1.,0.,0.));
#43732=DIRECTION('ref_axis',(0.,1.,0.));
#43733=DIRECTION('',(1.,0.,0.));
#43734=DIRECTION('center_axis',(0.,1.,0.));
#43735=DIRECTION('ref_axis',(1.,0.,0.));
#43736=DIRECTION('',(1.,0.,0.));
#43737=DIRECTION('center_axis',(1.,0.,0.));
#43738=DIRECTION('ref_axis',(0.,0.,-1.));
#43739=DIRECTION('center_axis',(-1.,0.,0.));
#43740=DIRECTION('ref_axis',(0.,1.,0.));
#43741=DIRECTION('center_axis',(0.,1.,0.));
#43742=DIRECTION('ref_axis',(1.,0.,0.));
#43743=DIRECTION('center_axis',(-1.,0.,0.));
#43744=DIRECTION('ref_axis',(0.,1.,0.));
#43745=DIRECTION('center_axis',(0.,1.,0.));
#43746=DIRECTION('ref_axis',(1.,0.,0.));
#43747=DIRECTION('center_axis',(3.93130878897075E-8,0.999999999999998,-3.93130878897075E-8));
#43748=DIRECTION('ref_axis',(0.707106723310616,4.55056292462304E-15,0.707106839062474));
#43749=DIRECTION('',(0.,-1.,0.));
#43750=DIRECTION('center_axis',(-0.0173649780999165,0.99984921740008,-1.91423167460546E-7));
#43751=DIRECTION('ref_axis',(0.760990338834415,0.0132166975786665,0.648628570990977));
#43752=DIRECTION('center_axis',(1.,0.,0.));
#43753=DIRECTION('ref_axis',(0.,-1.,0.));
#43754=DIRECTION('center_axis',(0.,0.994202177480807,0.107526881719979));
#43755=DIRECTION('ref_axis',(1.,0.,0.));
#43756=DIRECTION('center_axis',(-1.,0.,0.));
#43757=DIRECTION('ref_axis',(0.,-1.,0.));
#43758=DIRECTION('',(-1.,0.,0.));
#43759=DIRECTION('center_axis',(1.,0.,0.));
#43760=DIRECTION('ref_axis',(0.,-2.09002828430941E-15,-1.));
#43761=DIRECTION('',(-1.,0.,0.));
#43762=DIRECTION('center_axis',(-1.,0.,0.));
#43763=DIRECTION('ref_axis',(0.,1.,0.));
#43764=DIRECTION('center_axis',(-1.,0.,0.));
#43765=DIRECTION('ref_axis',(0.,-0.107526881719978,-0.994202177480807));
#43766=DIRECTION('',(-1.,0.,0.));
#43767=DIRECTION('center_axis',(1.,0.,0.));
#43768=DIRECTION('ref_axis',(0.,1.,0.));
#43769=DIRECTION('center_axis',(1.,0.,0.));
#43770=DIRECTION('ref_axis',(0.,0.930044067784185,0.367447999014073));
#43771=DIRECTION('',(-1.,0.,0.));
#43772=DIRECTION('center_axis',(1.,8.3307817066003E-9,3.39356925084603E-10));
#43773=DIRECTION('ref_axis',(-3.41030038156647E-10,0.000200933687209084,
0.999999979812826));
#43774=DIRECTION('center_axis',(0.,0.,1.));
#43775=DIRECTION('ref_axis',(1.,0.,0.));
#43776=DIRECTION('center_axis',(0.0173652351998802,-0.999849212934857,-1.53755357850641E-12));
#43777=DIRECTION('ref_axis',(0.760979857924961,0.0132165871066167,-0.648640869555534));
#43778=DIRECTION('center_axis',(0.0118197508200445,-0.999930144305366,-3.90308482337882E-8));
#43779=DIRECTION('ref_axis',(0.727691598926711,0.00860176102447277,-0.685850527854842));
#43780=DIRECTION('center_axis',(0.,-0.994202177480807,0.107526881719979));
#43781=DIRECTION('ref_axis',(1.,0.,0.));
#43782=DIRECTION('center_axis',(-1.,0.,0.));
#43783=DIRECTION('ref_axis',(0.,0.107526881719979,-0.994202177480807));
#43784=DIRECTION('center_axis',(-1.,0.,0.));
#43785=DIRECTION('ref_axis',(0.,1.,0.));
#43786=DIRECTION('center_axis',(-0.0103216872828093,-0.900955413872221,
0.43378889449359));
#43787=DIRECTION('ref_axis',(0.726589340957755,-0.304799871633038,-0.615763727300544));
#43788=DIRECTION('center_axis',(-9.83007148257777E-8,-0.901003452989707,
0.433811915120616));
#43789=DIRECTION('ref_axis',(0.707106781770852,-0.306751409315773,-0.637105620801179));
#43790=DIRECTION('center_axis',(8.58451173878204E-29,-0.901003410349976,
0.433812003680988));
#43791=DIRECTION('ref_axis',(1.,7.73467435283202E-29,-3.724064238024E-29));
#43792=DIRECTION('',(0.,0.901003410349976,-0.433812003680988));
#43793=DIRECTION('center_axis',(1.,0.,0.));
#43794=DIRECTION('ref_axis',(0.,1.,0.));
#78623=CARTESIAN_POINT('',(0.,0.,0.));
#78624=CARTESIAN_POINT('Origin',(7.54951656745E-15,-20.7780221998,-1.3270392201));
#78625=CARTESIAN_POINT('',(-3.61308907991371,-19.2125922380406,-0.960540656330234));
#78626=CARTESIAN_POINT('',(-3.88711717726,-19.0254782583927,-1.22484599905396));
#78627=CARTESIAN_POINT('Ctrl Pts',(-3.61308907991371,-19.2125922380406,
-0.960540656330234));
#78628=CARTESIAN_POINT('Ctrl Pts',(-3.61334186378693,-19.1910253579796,
-1.05216616964079));
#78629=CARTESIAN_POINT('Ctrl Pts',(-3.64741581668055,-19.1548229963094,
-1.14028371652892));
#78630=CARTESIAN_POINT('Ctrl Pts',(-3.71492697253399,-19.108516931192,-1.20628614736713));
#78631=CARTESIAN_POINT('Ctrl Pts',(-3.801022074897,-19.0627803730605,-1.23357916236737));
#78632=CARTESIAN_POINT('Ctrl Pts',(-3.88711717726,-19.0254782583,-1.22484599945));
#78633=CARTESIAN_POINT('',(-3.64161503967,-19.2306411737,-0.82776370433));
#78634=CARTESIAN_POINT('Origin',(-3.93441475488739,-19.0698572267847,-0.942962194752341));
#78635=CARTESIAN_POINT('',(-2.63891667039959,-17.8998816182875,-0.516206449181057));
#78636=CARTESIAN_POINT('Origin',(7.51064056026E-15,-20.8084305484,-1.19715554699));
#78637=CARTESIAN_POINT('',(-2.61824688650184,-17.8922584277925,-0.651424276437992));
#78638=CARTESIAN_POINT('Origin',(-2.76894427741165,-17.7302609546611,-0.594856157802496));
#78639=CARTESIAN_POINT('',(-2.81682310404,-17.6050062358,-0.892285274267));
#78640=CARTESIAN_POINT('Ctrl Pts',(-2.61824688650184,-17.8922584277925,
-0.651424276437992));
#78641=CARTESIAN_POINT('Ctrl Pts',(-2.61820300293512,-17.8744033188817,
-0.72790778770481));
#78642=CARTESIAN_POINT('Ctrl Pts',(-2.63960889197191,-17.8330169329895,
-0.798385310068769));
#78643=CARTESIAN_POINT('Ctrl Pts',(-2.71314604228615,-17.7266466553736,
-0.8875574924106));
#78644=CARTESIAN_POINT('Ctrl Pts',(-2.76482447353174,-17.6623177748382,
-0.905703044325404));
#78645=CARTESIAN_POINT('Ctrl Pts',(-2.81682310404,-17.6050062358,-0.892285274267));
#78646=CARTESIAN_POINT('Origin',(4.85143369921559E-9,-20.7096354418264,
-1.61914066024343));
#78647=CARTESIAN_POINT('Origin',(-6.2172489379E-15,-20.3611579168,2.27304371988));
#78648=CARTESIAN_POINT('',(-3.29086024220978,-18.2454109371054,1.04173423462419));
#78649=CARTESIAN_POINT('',(-3.53153637160979,-17.9397782141428,1.21096986282933));
#78650=CARTESIAN_POINT('Origin',(-3.52914694744576,-18.0912695033716,0.95419825055126));
#78651=CARTESIAN_POINT('',(-3.30849193722298,-18.2908119190758,0.937647175475319));
#78652=CARTESIAN_POINT('Origin',(-3.53120754646385,-18.090985806266,0.951651527640288));
#78653=CARTESIAN_POINT('',(-3.61003714743049,-18.6956696732126,1.17326396065629));
#78654=CARTESIAN_POINT('Origin',(-6.2172489379E-15,-20.4178945359,2.17555373363));
#78655=CARTESIAN_POINT('',(-3.59076491541284,-18.6481271742909,1.27610468451569));
#78656=CARTESIAN_POINT('Origin',(-3.85341043799,-18.5228280068,1.20318385007));
#78657=CARTESIAN_POINT('',(-3.85341043799,-18.3719297863,1.46247080897));
#78658=CARTESIAN_POINT('Origin',(-3.85341043799,-18.5228280068,1.20318385007));
#78659=CARTESIAN_POINT('Origin',(0.00142139409255115,-20.2110499150628,
2.53279056392384));
#78660=CARTESIAN_POINT('Origin',(4.55191440096E-15,-20.9224910251,0.373199680532));
#78661=CARTESIAN_POINT('',(3.37113078829735,-18.8600780815313,2.36677038101639));
#78662=CARTESIAN_POINT('',(3.36990985449358,-18.8395487394787,2.34355634748983));
#78663=CARTESIAN_POINT('Origin',(3.59839803273,-18.6983201284,2.47715137666));
#78664=CARTESIAN_POINT('',(3.59839803273,-18.4921598488,2.25921115747));
#78665=CARTESIAN_POINT('Origin',(3.59839803273,-18.6983201284,2.47715137666));
#78666=CARTESIAN_POINT('',(-3.59839802628,-18.4921598544775,2.25921116347192));
#78667=CARTESIAN_POINT('Origin',(-2.62234678416E-13,-20.7163307455,0.155259461344));
#78668=CARTESIAN_POINT('',(-3.36990985449358,-18.8395487394775,2.34355634748858));
#78669=CARTESIAN_POINT('Origin',(-3.59839803273,-18.6983201284,2.47715137666));
#78670=CARTESIAN_POINT('',(-3.37113078873609,-18.8600780898805,2.36677040528946));
#78671=CARTESIAN_POINT('Origin',(-3.59839803273,-18.6983201284,2.47715137666));
#78672=CARTESIAN_POINT('Origin',(4.54374776135E-15,-20.9437750269,0.39569984413));
#78673=CARTESIAN_POINT('Origin',(6.2172489379E-15,-20.3611579168,2.27304371988));
#78674=CARTESIAN_POINT('',(3.30849193622019,-18.2908119357476,0.937647359212487));
#78675=CARTESIAN_POINT('',(3.29086019657007,-18.2454109948681,1.04173426863756));
#78676=CARTESIAN_POINT('Origin',(3.53166730415163,-18.0906254246164,0.951572436110974));
#78677=CARTESIAN_POINT('',(3.53153633351,-17.9397782658,1.2109699402));
#78678=CARTESIAN_POINT('Ctrl Pts',(3.29086019657019,-18.2454109945417,1.04173426919817));
#78679=CARTESIAN_POINT('Ctrl Pts',(3.29082949183587,-18.2059257452771,1.10962705068825));
#78680=CARTESIAN_POINT('Ctrl Pts',(3.31677120622792,-18.149985595813,1.16738387145166));
#78681=CARTESIAN_POINT('Ctrl Pts',(3.40589056391193,-18.036820722088,1.23003743451762));
#78682=CARTESIAN_POINT('Ctrl Pts',(3.46851942482175,-17.9802928485517,1.23454836645887));
#78683=CARTESIAN_POINT('Ctrl Pts',(3.53153633351,-17.9397782658,1.2109699402));
#78684=CARTESIAN_POINT('',(3.85341040044001,-18.3719297862954,1.46247080897792));
#78685=CARTESIAN_POINT('Origin',(-0.00140566648756613,-20.211041526665,
2.53278568209601));
#78686=CARTESIAN_POINT('',(3.59076516652098,-18.6481269365579,1.27610454642206));
#78687=CARTESIAN_POINT('Origin',(3.8534092721712,-18.5228276087667,1.20318547093161));
#78688=CARTESIAN_POINT('',(3.61003708783018,-18.6956695658327,1.17326382994037));
#78689=CARTESIAN_POINT('Origin',(3.85338015716578,-18.5228452831943,1.20318513359903));
#78690=CARTESIAN_POINT('Origin',(6.20159509999E-15,-20.4178945359,2.17555373363));
#78691=CARTESIAN_POINT('Origin',(-1.68753899743E-14,-20.7780221998,-1.3270392201));
#78692=CARTESIAN_POINT('',(3.64161487464907,-19.2306407860628,-0.827763585289629));
#78693=CARTESIAN_POINT('',(3.61308908062573,-19.2125922405508,-0.960540656987445));
#78694=CARTESIAN_POINT('Origin',(3.82106060895697,-19.1266175913241,-0.921769890875969));
#78695=CARTESIAN_POINT('',(3.88711718104,-19.0254782583,-1.22484599945));
#78696=CARTESIAN_POINT('Ctrl Pts',(3.61308908062573,-19.2125922405508,-0.960540656987445));
#78697=CARTESIAN_POINT('Ctrl Pts',(3.6130284012607,-19.1947148817522,-1.03701895910761));
#78698=CARTESIAN_POINT('Ctrl Pts',(3.64256777805805,-19.1641230915394,-1.11002371080264));
#78699=CARTESIAN_POINT('Ctrl Pts',(3.74404646871257,-19.0948362447271,-1.2078778611402));
#78700=CARTESIAN_POINT('Ctrl Pts',(3.81536089299333,-19.0565678454691,-1.23212468954696));
#78701=CARTESIAN_POINT('Ctrl Pts',(3.88711718104,-19.0254782583,-1.22484599945));
#78702=CARTESIAN_POINT('',(2.81682317483321,-17.6050062274254,-0.892285262814533));
#78703=CARTESIAN_POINT('Origin',(-8.31938484768813E-8,-20.7096353378519,
-1.61914063590086));
#78704=CARTESIAN_POINT('',(2.61824690546747,-17.8922583873498,-0.651424266668572));
#78705=CARTESIAN_POINT('Ctrl Pts',(2.61824690546748,-17.8922583873498,-0.651424266668573));
#78706=CARTESIAN_POINT('Ctrl Pts',(2.61843004860693,-17.8705990179235,-0.743028110698349));
#78707=CARTESIAN_POINT('Ctrl Pts',(2.64312195677522,-17.8219449998149,-0.828230451813944));
#78708=CARTESIAN_POINT('Ctrl Pts',(2.69204431205891,-17.7509683072632,-0.888456978613999));
#78709=CARTESIAN_POINT('Ctrl Pts',(2.75443362214528,-17.673769970339,-0.90838416964567));
#78710=CARTESIAN_POINT('Ctrl Pts',(2.81682319433,-17.6050062358,-0.892285274267));
#78711=CARTESIAN_POINT('',(2.63891853137576,-17.8998831837931,-0.516206775081432));
#78712=CARTESIAN_POINT('Origin',(2.85113685828544,-17.6320686833311,-0.606360018255462));
#78713=CARTESIAN_POINT('Origin',(-1.69216709352E-14,-20.8084305484,-1.19715554699));
#78714=CARTESIAN_POINT('Origin',(-3.53495011041E-13,-21.0197764855,0.650835506465));
#78715=CARTESIAN_POINT('',(-4.0532699789542,-21.571070890106,-0.0674504972475476));
#78716=CARTESIAN_POINT('',(4.05326999191,-21.5710708896,-0.0674504957552));
#78717=CARTESIAN_POINT('Origin',(-3.53328477587E-13,-21.3048372788,0.744325314097));
#78718=CARTESIAN_POINT('',(4.34627739081414,-21.2879280691877,-0.225306331462357));
#78719=CARTESIAN_POINT('Ctrl Pts',(4.34627740764,-21.2879283386,-0.225306246837));
#78720=CARTESIAN_POINT('Ctrl Pts',(4.35210058992,-21.3811601618,-0.196020670745));
#78721=CARTESIAN_POINT('Ctrl Pts',(4.31892160248,-21.4741377387,-0.1581676115));
#78722=CARTESIAN_POINT('Ctrl Pts',(4.24485535575,-21.5457105806,-0.118264986841));
#78723=CARTESIAN_POINT('Ctrl Pts',(4.14906267383,-21.5773629037,-0.0866355443942));
#78724=CARTESIAN_POINT('Ctrl Pts',(4.05326999191,-21.5710708896,-0.0674504957552));
#78725=CARTESIAN_POINT('',(0.881570449864,-19.6457838359,4.78177176907));
#78726=CARTESIAN_POINT('Origin',(-3.53505134421E-13,-21.0024479625,0.645152366871));
#78727=CARTESIAN_POINT('',(-4.44088090492117,-20.9747479205191,0.729452226642898));
#78728=CARTESIAN_POINT('Ctrl Pts',(-4.44088090408204,-20.9747479074319,
0.729452222330876));
#78729=CARTESIAN_POINT('Ctrl Pts',(-4.44033851341439,-20.9662886381893,
0.755232231741162));
#78730=CARTESIAN_POINT('Ctrl Pts',(-4.43956056840391,-20.9580332073157,
0.780396132983051));
#78731=CARTESIAN_POINT('Ctrl Pts',(-4.43858185727784,-20.9499840167878,
0.804940747821991));
#78732=CARTESIAN_POINT('Ctrl Pts',(-4.43636923292827,-20.9317867832202,
0.860430065350874));
#78733=CARTESIAN_POINT('Ctrl Pts',(-4.43313310769655,-20.9146392251699,
0.91275188851088));
#78734=CARTESIAN_POINT('Ctrl Pts',(-4.42924276556979,-20.8985397211973,
0.961885171997912));
#78735=CARTESIAN_POINT('Ctrl Pts',(-4.42729759450641,-20.890489969211,0.986451813741426));
#78736=CARTESIAN_POINT('Ctrl Pts',(-4.42518817421974,-20.8827019166165,
1.01022167687519));
#78737=CARTESIAN_POINT('Ctrl Pts',(-4.42295644747595,-20.8751737494359,
1.03319399384914));
#78738=CARTESIAN_POINT('Ctrl Pts',(-4.42184058410406,-20.8714096658456,
1.04468015233612));
#78739=CARTESIAN_POINT('Ctrl Pts',(-4.42069410285316,-20.8677105572313,
1.05596692134127));
#78740=CARTESIAN_POINT('Ctrl Pts',(-4.41952197679202,-20.864076097256,1.06705432209663));
#78741=CARTESIAN_POINT('Ctrl Pts',(-4.41893591376145,-20.8622588672683,
1.07259802247431));
#78742=CARTESIAN_POINT('Ctrl Pts',(-4.41834343689534,-20.8604577996644,
1.07809188062318));
#78743=CARTESIAN_POINT('Ctrl Pts',(-4.41774515166877,-20.8586728527503,
1.08353590073895));
#78744=CARTESIAN_POINT('Ctrl Pts',(-4.41744600905548,-20.8577803792933,
1.08625791079684));
#78745=CARTESIAN_POINT('Ctrl Pts',(-4.41714541418869,-20.8568919360236,
1.08896746133314));
#78746=CARTESIAN_POINT('Ctrl Pts',(-4.41684344169986,-20.8560075174297,
1.0916645532355));
#78747=CARTESIAN_POINT('Ctrl Pts',(-4.41654146921104,-20.8551230988358,
1.09436164513785));
#78748=CARTESIAN_POINT('Ctrl Pts',(-4.41639664022107,-20.854698710831,1.09565585986192));
#78749=CARTESIAN_POINT('Ctrl Pts',(-4.41593346532297,-20.8533663301158,
1.09971845399856));
#78750=CARTESIAN_POINT('Ctrl Pts',(-4.40600422226456,-20.8248036165033,
1.18680971217248));
#78751=CARTESIAN_POINT('Ctrl Pts',(-4.39347291508139,-20.7970283698894,
1.27137761754194));
#78752=CARTESIAN_POINT('Ctrl Pts',(-4.37878794010872,-20.7701000627841,
1.35332388292646));
#78753=CARTESIAN_POINT('Ctrl Pts',(-4.36368716048736,-20.7424092814289,
1.43759045448469));
#78754=CARTESIAN_POINT('Ctrl Pts',(-4.34630941899308,-20.7156140029929,
1.5190850588711));
#78755=CARTESIAN_POINT('Ctrl Pts',(-4.32712048226691,-20.6897627700988,
1.59774998432596));
#78756=CARTESIAN_POINT('Ctrl Pts',(-4.30925992593525,-20.6657011241651,
1.67096922270594));
#78757=CARTESIAN_POINT('Ctrl Pts',(-4.28983019135619,-20.6424570841339,
1.74173778434547));
#78758=CARTESIAN_POINT('Ctrl Pts',(-4.26918657483247,-20.6200588534231,
1.81004248360131));
#78759=CARTESIAN_POINT('Ctrl Pts',(-4.24613721574523,-20.5950504028942,
1.88630719907324));
#78760=CARTESIAN_POINT('Ctrl Pts',(-4.22157405504016,-20.5710831539992,
1.95949758770353));
#78761=CARTESIAN_POINT('Ctrl Pts',(-4.19595352642011,-20.5481355019429,
2.02962580328218));
#78762=CARTESIAN_POINT('Ctrl Pts',(-4.1857871916205,-20.5390297759397,2.0574529776955));
#78763=CARTESIAN_POINT('Ctrl Pts',(-4.17545396884154,-20.5300844554319,
2.08479840962057));
#78764=CARTESIAN_POINT('Ctrl Pts',(-4.16498076975541,-20.5212976997503,
2.11166435494956));
#78765=CARTESIAN_POINT('Ctrl Pts',(-4.14654723630162,-20.505832419899,2.15895022223016));
#78766=CARTESIAN_POINT('Ctrl Pts',(-4.12768045405037,-20.4908572953069,
2.20475019302771));
#78767=CARTESIAN_POINT('Ctrl Pts',(-4.10851920046663,-20.4763542193862,
2.24908112387));
#78768=CARTESIAN_POINT('Ctrl Pts',(-4.09893857367477,-20.4691026814258,
2.27124658929114));
#78769=CARTESIAN_POINT('Ctrl Pts',(-4.08928424644404,-20.4619691715805,
2.29304476363202));
#78770=CARTESIAN_POINT('Ctrl Pts',(-4.07957257855448,-20.4549507827894,
2.3144784185172));
#78771=CARTESIAN_POINT('Ctrl Pts',(-4.0747167446097,-20.4514415883938,2.3251952459598));
#78772=CARTESIAN_POINT('Ctrl Pts',(-4.06984656963281,-20.4479611753603,
2.33582094142983));
#78773=CARTESIAN_POINT('Ctrl Pts',(-4.06496405358873,-20.4445091710698,
2.34635585710495));
#78774=CARTESIAN_POINT('Ctrl Pts',(-4.06252279556669,-20.4427831689246,
2.3516233149425));
#78775=CARTESIAN_POINT('Ctrl Pts',(-4.06007845192657,-20.4410642690357,
2.35686807769117));
#78776=CARTESIAN_POINT('Ctrl Pts',(-4.05763126898474,-20.4393524229206,
2.36209019124524));
#78777=CARTESIAN_POINT('Ctrl Pts',(-4.05640767751383,-20.438496499863,2.36470124802228));
#78778=CARTESIAN_POINT('Ctrl Pts',(-4.0551833761952,-20.4376423402533,2.36730664249168));
#78779=CARTESIAN_POINT('Ctrl Pts',(-4.05395839558517,-20.436789937912,2.36990638050782));
#78780=CARTESIAN_POINT('Ctrl Pts',(-4.05273341497514,-20.4359375355706,
2.37250611852396));
#78781=CARTESIAN_POINT('Ctrl Pts',(-4.05197605007509,-20.4354110607625,
2.37411174650506));
#78782=CARTESIAN_POINT('Ctrl Pts',(-4.0502814463181,-20.4342379964883,2.37768863106475));
#78783=CARTESIAN_POINT('Ctrl Pts',(-4.01118861434413,-20.4071765643552,
2.4602038187628));
#78784=CARTESIAN_POINT('Ctrl Pts',(-3.97020611342597,-20.3810987770343,
2.5396031757798));
#78785=CARTESIAN_POINT('Ctrl Pts',(-3.92779118828007,-20.3560255577381,
2.61590725626987));
#78786=CARTESIAN_POINT('Ctrl Pts',(-3.8842719929869,-20.3302995586135,2.69419790912594));
#78787=CARTESIAN_POINT('Ctrl Pts',(-3.83924511714191,-20.3056310140628,
2.76923032883936));
#78788=CARTESIAN_POINT('Ctrl Pts',(-3.79317122967888,-20.2820286625872,
2.84106897626654));
#78789=CARTESIAN_POINT('Ctrl Pts',(-3.7595712346176,-20.2648163339412,2.89345826511696));
#78790=CARTESIAN_POINT('Ctrl Pts',(-3.72541371197391,-20.2481707330716,
2.94414994133828));
#78791=CARTESIAN_POINT('Ctrl Pts',(-3.6908654173721,-20.2320912954077,2.99318105905564));
#78792=CARTESIAN_POINT('Ctrl Pts',(-3.64181519957344,-20.2092623850784,
3.06279338089863));
#78793=CARTESIAN_POINT('Ctrl Pts',(-3.59197772397555,-20.1875641826927,
3.129055007804));
#78794=CARTESIAN_POINT('Ctrl Pts',(-3.54178606204226,-20.1669387782563,
3.19209064841556));
#78795=CARTESIAN_POINT('Ctrl Pts',(-3.52643993993718,-20.1606325520276,
3.21136382249541));
#78796=CARTESIAN_POINT('Ctrl Pts',(-3.51106040139271,-20.1544265486155,
3.23033562160662));
#78797=CARTESIAN_POINT('Ctrl Pts',(-3.49565901852874,-20.1483189501994,
3.24901010602001));
#78798=CARTESIAN_POINT('Ctrl Pts',(-3.46277212706782,-20.1352772689446,
3.28888611893496));
#78799=CARTESIAN_POINT('Ctrl Pts',(-3.42978594374505,-20.1226833054986,
3.32740609871667));
#78800=CARTESIAN_POINT('Ctrl Pts',(-3.39680598782897,-20.1105123700283,
3.36461160092258));
#78801=CARTESIAN_POINT('Ctrl Pts',(-3.38031600987093,-20.1044269022932,
3.38321435202554));
#78802=CARTESIAN_POINT('Ctrl Pts',(-3.36382754753937,-20.0984472056528,
3.40148845134646));
#78803=CARTESIAN_POINT('Ctrl Pts',(-3.34735285274272,-20.0925696281575,
3.41943945376333));
#78804=CARTESIAN_POINT('Ctrl Pts',(-3.33911550534439,-20.0896308394098,
3.42841495497177));
#78805=CARTESIAN_POINT('Ctrl Pts',(-3.33088159671428,-20.0867175814878,
3.43730967957859));
#78806=CARTESIAN_POINT('Ctrl Pts',(-3.32265262387178,-20.0838293880027,
3.44612432080446));
#78807=CARTESIAN_POINT('Ctrl Pts',(-3.31853813745052,-20.0823852912602,
3.4505316414174));
#78808=CARTESIAN_POINT('Ctrl Pts',(-3.31442488479339,-20.0809474606917,
3.45491894103536));
#78809=CARTESIAN_POINT('Ctrl Pts',(-3.31031304956928,-20.079515836159,3.45928630729641));
#78810=CARTESIAN_POINT('Ctrl Pts',(-3.30651415218028,-20.0781931677147,
3.46332128812166));
#78811=CARTESIAN_POINT('Ctrl Pts',(-3.30349448908605,-20.0771448996417,
3.46651871720658));
#78812=CARTESIAN_POINT('Ctrl Pts',(-3.2990978311697,-20.0756250992641,3.47115298296621));
#78813=CARTESIAN_POINT('Ctrl Pts',(-3.29873565223483,-20.0754999042427,
3.47153473507626));
#78814=CARTESIAN_POINT('Ctrl Pts',(-3.29836410744608,-20.0753715156315,
3.47192621856882));
#78815=CARTESIAN_POINT('Ctrl Pts',(-3.29798197842631,-20.0752395201448,
3.47232869357418));
#78816=CARTESIAN_POINT('Ctrl Pts',(-3.23758565072548,-20.0543773446535,
3.53594074881669));
#78817=CARTESIAN_POINT('Ctrl Pts',(-3.17676275542274,-20.0346312495266,
3.59610390764184));
#78818=CARTESIAN_POINT('Ctrl Pts',(-3.11592842027533,-20.0159631944352,
3.65300094151748));
#78819=CARTESIAN_POINT('Ctrl Pts',(-3.09584462036267,-20.0098001373014,
3.6717848838621));
#78820=CARTESIAN_POINT('Ctrl Pts',(-3.07575920417414,-20.0037545110479,
3.69021304856488));
#78821=CARTESIAN_POINT('Ctrl Pts',(-3.05568602350684,-19.9978247650746,
3.70829256654954));
#78822=CARTESIAN_POINT('Ctrl Pts',(-3.01524834858015,-19.9858792172294,
3.74471398292656));
#78823=CARTESIAN_POINT('Ctrl Pts',(-2.97486058219296,-19.9744025284116,
3.7797200084947));
#78824=CARTESIAN_POINT('Ctrl Pts',(-2.93462718600761,-19.9633722941119,
3.81336992203629));
#78825=CARTESIAN_POINT('Ctrl Pts',(-2.91451048791493,-19.957857176962,3.83019487880708));
#78826=CARTESIAN_POINT('Ctrl Pts',(-2.89443234925921,-19.9524536882399,
3.8466807723206));
#78827=CARTESIAN_POINT('Ctrl Pts',(-2.87440469997387,-19.9471582525925,
3.86283526515468));
#78828=CARTESIAN_POINT('Ctrl Pts',(-2.8643908753312,-19.9445105347688,3.87091251157173));
#78829=CARTESIAN_POINT('Ctrl Pts',(-2.85438967038263,-19.941889831371,3.87890690506955));
#78830=CARTESIAN_POINT('Ctrl Pts',(-2.84440253537844,-19.9392956772258,
3.88681939970655));
#78831=CARTESIAN_POINT('Ctrl Pts',(-2.83669748021923,-19.9372942923669,
3.89292387387251));
#78832=CARTESIAN_POINT('Ctrl Pts',(-2.82962993939577,-19.9354704767983,
3.89848634882859));
#78833=CARTESIAN_POINT('Ctrl Pts',(-2.82174497977312,-19.9334493944361,
3.90464952892944));
#78834=CARTESIAN_POINT('Ctrl Pts',(-2.81940961590337,-19.9328507911518,
3.90647493689843));
#78835=CARTESIAN_POINT('Ctrl Pts',(-2.8170023346954,-19.9322349629246,3.90835279692559));
#78836=CARTESIAN_POINT('Ctrl Pts',(-2.81448476520693,-19.9315923875919,
3.91031213762162));
#78837=CARTESIAN_POINT('Ctrl Pts',(-2.74611514202516,-19.9141419721958,
3.96352194401839));
#78838=CARTESIAN_POINT('Ctrl Pts',(-2.6779675900044,-19.8977925243118,4.01331402163749));
#78839=CARTESIAN_POINT('Ctrl Pts',(-2.61040908145182,-19.8824919207325,
4.05993977067158));
#78840=CARTESIAN_POINT('Ctrl Pts',(-2.59087155071088,-19.8780670744889,
4.07342366817893));
#78841=CARTESIAN_POINT('Ctrl Pts',(-2.57138296302871,-19.8737299153642,
4.08664285027023));
#78842=CARTESIAN_POINT('Ctrl Pts',(-2.55195142198082,-19.8694791150827,
4.0996036035047));
#78843=CARTESIAN_POINT('Ctrl Pts',(-2.5086396471951,-19.8600043284975,4.12849236861916));
#78844=CARTESIAN_POINT('Ctrl Pts',(-2.46561133153172,-19.8509567140269,
4.15609677884506));
#78845=CARTESIAN_POINT('Ctrl Pts',(-2.42294637854088,-19.8423099220236,
4.18248542023493));
#78846=CARTESIAN_POINT('Ctrl Pts',(-2.40161390204546,-19.837986526022,4.19567974092987));
#78847=CARTESIAN_POINT('Ctrl Pts',(-2.38037223624416,-19.833763353459,4.2085700759519));
#78848=CARTESIAN_POINT('Ctrl Pts',(-2.35923010187459,-19.829636189821,4.22116502061894));
#78849=CARTESIAN_POINT('Ctrl Pts',(-2.34530431694811,-19.8269177323476,
4.22946098958442));
#78850=CARTESIAN_POINT('Ctrl Pts',(-2.33192749888427,-19.8243381868342,
4.23733234032053));
#78851=CARTESIAN_POINT('Ctrl Pts',(-2.3181038302266,-19.8217035718007,4.24536913204935));
#78852=CARTESIAN_POINT('Ctrl Pts',(-2.31094039749043,-19.8203383128347,
4.24953380196365));
#78853=CARTESIAN_POINT('Ctrl Pts',(-2.30365653629527,-19.8189584821368,
4.25374223887199));
#78854=CARTESIAN_POINT('Ctrl Pts',(-2.29611081239421,-19.8175385538874,
4.25807207736949));
#78855=CARTESIAN_POINT('Ctrl Pts',(-2.22478241720023,-19.8041162229556,
4.29900127588314));
#78856=CARTESIAN_POINT('Ctrl Pts',(-2.15398926896422,-19.791648078878,4.33701687720016));
#78857=CARTESIAN_POINT('Ctrl Pts',(-2.08420171936975,-19.780091596446,4.37225205974607));
#78858=CARTESIAN_POINT('Ctrl Pts',(-2.01208080452018,-19.7681487199547,
4.40866533997827));
#78859=CARTESIAN_POINT('Ctrl Pts',(-1.94103439245925,-19.7571793779235,
4.44210949940517));
#78860=CARTESIAN_POINT('Ctrl Pts',(-1.87156021712279,-19.7471205066914,
4.47278070489698));
#78861=CARTESIAN_POINT('Ctrl Pts',(-1.84157455921399,-19.7427790104411,
4.48601866376549));
#78862=CARTESIAN_POINT('Ctrl Pts',(-1.81188147450031,-19.7386069332423,
4.49874063615051));
#78863=CARTESIAN_POINT('Ctrl Pts',(-1.78251945458098,-19.7345984158543,
4.5109647993908));
#78864=CARTESIAN_POINT('Ctrl Pts',(-1.70718535143936,-19.7243137670739,
4.54232832195819));
#78865=CARTESIAN_POINT('Ctrl Pts',(-1.63291517057692,-19.7149314387773,
4.57087456090056));
#78866=CARTESIAN_POINT('Ctrl Pts',(-1.55983928822529,-19.7063873463962,
4.59691663623052));
#78867=CARTESIAN_POINT('Ctrl Pts',(-1.55375173433672,-19.7056755845793,
4.59908605973716));
#78868=CARTESIAN_POINT('Ctrl Pts',(-1.54767244104875,-19.7049696434347,
4.60123809422092));
#78869=CARTESIAN_POINT('Ctrl Pts',(-1.54160146907483,-19.7042694879189,
4.6033729145871));
#78870=CARTESIAN_POINT('Ctrl Pts',(-1.50212756776972,-19.6997170258344,
4.61725367186955));
#78871=CARTESIAN_POINT('Ctrl Pts',(-1.46300461299036,-19.6954074668301,
4.63040669962543));
#78872=CARTESIAN_POINT('Ctrl Pts',(-1.42423897861779,-19.6913228213346,
4.642878158682));
#78873=CARTESIAN_POINT('Ctrl Pts',(-1.40485616143151,-19.6892804985869,
4.64911388821028));
#78874=CARTESIAN_POINT('Ctrl Pts',(-1.38556265643057,-19.6872944243512,
4.65517917530087));
#78875=CARTESIAN_POINT('Ctrl Pts',(-1.36635812914976,-19.6853618384192,
4.66107956383069));
#78876=CARTESIAN_POINT('Ctrl Pts',(-1.35378375648046,-19.6840964568053,
4.66494290725918));
#78877=CARTESIAN_POINT('Ctrl Pts',(-1.34051452660817,-19.6827816842502,
4.66895619379731));
#78878=CARTESIAN_POINT('Ctrl Pts',(-1.32798939829712,-19.6815595627749,
4.6726853210244));
#78879=CARTESIAN_POINT('Ctrl Pts',(-1.32138520901345,-19.6809151684542,
4.67465159725399));
#78880=CARTESIAN_POINT('Ctrl Pts',(-1.31498818680823,-19.6802962481877,
4.67653973989695));
#78881=CARTESIAN_POINT('Ctrl Pts',(-1.30901098191806,-19.6797219011273,
4.6782913668485));
#78882=CARTESIAN_POINT('Ctrl Pts',(-1.23975806031836,-19.6730674175229,
4.69858601730414));
#78883=CARTESIAN_POINT('Ctrl Pts',(-1.1715125981574,-19.6671035761371,4.71683336740599));
#78884=CARTESIAN_POINT('Ctrl Pts',(-1.104147192934,-19.6617360511869,4.73326901928545));
#78885=CARTESIAN_POINT('Ctrl Pts',(-1.03678178771059,-19.6563685262367,
4.7497046711649));
#78886=CARTESIAN_POINT('Ctrl Pts',(-0.970295895358319,-19.6515973499143,
4.76432852674912));
#78887=CARTESIAN_POINT('Ctrl Pts',(-0.904531595433205,-19.6473433846981,
4.77732987546702));
#78888=CARTESIAN_POINT('Ctrl Pts',(-0.844034296727092,-19.6434301155738,
4.78928995833667));
#78889=CARTESIAN_POINT('Ctrl Pts',(-0.784130214998427,-19.6399493355338,
4.79987958392767));
#78890=CARTESIAN_POINT('Ctrl Pts',(-0.724577840661874,-19.6368606964938,
4.80922780530557));
#78891=CARTESIAN_POINT('Ctrl Pts',(-0.71939310622028,-19.6365917941472,
4.81004167789899));
#78892=CARTESIAN_POINT('Ctrl Pts',(-0.714211027536302,-19.6363258737797,
4.81084611154134));
#78893=CARTESIAN_POINT('Ctrl Pts',(-0.709031439732714,-19.6360629142671,
4.8116411746211));
#78894=CARTESIAN_POINT('Ctrl Pts',(-0.676695016060087,-19.6344212449816,
4.81660479287963));
#78895=CARTESIAN_POINT('Ctrl Pts',(-0.644454374652469,-19.6328953299266,
4.82120400448747));
#78896=CARTESIAN_POINT('Ctrl Pts',(-0.612260437535052,-19.6314855189305,
4.82545593040161));
#78897=CARTESIAN_POINT('Ctrl Pts',(-0.596163468976344,-19.6307806134325,
4.82758189335868));
#78898=CARTESIAN_POINT('Ctrl Pts',(-0.580078166296216,-19.630104762066,
4.82962096413189));
#78899=CARTESIAN_POINT('Ctrl Pts',(-0.563997665342666,-19.6294586694314,
4.83157512690825));
#78900=CARTESIAN_POINT('Ctrl Pts',(-0.552534605636963,-19.6289980992994,
4.83296816090916));
#78901=CARTESIAN_POINT('Ctrl Pts',(-0.540277388802875,-19.6285222854744,
4.83441058736567));
#78902=CARTESIAN_POINT('Ctrl Pts',(-0.528926901809803,-19.6280969826263,
4.83570367497362));
#78903=CARTESIAN_POINT('Ctrl Pts',(-0.524354806036902,-19.6279256661572,
4.83622454428874));
#78904=CARTESIAN_POINT('Ctrl Pts',(-0.519929910169658,-19.6277623502447,
4.83672177752299));
#78905=CARTESIAN_POINT('Ctrl Pts',(-0.515763655468914,-19.6276106046347,
4.83718460528559));
#78906=CARTESIAN_POINT('Ctrl Pts',(-0.462270835908533,-19.6256622598706,
4.8431271037093));
#78907=CARTESIAN_POINT('Ctrl Pts',(-0.409259551027216,-19.6240572226069,
4.84809105159708));
#78908=CARTESIAN_POINT('Ctrl Pts',(-0.356405021564706,-19.6227344098681,
4.85213514155229));
#78909=CARTESIAN_POINT('Ctrl Pts',(-0.351915189055131,-19.6226220409245,
4.85247867476954));
#78910=CARTESIAN_POINT('Ctrl Pts',(-0.347426483201641,-19.6225117180823,
4.85281554111355));
#78911=CARTESIAN_POINT('Ctrl Pts',(-0.342938702630177,-19.6224034092166,
4.85314576034748));
#78912=CARTESIAN_POINT('Ctrl Pts',(-0.310871126117556,-19.6216294848273,
4.85550535221737));
#78913=CARTESIAN_POINT('Ctrl Pts',(-0.278439324545288,-19.6209494103661,
4.85755146880844));
#78914=CARTESIAN_POINT('Ctrl Pts',(-0.246251603405228,-19.6203854740379,
4.85924693559752));
#78915=CARTESIAN_POINT('Ctrl Pts',(-0.220906421391697,-19.6199414205798,
4.86058197619205));
#78916=CARTESIAN_POINT('Ctrl Pts',(-0.195712706518268,-19.6195690415602,
4.86170062386772));
#78917=CARTESIAN_POINT('Ctrl Pts',(-0.170968442363936,-19.6192721290622,
4.86260634567848));
#78918=CARTESIAN_POINT('Ctrl Pts',(-0.120043389665838,-19.6186610668574,
4.8644703708382));
#78919=CARTESIAN_POINT('Ctrl Pts',(-0.0695096448294374,-19.6183493595768,
4.86549911419981));
#78920=CARTESIAN_POINT('Ctrl Pts',(-0.019010528798765,-19.6182855485251,
4.86570589228436));
#78921=CARTESIAN_POINT('Ctrl Pts',(-0.0138106051836958,-19.6182789778637,
4.86572718434508));
#78922=CARTESIAN_POINT('Ctrl Pts',(-0.00861104704102354,-19.6182750498029,
4.86573971794318));
#78923=CARTESIAN_POINT('Ctrl Pts',(-0.00341146415241323,-19.6182737179049,
4.86574347790516));
#78924=CARTESIAN_POINT('Ctrl Pts',(0.0244362308228306,-19.6182665845848,
4.86576361534244));
#78925=CARTESIAN_POINT('Ctrl Pts',(0.0522848670786102,-19.6183355811537,
4.86553316457071));
#78926=CARTESIAN_POINT('Ctrl Pts',(0.0801947426845153,-19.6184852044545,
4.86505132588967));
#78927=CARTESIAN_POINT('Ctrl Pts',(0.0966689801100628,-19.6185735219309,
4.86476691312681));
#78928=CARTESIAN_POINT('Ctrl Pts',(0.112524662857614,-19.6186850569718,
4.86440975997926));
#78929=CARTESIAN_POINT('Ctrl Pts',(0.128907271508895,-19.6188300157461,
4.86395649894601));
#78930=CARTESIAN_POINT('Ctrl Pts',(0.140279305318237,-19.6189306392865,
4.8636418665267));
#78931=CARTESIAN_POINT('Ctrl Pts',(0.151905232556995,-19.6190476668708,
4.86328001337933));
#78932=CARTESIAN_POINT('Ctrl Pts',(0.164167684591193,-19.6191891080271,
4.86284911049531));
#78933=CARTESIAN_POINT('Ctrl Pts',(0.219243055735599,-19.6198243744615,
4.86091376051812));
#78934=CARTESIAN_POINT('Ctrl Pts',(0.273839067448982,-19.6207726130671,
4.85802404995734));
#78935=CARTESIAN_POINT('Ctrl Pts',(0.328278900113335,-19.6220303246855,
4.85419059485297));
#78936=CARTESIAN_POINT('Ctrl Pts',(0.382727880026239,-19.6232882476307,
4.8503564956326));
#78937=CARTESIAN_POINT('Ctrl Pts',(0.437020950294054,-19.6248557620228,
4.84557829070741));
#78938=CARTESIAN_POINT('Ctrl Pts',(0.491478298025858,-19.6267454877189,
4.83981744742401));
#78939=CARTESIAN_POINT('Ctrl Pts',(0.545598398233708,-19.6286235105807,
4.83409228032049));
#78940=CARTESIAN_POINT('Ctrl Pts',(0.59988106922271,-19.630819769465,4.82739659815985));
#78941=CARTESIAN_POINT('Ctrl Pts',(0.654632697086247,-19.6333624172747,
4.81964450729371));
#78942=CARTESIAN_POINT('Ctrl Pts',(0.708445951353243,-19.6358614873194,
4.81202527745237));
#78943=CARTESIAN_POINT('Ctrl Pts',(0.762712537127494,-19.6386951824065,
4.80338551612137));
#78944=CARTESIAN_POINT('Ctrl Pts',(0.817711082827369,-19.6419053928723,
4.79359744533806));
#78945=CARTESIAN_POINT('Ctrl Pts',(0.838884132943331,-19.64314124277,4.78982928546044));
#78946=CARTESIAN_POINT('Ctrl Pts',(0.860165508044187,-19.644433055478,4.7858904484103));
#78947=CARTESIAN_POINT('Ctrl Pts',(0.881570449864978,-19.6457838358982,
4.7817717690745));
#78948=CARTESIAN_POINT('',(-4.34627742980843,-21.2879273673038,-0.2253061846382));
#78949=CARTESIAN_POINT('Ctrl Pts',(-4.34627742739142,-21.2879273614,-0.225306186038311));
#78950=CARTESIAN_POINT('Ctrl Pts',(-4.34876256073138,-21.2842530500451,
-0.214102742103554));
#78951=CARTESIAN_POINT('Ctrl Pts',(-4.3519425262521,-21.2794971786555,-0.199560523662125));
#78952=CARTESIAN_POINT('Ctrl Pts',(-4.35570626500914,-21.2736452569576,
-0.181658306238884));
#78953=CARTESIAN_POINT('Ctrl Pts',(-4.35946565330856,-21.2678000994214,
-0.163776781760393));
#78954=CARTESIAN_POINT('Ctrl Pts',(-4.36380750279823,-21.2608613548734,
-0.142542810694277));
#78955=CARTESIAN_POINT('Ctrl Pts',(-4.36856958664169,-21.2528125480096,
-0.117929036995139));
#78956=CARTESIAN_POINT('Ctrl Pts',(-4.37331768326236,-21.2447873821523,
-0.0933875590277396));
#78957=CARTESIAN_POINT('Ctrl Pts',(-4.37848357402662,-21.2356585710447,
-0.0654858160552947));
#78958=CARTESIAN_POINT('Ctrl Pts',(-4.38385473197136,-21.2254089829913,
-0.034194250688982));
#78959=CARTESIAN_POINT('Ctrl Pts',(-4.38540961945695,-21.2224418469732,
-0.0251357080259122));
#78960=CARTESIAN_POINT('Ctrl Pts',(-4.38698137592943,-21.2193807860287,
-0.0157930867037397));
#78961=CARTESIAN_POINT('Ctrl Pts',(-4.3885640285451,-21.216225391,-0.00616568935559134));
#78962=CARTESIAN_POINT('Ctrl Pts',(-4.39398839891311,-21.20541061641,0.0268311719766124));
#78963=CARTESIAN_POINT('Ctrl Pts',(-4.3995446940136,-21.1934868320056,0.0631739988383164));
#78964=CARTESIAN_POINT('Ctrl Pts',(-4.40495994007788,-21.1804469665788,
0.102890079547786));
#78965=CARTESIAN_POINT('Ctrl Pts',(-4.40854074396456,-21.1718244219616,
0.129152135690801));
#78966=CARTESIAN_POINT('Ctrl Pts',(-4.41205882742973,-21.162713903488,0.156889047950214));
#78967=CARTESIAN_POINT('Ctrl Pts',(-4.41542294788823,-21.1531141059222,
0.18610645229467));
#78968=CARTESIAN_POINT('Ctrl Pts',(-4.41964878608593,-21.1410553251072,
0.222807879856458));
#78969=CARTESIAN_POINT('Ctrl Pts',(-4.42363246084328,-21.1282252001997,
0.261845944632033));
#78970=CARTESIAN_POINT('Ctrl Pts',(-4.42717158187633,-21.114630400055,0.303226839575934));
#78971=CARTESIAN_POINT('Ctrl Pts',(-4.42894114239285,-21.1078329999827,
0.323917287047885));
#78972=CARTESIAN_POINT('Ctrl Pts',(-4.4305991886873,-21.1008445658588,0.345193332465333));
#78973=CARTESIAN_POINT('Ctrl Pts',(-4.43211818822347,-21.0936668708972,
0.367054961915476));
#78974=CARTESIAN_POINT('Ctrl Pts',(-4.43287768799156,-21.0900780234164,
0.377985776640548));
#78975=CARTESIAN_POINT('Ctrl Pts',(-4.43360240346858,-21.0864418615886,
0.389062989167634));
#78976=CARTESIAN_POINT('Ctrl Pts',(-4.43428875480373,-21.0827586876202,
0.400286525438272));
#78977=CARTESIAN_POINT('Ctrl Pts',(-4.43463193047131,-21.080917100636,0.40589829357359));
#78978=CARTESIAN_POINT('Ctrl Pts',(-4.43496551371776,-21.0790637606659,
0.411546642765532));
#78979=CARTESIAN_POINT('Ctrl Pts',(-4.43528904862596,-21.0771987086789,
0.41723156134437));
#78980=CARTESIAN_POINT('Ctrl Pts',(-4.43558652017649,-21.0754839017375,
0.422458513680551));
#78981=CARTESIAN_POINT('Ctrl Pts',(-4.43594350612929,-21.0733400774869,
0.428994312633909));
#78982=CARTESIAN_POINT('Ctrl Pts',(-4.43617196726052,-21.0719233268787,
0.433314000298841));
#78983=CARTESIAN_POINT('Ctrl Pts',(-4.43619198418035,-21.0717991964273,
0.433692475364639));
#78984=CARTESIAN_POINT('Ctrl Pts',(-4.43621104747127,-21.0716806479611,
0.434053936609418));
#78985=CARTESIAN_POINT('Ctrl Pts',(-4.43622904681129,-21.0715684593114,
0.434396012400812));
#78986=CARTESIAN_POINT('Ctrl Pts',(-4.43973687615582,-21.0497044000089,
0.501061984502047));
#78987=CARTESIAN_POINT('Ctrl Pts',(-4.44142459043637,-21.028785541782,0.564800751777492));
#78988=CARTESIAN_POINT('Ctrl Pts',(-4.44172071894098,-21.0088522514293,
0.625534487408663));
#78989=CARTESIAN_POINT('Ctrl Pts',(-4.44189468413807,-20.9971421366286,
0.661213444767486));
#78990=CARTESIAN_POINT('Ctrl Pts',(-4.44158774005072,-20.9857719093663,
0.695856072893091));
#78991=CARTESIAN_POINT('Ctrl Pts',(-4.44088090408204,-20.9747479074319,
0.729452222330876));
#78992=CARTESIAN_POINT('Origin',(-4.05326997582804,-21.2860101201162,-0.160940375904291));
#78993=CARTESIAN_POINT('Origin',(0.,-22.8742356128,-0.678262730068));
#78994=CARTESIAN_POINT('',(3.62140732971,-22.8742356128,-0.813060915858));
#78995=CARTESIAN_POINT('',(-3.62140732971,-22.8742356128,-0.813060915858));
#78996=CARTESIAN_POINT('',(-2.26135909998E-9,-22.8742356128,-0.813060915858));
#78997=CARTESIAN_POINT('Origin',(4.36973020788E-13,-22.8742356128,0.729452270839));
#78998=CARTESIAN_POINT('Origin',(-2.26135909998E-9,-22.5742356128,-0.813060915858));
#78999=CARTESIAN_POINT('',(3.62140732971,-22.6596242971,-0.525469586725));
#79000=CARTESIAN_POINT('Ctrl Pts',(3.62140732971,-22.6596242971005,-0.525469586723355));
#79001=CARTESIAN_POINT('Ctrl Pts',(3.62140732971008,-22.6699477832947,-0.528534730954812));
#79002=CARTESIAN_POINT('Ctrl Pts',(3.62141714315506,-22.6806901701076,-0.532327683633485));
#79003=CARTESIAN_POINT('Ctrl Pts',(3.62142184225419,-22.6917209824537,-0.537022534618477));
#79004=CARTESIAN_POINT('Ctrl Pts',(3.62142321631071,-22.6949464857043,-0.538395348935147));
#79005=CARTESIAN_POINT('Ctrl Pts',(3.62142415307669,-22.6981963160703,-0.539845282632328));
#79006=CARTESIAN_POINT('Ctrl Pts',(3.62142427933164,-22.7014663477083,-0.541376650405068));
#79007=CARTESIAN_POINT('Ctrl Pts',(3.62142455834708,-22.7086929104212,-0.544760876146999));
#79008=CARTESIAN_POINT('Ctrl Pts',(3.62142164111691,-22.7160184972014,-0.548542904520612));
#79009=CARTESIAN_POINT('Ctrl Pts',(3.62141741127485,-22.7233891494459,-0.552766423972345));
#79010=CARTESIAN_POINT('Ctrl Pts',(3.62141529635382,-22.7270744755682,-0.554878183698211));
#79011=CARTESIAN_POINT('Ctrl Pts',(3.62141285327981,-22.7307710466164,-0.557100352677717));
#79012=CARTESIAN_POINT('Ctrl Pts',(3.62141087609901,-22.7344708103863,-0.559437806787722));
#79013=CARTESIAN_POINT('Ctrl Pts',(3.62140988750862,-22.7363206922713,-0.560606533842724));
#79014=CARTESIAN_POINT('Ctrl Pts',(3.62140901539152,-22.7381713722864,-0.561804082618375));
#79015=CARTESIAN_POINT('Ctrl Pts',(3.62140838179892,-22.7400217976135,-0.563031035793675));
#79016=CARTESIAN_POINT('Ctrl Pts',(3.62140800542491,-22.7411210086764,-0.563759884715135));
#79017=CARTESIAN_POINT('Ctrl Pts',(3.62140770758826,-22.7426310270696,-0.564776697577344));
#79018=CARTESIAN_POINT('Ctrl Pts',(3.62140752622844,-22.7438174542328,-0.565589707317948));
#79019=CARTESIAN_POINT('Ctrl Pts',(3.62140740228493,-22.7446282730451,-0.566145328103387));
#79020=CARTESIAN_POINT('Ctrl Pts',(3.62140733274219,-22.7452889497865,-0.566604278368968));
#79021=CARTESIAN_POINT('Ctrl Pts',(3.62140732971009,-22.7455712334679,-0.566800677308756));
#79022=CARTESIAN_POINT('Ctrl Pts',(3.62140730352346,-22.7480091664161,-0.568496869748418));
#79023=CARTESIAN_POINT('Ctrl Pts',(3.6214211167595,-22.7511789206969,-0.570750760982344));
#79024=CARTESIAN_POINT('Ctrl Pts',(3.6214374946079,-22.755018246027,-0.57364988953821));
#79025=CARTESIAN_POINT('Ctrl Pts',(3.62145363121916,-22.7588010201036,-0.57650631544711));
#79026=CARTESIAN_POINT('Ctrl Pts',(3.62147225744839,-22.763234296542,-0.579989678194066));
#79027=CARTESIAN_POINT('Ctrl Pts',(3.62148258939903,-22.7682192058606,-0.584215191354991));
#79028=CARTESIAN_POINT('Ctrl Pts',(3.62148569805628,-22.7697190557,-0.585486555552531));
#79029=CARTESIAN_POINT('Ctrl Pts',(3.62148805585235,-22.7712685402352,-0.586825289535902));
#79030=CARTESIAN_POINT('Ctrl Pts',(3.62148936905792,-22.7728641378073,-0.588234963055801));
#79031=CARTESIAN_POINT('Ctrl Pts',(3.62149361630903,-22.7780247186582,-0.592794216779927));
#79032=CARTESIAN_POINT('Ctrl Pts',(3.62148677078224,-22.7836714580148,-0.59809482393021));
#79033=CARTESIAN_POINT('Ctrl Pts',(3.62147178598681,-22.7896502718194,-0.604263107728835));
#79034=CARTESIAN_POINT('Ctrl Pts',(3.621468940372,-22.7907856494244,-0.605434465713029));
#79035=CARTESIAN_POINT('Ctrl Pts',(3.62146580123835,-22.7919328531322,-0.606637136087257));
#79036=CARTESIAN_POINT('Ctrl Pts',(3.62146238881206,-22.7930906114698,-0.607872003981022));
#79037=CARTESIAN_POINT('Ctrl Pts',(3.62145169780773,-22.7967178251754,-0.611740799051204));
#79038=CARTESIAN_POINT('Ctrl Pts',(3.6214387449041,-22.8004490769422,-0.615925609208144));
#79039=CARTESIAN_POINT('Ctrl Pts',(3.62142766212208,-22.8042397922835,-0.620452303848787));
#79040=CARTESIAN_POINT('Ctrl Pts',(3.62142246582197,-22.8060171162892,-0.622574700897024));
#79041=CARTESIAN_POINT('Ctrl Pts',(3.62141766979187,-22.8080079092195,-0.625018234205574));
#79042=CARTESIAN_POINT('Ctrl Pts',(3.62141404227473,-22.8099186181219,-0.627444319071953));
#79043=CARTESIAN_POINT('Ctrl Pts',(3.62141025972111,-22.8119109888293,-0.629974092401307));
#79044=CARTESIAN_POINT('Ctrl Pts',(3.62140774769706,-22.8138161559041,-0.63248461828544));
#79045=CARTESIAN_POINT('Ctrl Pts',(3.62140737721721,-22.815348938655,-0.634554994121101));
#79046=CARTESIAN_POINT('Ctrl Pts',(3.62140734521127,-22.8154813565557,-0.634733854968577));
#79047=CARTESIAN_POINT('Ctrl Pts',(3.62140732918835,-22.8156110208474,-0.63490941283829));
#79048=CARTESIAN_POINT('Ctrl Pts',(3.62140732971007,-22.8157377607153,-0.63508138739397));
#79049=CARTESIAN_POINT('Ctrl Pts',(3.62140736343285,-22.8239299728543,-0.646197479479502));
#79050=CARTESIAN_POINT('Ctrl Pts',(3.62140738564739,-22.8310489680643,-0.657463854897076));
#79051=CARTESIAN_POINT('Ctrl Pts',(3.62140739929918,-22.8372039362312,-0.668673725041791));
#79052=CARTESIAN_POINT('Ctrl Pts',(3.62140741342894,-22.8435743977133,-0.680276067091498));
#79053=CARTESIAN_POINT('Ctrl Pts',(3.62140741838586,-22.8489130072506,-0.691817776465343));
#79054=CARTESIAN_POINT('Ctrl Pts',(3.62140741743574,-22.8533648006108,-0.703120493300786));
#79055=CARTESIAN_POINT('Ctrl Pts',(3.62140741643095,-22.858072765324,-0.71507360696048));
#79056=CARTESIAN_POINT('Ctrl Pts',(3.62140740881975,-22.861789805585,-0.726759362272155));
#79057=CARTESIAN_POINT('Ctrl Pts',(3.62140739846477,-22.8646999547098,-0.738024484180477));
#79058=CARTESIAN_POINT('Ctrl Pts',(3.62140738776206,-22.8677078290071,-0.749667898036567));
#79059=CARTESIAN_POINT('Ctrl Pts',(3.62140737412821,-22.869854607863,-0.760862342676822));
#79060=CARTESIAN_POINT('Ctrl Pts',(3.6214073618282,-22.8713422147409,-0.771495701036556));
#79061=CARTESIAN_POINT('Ctrl Pts',(3.6214073488987,-22.8729059559173,-0.782673264517133));
#79062=CARTESIAN_POINT('Ctrl Pts',(3.62140733744306,-22.8737421881999,-0.793231321316465));
#79063=CARTESIAN_POINT('Ctrl Pts',(3.62140733241521,-22.8740700378175,-0.803095095549144));
#79064=CARTESIAN_POINT('Ctrl Pts',(3.62140733067966,-22.8741832072463,-0.806499942272538));
#79065=CARTESIAN_POINT('Ctrl Pts',(3.62140732971,-22.8742356128,-0.809822492012007));
#79066=CARTESIAN_POINT('Ctrl Pts',(3.62140732971,-22.8742356128,-0.813060915858));
#79067=CARTESIAN_POINT('',(-3.62140732971,-22.6596242971,-0.525469586725));
#79068=CARTESIAN_POINT('',(9.81437153769E-14,-22.6596242971,-0.525469586725));
#79069=CARTESIAN_POINT('Ctrl Pts',(-3.62140732971,-22.8742356128,-0.813060915858));
#79070=CARTESIAN_POINT('Ctrl Pts',(-3.62140732970999,-22.8742356128,-0.803744725297564));
#79071=CARTESIAN_POINT('Ctrl Pts',(-3.62136469902042,-22.873804016399,-0.793745508480425));
#79072=CARTESIAN_POINT('Ctrl Pts',(-3.62131260175645,-22.8727364911915,
-0.783107191556518));
#79073=CARTESIAN_POINT('Ctrl Pts',(-3.62126327948377,-22.8717258283395,
-0.773035530816041));
#79074=CARTESIAN_POINT('Ctrl Pts',(-3.62120547226317,-22.870144557252,-0.762390552719321));
#79075=CARTESIAN_POINT('Ctrl Pts',(-3.62116732196172,-22.8677991370249,
-0.751251068384887));
#79076=CARTESIAN_POINT('Ctrl Pts',(-3.62114578449456,-22.8664750475895,
-0.744962355875019));
#79077=CARTESIAN_POINT('Ctrl Pts',(-3.62113051184974,-22.8649070869389,
-0.738516841232333));
#79078=CARTESIAN_POINT('Ctrl Pts',(-3.62112656743464,-22.8630586371168,
-0.731935946677658));
#79079=CARTESIAN_POINT('Ctrl Pts',(-3.62111996128396,-22.8599628326116,
-0.720914190627644));
#79080=CARTESIAN_POINT('Ctrl Pts',(-3.62114127299378,-22.8560800676364,
-0.709511995309836));
#79081=CARTESIAN_POINT('Ctrl Pts',(-3.62118066024351,-22.8512437853523,
-0.697880742480753));
#79082=CARTESIAN_POINT('Ctrl Pts',(-3.62119586107707,-22.8493773051454,
-0.693391859923282));
#79083=CARTESIAN_POINT('Ctrl Pts',(-3.62121375415682,-22.8473688902165,
-0.688869387884984));
#79084=CARTESIAN_POINT('Ctrl Pts',(-3.62123377372212,-22.8452094665408,
-0.684324089002303));
#79085=CARTESIAN_POINT('Ctrl Pts',(-3.62126972009617,-22.8413320870857,
-0.676162722289865));
#79086=CARTESIAN_POINT('Ctrl Pts',(-3.62131121006315,-22.83696757079,-0.667927477355911));
#79087=CARTESIAN_POINT('Ctrl Pts',(-3.62134559074755,-22.8320694821121,
-0.659693071002674));
#79088=CARTESIAN_POINT('Ctrl Pts',(-3.62136278108975,-22.8296204377731,
-0.655575867826055));
#79089=CARTESIAN_POINT('Ctrl Pts',(-3.62137808417274,-22.8270381252706,
-0.65145909978056));
#79090=CARTESIAN_POINT('Ctrl Pts',(-3.62138921781553,-22.8243176686862,
-0.647353446733183));
#79091=CARTESIAN_POINT('Ctrl Pts',(-3.62139478463693,-22.8229574403939,
-0.645300620209494));
#79092=CARTESIAN_POINT('Ctrl Pts',(-3.62139930863626,-22.821765563472,-0.643549012983476));
#79093=CARTESIAN_POINT('Ctrl Pts',(-3.62140244291738,-22.8204425274908,
-0.641648678376371));
#79094=CARTESIAN_POINT('Ctrl Pts',(-3.62140533511476,-22.8192216793752,
-0.639895120682618));
#79095=CARTESIAN_POINT('Ctrl Pts',(-3.62140704397987,-22.8178893909459,
-0.638014546259289));
#79096=CARTESIAN_POINT('Ctrl Pts',(-3.62140729694812,-22.8161762062179,
-0.635677857882931));
#79097=CARTESIAN_POINT('Ctrl Pts',(-3.62140731812216,-22.816032808617,-0.635482271556591));
#79098=CARTESIAN_POINT('Ctrl Pts',(-3.62140732909606,-22.8158867177009,
-0.635283508571965));
#79099=CARTESIAN_POINT('Ctrl Pts',(-3.62140732970999,-22.8157377607153,
-0.635081387393934));
#79100=CARTESIAN_POINT('Ctrl Pts',(-3.62140735533527,-22.8095203002477,
-0.626644854999134));
#79101=CARTESIAN_POINT('Ctrl Pts',(-3.62142235572899,-22.803325198848,-0.619159888756903));
#79102=CARTESIAN_POINT('Ctrl Pts',(-3.62143959581722,-22.7973595082029,
-0.612522322813618));
#79103=CARTESIAN_POINT('Ctrl Pts',(-3.62145759034423,-22.7911327546029,
-0.605594292164457));
#79104=CARTESIAN_POINT('Ctrl Pts',(-3.62147802487608,-22.7851558742559,
-0.599588282153463));
#79105=CARTESIAN_POINT('Ctrl Pts',(-3.62148641822033,-22.7796081474466,
-0.594378218753685));
#79106=CARTESIAN_POINT('Ctrl Pts',(-3.62148993808707,-22.7772816303239,
-0.592193305522268));
#79107=CARTESIAN_POINT('Ctrl Pts',(-3.62149134031594,-22.7750299356726,
-0.590148386434912));
#79108=CARTESIAN_POINT('Ctrl Pts',(-3.62148955689063,-22.7728636189422,
-0.588234504651515));
#79109=CARTESIAN_POINT('Ctrl Pts',(-3.62148519496225,-22.7675652089869,
-0.58355350387633));
#79110=CARTESIAN_POINT('Ctrl Pts',(-3.62147007641132,-22.7627786705937,
-0.579652790409958));
#79111=CARTESIAN_POINT('Ctrl Pts',(-3.62145348161823,-22.7586166593081,
-0.576410055541454));
#79112=CARTESIAN_POINT('Ctrl Pts',(-3.62145084388833,-22.7579551107418,
-0.575894625270851));
#79113=CARTESIAN_POINT('Ctrl Pts',(-3.62144816886139,-22.7573092469938,
-0.57539587012562));
#79114=CARTESIAN_POINT('Ctrl Pts',(-3.62144549380582,-22.7566794179112,
-0.574913360807467));
#79115=CARTESIAN_POINT('Ctrl Pts',(-3.62143574146768,-22.7543832763796,
-0.573154296776697));
#79116=CARTESIAN_POINT('Ctrl Pts',(-3.62142616868904,-22.7523005262405,
-0.571610833801016));
#79117=CARTESIAN_POINT('Ctrl Pts',(-3.62141906430083,-22.7504451611699,
-0.570264303313079));
#79118=CARTESIAN_POINT('Ctrl Pts',(-3.62141551210673,-22.7495174786345,
-0.56959103806911));
#79119=CARTESIAN_POINT('Ctrl Pts',(-3.62141257701023,-22.7486465927841,
-0.568967075004624));
#79120=CARTESIAN_POINT('Ctrl Pts',(-3.62141053318238,-22.7478338505885,
-0.568390419400569));
#79121=CARTESIAN_POINT('Ctrl Pts',(-3.62140951126845,-22.7474274794907,
-0.568102091598542));
#79122=CARTESIAN_POINT('Ctrl Pts',(-3.62140871536219,-22.7473224594101,
-0.568028214121263));
#79123=CARTESIAN_POINT('Ctrl Pts',(-3.62140817245349,-22.7470892859499,
-0.567863836596028));
#79124=CARTESIAN_POINT('Ctrl Pts',(-3.6214076295448,-22.7468561124896,-0.567699459070793));
#79125=CARTESIAN_POINT('Ctrl Pts',(-3.62140733963366,-22.746495411902,-0.567443674678283));
#79126=CARTESIAN_POINT('Ctrl Pts',(-3.62140732970999,-22.7455712334679,
-0.56680067730871));
#79127=CARTESIAN_POINT('Ctrl Pts',(-3.6214072131747,-22.7347184538603,-0.559249853265867));
#79128=CARTESIAN_POINT('Ctrl Pts',(-3.62140718217023,-22.7238266504752,
-0.552735625785393));
#79129=CARTESIAN_POINT('Ctrl Pts',(-3.62140718961521,-22.713088824196,-0.54712899659101));
#79130=CARTESIAN_POINT('Ctrl Pts',(-3.62140719744237,-22.7017997952552,
-0.541234563435771));
#79131=CARTESIAN_POINT('Ctrl Pts',(-3.62140724776773,-22.6906810403832,
-0.536342399783166));
#79132=CARTESIAN_POINT('Ctrl Pts',(-3.62140728588091,-22.6799007092827,
-0.53228540519991));
#79133=CARTESIAN_POINT('Ctrl Pts',(-3.62140731030249,-22.6729930566932,
-0.529685827424681));
#79134=CARTESIAN_POINT('Ctrl Pts',(-3.62140732971,-22.6662231970864,-0.527428864804953));
#79135=CARTESIAN_POINT('Ctrl Pts',(-3.62140732971,-22.6596242971005,-0.525469586723355));
#79136=CARTESIAN_POINT('Origin',(0.,-21.6200560145,-0.216811574779));
#79137=CARTESIAN_POINT('',(-3.92508992147,-21.7707429986,-0.261552017256));
#79138=CARTESIAN_POINT('',(3.92508992519015,-21.7707429981472,-0.261552017112367));
#79139=CARTESIAN_POINT('',(-0.0354705937405,-21.7707429986,-0.261552017256));
#79140=CARTESIAN_POINT('Origin',(3.03257419176E-14,-21.0305048468,-0.0417680548823));
#79141=CARTESIAN_POINT('Origin',(-8.33777491493E-15,-21.0305048468,-0.0417680548823));
#79142=CARTESIAN_POINT('Origin',(-0.0354705937405,-21.8561316829,0.0260393118769));
#79143=CARTESIAN_POINT('Ctrl Pts',(4.05326999191,-21.5710708896125,-0.0674504957510902));
#79144=CARTESIAN_POINT('Ctrl Pts',(4.04568105172187,-21.5766811085323,-0.0845566755192819));
#79145=CARTESIAN_POINT('Ctrl Pts',(4.03782073411841,-21.5838132252431,-0.101090041800997));
#79146=CARTESIAN_POINT('Ctrl Pts',(4.02981682449863,-21.5923201463575,-0.116801414763259));
#79147=CARTESIAN_POINT('Ctrl Pts',(4.0217466234343,-21.6008975250503,-0.132642915333036));
#79148=CARTESIAN_POINT('Ctrl Pts',(4.01353044193539,-21.6108721210905,-0.147648314175529));
#79149=CARTESIAN_POINT('Ctrl Pts',(4.00529926687375,-21.6220544382609,-0.161598220461817));
#79150=CARTESIAN_POINT('Ctrl Pts',(4.00311074712359,-21.6250276130259,-0.165307246839182));
#79151=CARTESIAN_POINT('Ctrl Pts',(4.00092116743143,-21.6280859765477,-0.168941872280921));
#79152=CARTESIAN_POINT('Ctrl Pts',(3.99873298982911,-21.6312255779638,-0.172498452698097));
#79153=CARTESIAN_POINT('Ctrl Pts',(3.98987872328167,-21.64392969657,-0.18688983984035));
#79154=CARTESIAN_POINT('Ctrl Pts',(3.98105148723871,-21.6579637936179,-0.19999754833016));
#79155=CARTESIAN_POINT('Ctrl Pts',(3.97239798326953,-21.6730612515873,-0.211626876671228));
#79156=CARTESIAN_POINT('Ctrl Pts',(3.96363330690678,-21.688352668044,-0.223405608106326));
#79157=CARTESIAN_POINT('Ctrl Pts',(3.95504685519709,-21.7047345766709,-0.233667645129993));
#79158=CARTESIAN_POINT('Ctrl Pts',(3.94679105672644,-21.7219091373593,-0.242259604014651));
#79159=CARTESIAN_POINT('Ctrl Pts',(3.94578814651856,-21.7239954942746,-0.243303350819001));
#79160=CARTESIAN_POINT('Ctrl Pts',(3.94479011584885,-21.7260935274999,-0.244322511279171));
#79161=CARTESIAN_POINT('Ctrl Pts',(3.94379723797682,-21.7282026864134,-0.245316859709329));
#79162=CARTESIAN_POINT('Ctrl Pts',(3.9373235011442,-21.7419547702585,-0.251800184837398));
#79163=CARTESIAN_POINT('Ctrl Pts',(3.93106588671667,-21.7561829643929,-0.257229000399012));
#79164=CARTESIAN_POINT('Ctrl Pts',(3.92508992725,-21.7707429985995,-0.261552017257738));
#79165=CARTESIAN_POINT('',(-9.7699626167E-15,-21.5710708896,-0.0674504957552));
#79166=CARTESIAN_POINT('Ctrl Pts',(-3.92508992147,-21.7707429985995,-0.261552017257738));
#79167=CARTESIAN_POINT('Ctrl Pts',(-3.93309231670333,-21.7512455755997,
-0.255763041274999));
#79168=CARTESIAN_POINT('Ctrl Pts',(-3.94160650345342,-21.7323352144214,
-0.24798610008293));
#79169=CARTESIAN_POINT('Ctrl Pts',(-3.95046295408005,-21.7143708969331,
-0.238354106274979));
#79170=CARTESIAN_POINT('Ctrl Pts',(-3.95931940470668,-21.6964065794448,
-0.228722112467028));
#79171=CARTESIAN_POINT('Ctrl Pts',(-3.96851811920986,-21.6793884890492,
-0.217234920628154));
#79172=CARTESIAN_POINT('Ctrl Pts',(-3.97788956994937,-21.6636589267433,
-0.204078566910147));
#79173=CARTESIAN_POINT('Ctrl Pts',(-3.98619702881204,-21.6497152273721,
-0.192415925731835));
#79174=CARTESIAN_POINT('Ctrl Pts',(-3.99463812765578,-21.6367863343899,
-0.179442566946254));
#79175=CARTESIAN_POINT('Ctrl Pts',(-4.00307451569265,-21.6251068301091,
-0.165343857166143));
#79176=CARTESIAN_POINT('Ctrl Pts',(-4.01143033516254,-21.6135388665634,
-0.151379791837931));
#79177=CARTESIAN_POINT('Ctrl Pts',(-4.0197815333735,-21.6031970209888,-0.136312056895106));
#79178=CARTESIAN_POINT('Ctrl Pts',(-4.02799368560558,-21.5942795872117,
-0.12036246401268));
#79179=CARTESIAN_POINT('Ctrl Pts',(-4.02999966943303,-21.5921013241408,
-0.11646645423688));
#79180=CARTESIAN_POINT('Ctrl Pts',(-4.03199735667665,-21.590007894118,-0.11251801042259));
#79181=CARTESIAN_POINT('Ctrl Pts',(-4.03398478808377,-21.5880018653709,
-0.108520715440977));
#79182=CARTESIAN_POINT('Ctrl Pts',(-4.04055050501333,-21.5813747099083,
-0.0953151742387814));
#79183=CARTESIAN_POINT('Ctrl Pts',(-4.04700277586667,-21.5757039879415,
-0.0815773264565373));
#79184=CARTESIAN_POINT('Ctrl Pts',(-4.0532699684,-21.5710708896125,-0.0674504957510902));
#79185=CARTESIAN_POINT('Origin',(0.,-19.3367276644,6.74530982971));
#79186=CARTESIAN_POINT('Origin',(3.62140732971,-22.5742356128,-0.813060915858));
#79187=CARTESIAN_POINT('',(3.88319581089567,-22.6692776296171,-0.924567893965636));
#79188=CARTESIAN_POINT('Origin',(3.62140732971,-22.5742356128,-0.813060915858));
#79189=CARTESIAN_POINT('Origin',(3.62140732971,-22.5742356128,-0.813060915858));
#79190=CARTESIAN_POINT('Origin',(-8.43769498715E-15,-20.9451161625,-0.329359384015));
#79191=CARTESIAN_POINT('',(4.20883143442254,-21.7161399162306,-0.641571696058489));
#79192=CARTESIAN_POINT('Origin',(3.92508988180106,-21.6853545076789,-0.549143403786509));
#79193=CARTESIAN_POINT('Origin',(-5.90154768276285E-6,-20.922394848479,
-0.405877494386963));
#79194=CARTESIAN_POINT('Ctrl Pts',(4.05326999191,-21.5710708896,-0.0674504957552));
#79195=CARTESIAN_POINT('Ctrl Pts',(4.14906267383,-21.5773629037,-0.0866355443942));
#79196=CARTESIAN_POINT('Ctrl Pts',(4.24485535575,-21.5457105806,-0.118264986841));
#79197=CARTESIAN_POINT('Ctrl Pts',(4.31892160248,-21.4741377387,-0.1581676115));
#79198=CARTESIAN_POINT('Ctrl Pts',(4.35210058992,-21.3811601618,-0.196020670745));
#79199=CARTESIAN_POINT('Ctrl Pts',(4.34627746121,-21.2879273766,-0.225306031645));
#79200=CARTESIAN_POINT('Ctrl Pts',(4.02839229827,-21.5894620357,-0.123527140032));
#79201=CARTESIAN_POINT('Ctrl Pts',(4.12621567612,-21.6002038923,-0.14353500743));
#79202=CARTESIAN_POINT('Ctrl Pts',(4.22403905397,-21.5735624324,-0.184070478262));
#79203=CARTESIAN_POINT('Ctrl Pts',(4.29855068001,-21.5064409415,-0.240682386349));
#79204=CARTESIAN_POINT('Ctrl Pts',(4.32942721023,-21.4172157026,-0.298161067627));
#79205=CARTESIAN_POINT('Ctrl Pts',(4.31960138008,-21.3273686296,-0.345566786841));
#79206=CARTESIAN_POINT('Ctrl Pts',(4.00108772463,-21.6214549247,-0.174510108847));
#79207=CARTESIAN_POINT('Ctrl Pts',(4.10130096444,-21.6370719606,-0.193345500879));
#79208=CARTESIAN_POINT('Ctrl Pts',(4.20151420426,-21.6177474532,-0.241118366914));
#79209=CARTESIAN_POINT('Ctrl Pts',(4.27654207061,-21.5590494503,-0.313527678841));
#79210=CARTESIAN_POINT('Ctrl Pts',(4.30472756187,-21.4781622142,-0.390048280054));
#79211=CARTESIAN_POINT('Ctrl Pts',(4.29032296542,-21.3959792109,-0.454901796918));
#79212=CARTESIAN_POINT('Ctrl Pts',(3.97344013776,-21.6649708651,-0.215919998082));
#79213=CARTESIAN_POINT('Ctrl Pts',(4.07632718344,-21.6845855954,-0.231221519449));
#79214=CARTESIAN_POINT('Ctrl Pts',(4.17921422913,-21.6739877397,-0.283641075841));
#79215=CARTESIAN_POINT('Ctrl Pts',(4.2548069522,-21.6274322849,-0.369678608099));
#79216=CARTESIAN_POINT('Ctrl Pts',(4.28000984415,-21.5595261872,-0.463318063595));
#79217=CARTESIAN_POINT('Ctrl Pts',(4.26067677377,-21.4893040651,-0.543710875712));
#79218=CARTESIAN_POINT('Ctrl Pts',(3.94760066504,-21.7158967526,-0.245267576656));
#79219=CARTESIAN_POINT('Ctrl Pts',(4.05328834439,-21.7371001908,-0.255802966429));
#79220=CARTESIAN_POINT('Ctrl Pts',(4.15897602375,-21.7351383126,-0.310326311117));
#79221=CARTESIAN_POINT('Ctrl Pts',(4.23514222118,-21.7035971961,-0.40670982973));
#79222=CARTESIAN_POINT('Ctrl Pts',(4.25725324903,-21.6528882528,-0.513991630809));
#79223=CARTESIAN_POINT('Ctrl Pts',(4.2329693852,-21.5985179932,-0.606648702621));
#79224=CARTESIAN_POINT('Ctrl Pts',(3.92508992725,-21.7707430499,-0.261552067196));
#79225=CARTESIAN_POINT('Ctrl Pts',(4.03342463854,-21.7911739994,-0.267618198038));
#79226=CARTESIAN_POINT('Ctrl Pts',(4.14175934982,-21.7971474076,-0.32237766681));
#79227=CARTESIAN_POINT('Ctrl Pts',(4.21845509047,-21.7823880347,-0.42509762008));
#79228=CARTESIAN_POINT('Ctrl Pts',(4.23766397715,-21.7518700624,-0.541159533462));
#79229=CARTESIAN_POINT('Ctrl Pts',(4.20883136913,-21.7161396821,-0.641571966647));
#79230=CARTESIAN_POINT('Ctrl Pts',(4.34627740764205,-21.2879283386,-0.225306246837449));
#79231=CARTESIAN_POINT('Ctrl Pts',(4.33972068909289,-21.2976225055542,-0.254865144793904));
#79232=CARTESIAN_POINT('Ctrl Pts',(4.33297529253917,-21.3094345052532,-0.283628668746071));
#79233=CARTESIAN_POINT('Ctrl Pts',(4.3261130717861,-21.3232019719801,-0.311308815013811));
#79234=CARTESIAN_POINT('Ctrl Pts',(4.31906170088675,-21.3373489249461,-0.339751936403424));
#79235=CARTESIAN_POINT('Ctrl Pts',(4.31188705509232,-21.3535602107086,-0.36705104974735));
#79236=CARTESIAN_POINT('Ctrl Pts',(4.30466668690189,-21.3716230344419,-0.392936317507967));
#79237=CARTESIAN_POINT('Ctrl Pts',(4.29724098019976,-21.3901995429687,-0.419557730880084));
#79238=CARTESIAN_POINT('Ctrl Pts',(4.28976700965491,-21.4107338684777,-0.44468365175604));
#79239=CARTESIAN_POINT('Ctrl Pts',(4.28232735834422,-21.4329636594452,-0.468066387452847));
#79240=CARTESIAN_POINT('Ctrl Pts',(4.27459360193598,-21.4560722409054,-0.492373491977681));
#79241=CARTESIAN_POINT('Ctrl Pts',(4.26689705997568,-21.4810123362882,-0.514796688212307));
#79242=CARTESIAN_POINT('Ctrl Pts',(4.25932685806936,-21.5074654407041,-0.535108738097012));
#79243=CARTESIAN_POINT('Ctrl Pts',(4.2516335219164,-21.5343488220299,-0.555751176654447));
#79244=CARTESIAN_POINT('Ctrl Pts',(4.24407080218707,-21.5627939658263,-0.574213257646628));
#79245=CARTESIAN_POINT('Ctrl Pts',(4.23672655941918,-21.592454313204,-0.590309019639578));
#79246=CARTESIAN_POINT('Ctrl Pts',(4.22932882511418,-21.6223306906916,-0.60652201455594));
#79247=CARTESIAN_POINT('Ctrl Pts',(4.22215289497375,-21.6534390908336,-0.620334206824725));
#79248=CARTESIAN_POINT('Ctrl Pts',(4.21528083331161,-21.6854267960447,-0.631607268719839));
#79249=CARTESIAN_POINT('Ctrl Pts',(4.21309968663009,-21.6955794810031,-0.635185263614525));
#79250=CARTESIAN_POINT('Ctrl Pts',(4.21094908501466,-21.7058208153124,-0.638507851389803));
#79251=CARTESIAN_POINT('Ctrl Pts',(4.20883145763016,-21.7161397917727,-0.641571658435669));
#79252=CARTESIAN_POINT('Origin',(0.,-21.2594877202,0.729452270839));
#79253=CARTESIAN_POINT('',(-0.770172012660285,-22.6692778677973,-3.42046662122282));
#79254=CARTESIAN_POINT('',(-3.88319582787855,-22.6692776500678,-0.924567836647076));
#79255=CARTESIAN_POINT('Ctrl Pts',(-0.770171998117105,-22.6692781063945,
-3.42046654285371));
#79256=CARTESIAN_POINT('Ctrl Pts',(-0.827421116550194,-22.6692778637131,
-3.40984191914858));
#79257=CARTESIAN_POINT('Ctrl Pts',(-0.885473202714977,-22.6693131840285,
-3.39783479732127));
#79258=CARTESIAN_POINT('Ctrl Pts',(-0.944508027397569,-22.6693497782976,
-3.38426788045991));
#79259=CARTESIAN_POINT('Ctrl Pts',(-1.00214482600105,-22.669385505964,-3.37102224690357));
#79260=CARTESIAN_POINT('Ctrl Pts',(-1.06071870631787,-22.6694224477752,
-3.35628980600909));
#79261=CARTESIAN_POINT('Ctrl Pts',(-1.12037526257652,-22.6694287047423,
-3.33986282387073));
#79262=CARTESIAN_POINT('Ctrl Pts',(-1.1807553272836,-22.6694350375933,-3.32323661701836));
#79263=CARTESIAN_POINT('Ctrl Pts',(-1.24222354321397,-22.66941191933,-3.30487819993372));
#79264=CARTESIAN_POINT('Ctrl Pts',(-1.30479393660715,-22.6693729785012,
-3.28455273682354));
#79265=CARTESIAN_POINT('Ctrl Pts',(-1.33607913330373,-22.6693535080868,
-3.27439000526844));
#79266=CARTESIAN_POINT('Ctrl Pts',(-1.36763842454216,-22.66933084145,-3.2637351011711));
#79267=CARTESIAN_POINT('Ctrl Pts',(-1.39946526850315,-22.6693119348859,
-3.2525563464012));
#79268=CARTESIAN_POINT('Ctrl Pts',(-1.4167002163369,-22.6693016965587,-3.2465028006729));
#79269=CARTESIAN_POINT('Ctrl Pts',(-1.43345280452839,-22.6692925607939,
-3.24049710780066));
#79270=CARTESIAN_POINT('Ctrl Pts',(-1.45063396294028,-22.6692862684275,
-3.23421133216339));
#79271=CARTESIAN_POINT('Ctrl Pts',(-1.46518031847964,-22.669280941022,-3.22888950664568));
#79272=CARTESIAN_POINT('Ctrl Pts',(-1.48003370917092,-22.6692776518028,
-3.22336628878764));
#79273=CARTESIAN_POINT('Ctrl Pts',(-1.49573670679619,-22.669277457247,-3.21741542407968));
#79274=CARTESIAN_POINT('Ctrl Pts',(-1.55860736494078,-22.6692766782972,
-3.19358973234571));
#79275=CARTESIAN_POINT('Ctrl Pts',(-1.62324025161164,-22.6693594306987,
-3.16735192589975));
#79276=CARTESIAN_POINT('Ctrl Pts',(-1.68950078842028,-22.6694495359061,
-3.1383758418892));
#79277=CARTESIAN_POINT('Ctrl Pts',(-1.75397033305575,-22.6695372056108,
-3.11018296825049));
#79278=CARTESIAN_POINT('Ctrl Pts',(-1.8199809895668,-22.6696318336522,-3.07939755499398));
#79279=CARTESIAN_POINT('Ctrl Pts',(-1.88736401840794,-22.6696633157624,
-3.04569799944922));
#79280=CARTESIAN_POINT('Ctrl Pts',(-1.90163924554861,-22.6696699853094,
-3.03855868235092));
#79281=CARTESIAN_POINT('Ctrl Pts',(-1.91597589413568,-22.6696738209404,
-3.03128850615114));
#79282=CARTESIAN_POINT('Ctrl Pts',(-1.93037207366804,-22.6696741560997,
-3.02388430536752));
#79283=CARTESIAN_POINT('Ctrl Pts',(-1.99655808933587,-22.6696756969843,
-2.98984370814027));
#79284=CARTESIAN_POINT('Ctrl Pts',(-2.0639921443857,-22.6696207195799,-2.9529710534281));
#79285=CARTESIAN_POINT('Ctrl Pts',(-2.13240457787468,-22.6695411390171,
-2.91295064540045));
#79286=CARTESIAN_POINT('Ctrl Pts',(-2.14264786298145,-22.6695292235457,
-2.90695845321243));
#79287=CARTESIAN_POINT('Ctrl Pts',(-2.15291298661854,-22.6695167564933,
-2.90089569368716));
#79288=CARTESIAN_POINT('Ctrl Pts',(-2.16319894137902,-22.6695038449986,
-2.89476131015632));
#79289=CARTESIAN_POINT('Ctrl Pts',(-2.20269062567246,-22.66945427287,-2.87120908351563));
#79290=CARTESIAN_POINT('Ctrl Pts',(-2.24248921550098,-22.6693997396279,
-2.84660073830231));
#79291=CARTESIAN_POINT('Ctrl Pts',(-2.28253057469024,-22.6693557511123,
-2.82087535025402));
#79292=CARTESIAN_POINT('Ctrl Pts',(-2.30255125428487,-22.6693337568545,
-2.80801265622987));
#79293=CARTESIAN_POINT('Ctrl Pts',(-2.32263260683188,-22.6693143869059,
-2.79487067172989));
#79294=CARTESIAN_POINT('Ctrl Pts',(-2.34276574314777,-22.6693002735175,
-2.78144180749629));
#79295=CARTESIAN_POINT('Ctrl Pts',(-2.35283231130571,-22.6692932168234,
-2.77472737537949));
#79296=CARTESIAN_POINT('Ctrl Pts',(-2.36291182443243,-22.6692874736491,
-2.76794122175153));
#79297=CARTESIAN_POINT('Ctrl Pts',(-2.37300314129246,-22.6692833898957,
-2.76108239602025));
#79298=CARTESIAN_POINT('Ctrl Pts',(-2.38038679038729,-22.669280401881,-2.75606390704554));
#79299=CARTESIAN_POINT('Ctrl Pts',(-2.38857249092499,-22.6692782681744,
-2.75045999729516));
#79300=CARTESIAN_POINT('Ctrl Pts',(-2.39581236961099,-22.6692772028579,
-2.7454688367743));
#79301=CARTESIAN_POINT('Ctrl Pts',(-2.39846731513863,-22.6692768121942,
-2.74363852167134));
#79302=CARTESIAN_POINT('Ctrl Pts',(-2.40099538064462,-22.6692765652046,
-2.7418910615617));
#79303=CARTESIAN_POINT('Ctrl Pts',(-2.40331134426068,-22.6692764724457,
-2.74028694940537));
#79304=CARTESIAN_POINT('Ctrl Pts',(-2.46397465313337,-22.6692740427598,
-2.69826955736538));
#79305=CARTESIAN_POINT('Ctrl Pts',(-2.52566450010339,-22.6693011190506,
-2.65317766664651));
#79306=CARTESIAN_POINT('Ctrl Pts',(-2.58806079523629,-22.6693303276831,
-2.60473205212716));
#79307=CARTESIAN_POINT('Ctrl Pts',(-2.64885457236354,-22.6693587861532,
-2.55753066163419));
#79308=CARTESIAN_POINT('Ctrl Pts',(-2.71031901472123,-22.6693892685942,
-2.50714516049489));
#79309=CARTESIAN_POINT('Ctrl Pts',(-2.77210904370985,-22.6693964638087,
-2.45332459335306));
#79310=CARTESIAN_POINT('Ctrl Pts',(-2.79127659167261,-22.669398695797,-2.43662920869376));
#79311=CARTESIAN_POINT('Ctrl Pts',(-2.81047510471493,-22.6693986869654,
-2.41960335863671));
#79312=CARTESIAN_POINT('Ctrl Pts',(-2.82969328071026,-22.6693956817224,
-2.40223980577816));
#79313=CARTESIAN_POINT('Ctrl Pts',(-2.88915359094509,-22.6693863836141,
-2.34851762943846));
#79314=CARTESIAN_POINT('Ctrl Pts',(-2.94880203112499,-22.6693568467461,
-2.2915606455428));
#79315=CARTESIAN_POINT('Ctrl Pts',(-3.00826142484105,-22.6693210102179,
-2.23116139277267));
#79316=CARTESIAN_POINT('Ctrl Pts',(-3.02117978164482,-22.6693132242478,
-2.21803883888839));
#79317=CARTESIAN_POINT('Ctrl Pts',(-3.03408903777896,-22.6693051409203,
-2.20475387938249));
#79318=CARTESIAN_POINT('Ctrl Pts',(-3.04698502834267,-22.6692969032137,
-2.19130453156101));
#79319=CARTESIAN_POINT('Ctrl Pts',(-3.08311124787292,-22.6692738264912,
-2.15362816311631));
#79320=CARTESIAN_POINT('Ctrl Pts',(-3.11913371676518,-22.6692501395918,
-2.11466130127486));
#79321=CARTESIAN_POINT('Ctrl Pts',(-3.15495571344203,-22.6692321258323,
-2.07436211765109));
#79322=CARTESIAN_POINT('Ctrl Pts',(-3.17286671178045,-22.6692231189525,
-2.05421252583921));
#79323=CARTESIAN_POINT('Ctrl Pts',(-3.19072756673692,-22.669215519106,-2.03372983133757));
#79324=CARTESIAN_POINT('Ctrl Pts',(-3.20852543408119,-22.6692103105793,
-2.01290924567968));
#79325=CARTESIAN_POINT('Ctrl Pts',(-3.21742436775332,-22.669207706316,-2.00249895285073));
#79326=CARTESIAN_POINT('Ctrl Pts',(-3.22630755326258,-22.6692056993086,
-1.99200418606258));
#79327=CARTESIAN_POINT('Ctrl Pts',(-3.23517335911292,-22.6692044130975,
-1.98142435854934));
#79328=CARTESIAN_POINT('Ctrl Pts',(-3.23960626203808,-22.6692037699919,
-1.97613444479272));
#79329=CARTESIAN_POINT('Ctrl Pts',(-3.24403481995821,-22.6692033070462,
-1.97082326577994));
#79330=CARTESIAN_POINT('Ctrl Pts',(-3.2484588262394,-22.6692030402757,-1.9654907498876));
#79331=CARTESIAN_POINT('Ctrl Pts',(-3.25249029555434,-22.6692027971755,
-1.9606313819697));
#79332=CARTESIAN_POINT('Ctrl Pts',(-3.25722491356279,-22.6692027395928,
-1.95489491403983));
#79333=CARTESIAN_POINT('Ctrl Pts',(-3.26072982709033,-22.6692028178804,
-1.95063061071083));
#79334=CARTESIAN_POINT('Ctrl Pts',(-3.26107109426008,-22.6692028255031,
-1.95021540311252));
#79335=CARTESIAN_POINT('Ctrl Pts',(-3.26140073474145,-22.669202834414,-1.94981417846874));
#79336=CARTESIAN_POINT('Ctrl Pts',(-3.2617169825235,-22.6692028445671,-1.94942912033732));
#79337=CARTESIAN_POINT('Ctrl Pts',(-3.31475501068454,-22.6692045473556,
-1.88485088397679));
#79338=CARTESIAN_POINT('Ctrl Pts',(-3.36728482418238,-22.6692094999319,
-1.8169814029747));
#79339=CARTESIAN_POINT('Ctrl Pts',(-3.41889782933495,-22.6692160992244,
-1.74568479034844));
#79340=CARTESIAN_POINT('Ctrl Pts',(-3.46899241050097,-22.6692225043696,
-1.67648568176115));
#79341=CARTESIAN_POINT('Ctrl Pts',(-3.51822313576445,-22.6692304607544,
-1.60405778105421));
#79342=CARTESIAN_POINT('Ctrl Pts',(-3.56617794568295,-22.6692385027401,
-1.52830714221755));
#79343=CARTESIAN_POINT('Ctrl Pts',(-3.61332783129169,-22.6692464097407,
-1.45382798231662));
#79344=CARTESIAN_POINT('Ctrl Pts',(-3.65924411183341,-22.6692543994925,
-1.37613630659395));
#79345=CARTESIAN_POINT('Ctrl Pts',(-3.70349988977995,-22.6692610790745,
-1.29517797657114));
#79346=CARTESIAN_POINT('Ctrl Pts',(-3.74668697832313,-22.6692675973577,
-1.21617462990695));
#79347=CARTESIAN_POINT('Ctrl Pts',(-3.78829254637394,-22.6692728679912,
-1.13406018429735));
#79348=CARTESIAN_POINT('Ctrl Pts',(-3.82788909455231,-22.6692755966254,
-1.04882307993202));
#79349=CARTESIAN_POINT('Ctrl Pts',(-3.84679962356306,-22.6692768997671,
-1.00811552311086));
#79350=CARTESIAN_POINT('Ctrl Pts',(-3.86525149387254,-22.6692776231228,
-0.966696345601946));
#79351=CARTESIAN_POINT('Ctrl Pts',(-3.88319583536254,-22.669277625697,-0.924567839834829));
#79352=CARTESIAN_POINT('',(-4.20883136514917,-21.7161398144877,-0.641571946513287));
#79353=CARTESIAN_POINT('Origin',(3.73454221824776E-6,-20.9223934778998,
-0.405886279792362));
#79354=CARTESIAN_POINT('Ctrl Pts',(-4.20883136830913,-21.7161398184096,
-0.64157193548822));
#79355=CARTESIAN_POINT('Ctrl Pts',(-4.21550983438282,-21.6835963441684,
-0.63190945713986));
#79356=CARTESIAN_POINT('Ctrl Pts',(-4.22251793270132,-21.6518194483258,
-0.619667932074284));
#79357=CARTESIAN_POINT('Ctrl Pts',(-4.22977564768318,-21.6211630765059,
-0.604970177269395));
#79358=CARTESIAN_POINT('Ctrl Pts',(-4.23697770143729,-21.5907418160534,
-0.59038514321472));
#79359=CARTESIAN_POINT('Ctrl Pts',(-4.24442542990854,-21.5614248621562,
-0.573381306580857));
#79360=CARTESIAN_POINT('Ctrl Pts',(-4.25203271689245,-21.5335621959175,
-0.554128793480935));
#79361=CARTESIAN_POINT('Ctrl Pts',(-4.2597570299117,-21.5052709067846,-0.534580111026121));
#79362=CARTESIAN_POINT('Ctrl Pts',(-4.26764574195468,-21.4784799550627,
-0.512712720685886));
#79363=CARTESIAN_POINT('Ctrl Pts',(-4.27560222375549,-21.4535458981271,
-0.488760025977522));
#79364=CARTESIAN_POINT('Ctrl Pts',(-4.28299622290362,-21.4303745517511,
-0.466500664528232));
#79365=CARTESIAN_POINT('Ctrl Pts',(-4.29044860517308,-21.4088073429688,
-0.442440851489234));
#79366=CARTESIAN_POINT('Ctrl Pts',(-4.2978781876711,-21.3891119189423,-0.416813074488966));
#79367=CARTESIAN_POINT('Ctrl Pts',(-4.30513300329695,-21.3698797925041,
-0.391788142457173));
#79368=CARTESIAN_POINT('Ctrl Pts',(-4.31236599107304,-21.3524329342998,
-0.365268199171376));
#79369=CARTESIAN_POINT('Ctrl Pts',(-4.31949956336828,-21.3369948228324,
-0.337511485985271));
#79370=CARTESIAN_POINT('Ctrl Pts',(-4.32640210728653,-21.3220566911352,
-0.310653703675961));
#79371=CARTESIAN_POINT('Ctrl Pts',(-4.33321149785558,-21.3089996578518,
-0.282638077731985));
#79372=CARTESIAN_POINT('Ctrl Pts',(-4.33985671302662,-21.2979956656104,
-0.253736824411127));
#79373=CARTESIAN_POINT('Ctrl Pts',(-4.34201508527133,-21.2944215584035,
-0.244349669684097));
#79374=CARTESIAN_POINT('Ctrl Pts',(-4.34415613630056,-21.2910637697605,
-0.23486938707577));
#79375=CARTESIAN_POINT('Ctrl Pts',(-4.34627743422821,-21.2879273724791,
-0.225306183921295));
#79376=CARTESIAN_POINT('',(-3.90524240041216,-19.1260440734113,0.729452270839));
#79377=CARTESIAN_POINT('Origin',(0.,-21.2594877202,0.729452270839));
#79378=CARTESIAN_POINT('Origin',(4.36980373112E-13,-22.6692776292,0.729452270839));
#79379=CARTESIAN_POINT('',(3.02151310590175,-19.2807402146197,-1.87007015835883));
#79380=CARTESIAN_POINT('',(-3.0215131091296,-19.2807402513822,-1.87007018262017));
#79381=CARTESIAN_POINT('Origin',(-7.89278894574E-12,-21.9012363954,-0.65794048406));
#79382=CARTESIAN_POINT('',(3.69310715296,-19.4536303653,-0.974172913954));
#79383=CARTESIAN_POINT('Ctrl Pts',(3.69310715296,-19.4536303653,-0.974172913954));
#79384=CARTESIAN_POINT('Ctrl Pts',(3.69310715296,-19.5414102009,-1.06722029503));
#79385=CARTESIAN_POINT('Ctrl Pts',(3.66216118733,-19.6043893474,-1.18881869517));
#79386=CARTESIAN_POINT('Ctrl Pts',(3.60362130644,-19.6185190275,-1.30670041311));
#79387=CARTESIAN_POINT('Ctrl Pts',(3.4596034448,-19.6046311185,-1.53737756014));
#79388=CARTESIAN_POINT('Ctrl Pts',(3.29105041121,-19.5054576982,-1.70454430458));
#79389=CARTESIAN_POINT('Ctrl Pts',(3.20000833496,-19.4397458552,-1.77583596615));
#79390=CARTESIAN_POINT('Ctrl Pts',(3.10925931489,-19.3640825186,-1.83151964554));
#79391=CARTESIAN_POINT('Ctrl Pts',(3.02151310998,-19.2807402046,-1.87007014598));
#79392=CARTESIAN_POINT('',(3.69310716477216,-19.422499072587,-0.940557363267574));
#79393=CARTESIAN_POINT('Origin',(3.69310715296,-21.2594877202,0.729452270839));
#79394=CARTESIAN_POINT('Ctrl Pts',(3.64161488688817,-19.230640786913,-0.827763557767012));
#79395=CARTESIAN_POINT('Ctrl Pts',(3.65108695555808,-19.2513668038831,-0.832615986554939));
#79396=CARTESIAN_POINT('Ctrl Pts',(3.65983669873976,-19.2723722033248,-0.839085878865248));
#79397=CARTESIAN_POINT('Ctrl Pts',(3.66773155157564,-19.2935662778242,-0.847342030102235));
#79398=CARTESIAN_POINT('Ctrl Pts',(3.67975962178233,-19.3308348577536,-0.865342889941905));
#79399=CARTESIAN_POINT('Ctrl Pts',(3.68778346002,-19.3668639601,-0.889584895726));
#79400=CARTESIAN_POINT('Ctrl Pts',(3.69041389404,-19.382098195,-0.901291061203));
#79401=CARTESIAN_POINT('Ctrl Pts',(3.6923955115,-19.3993093787,-0.916416350024));
#79402=CARTESIAN_POINT('Ctrl Pts',(3.69301434458,-19.4154261934,-0.932955637331));
#79403=CARTESIAN_POINT('Ctrl Pts',(3.6930761889,-19.4178108664,-0.935459919036));
#79404=CARTESIAN_POINT('Ctrl Pts',(3.69310716781,-19.4201688307,-0.937994127672));
#79405=CARTESIAN_POINT('Ctrl Pts',(3.6931071763,-19.4224990853,-0.940557351746));
#79406=CARTESIAN_POINT('',(2.15473693583979,-17.5697153947013,-0.513604012327406));
#79407=CARTESIAN_POINT('Ctrl Pts',(2.15473698243741,-17.5697154200519,-0.5136040068197));
#79408=CARTESIAN_POINT('Ctrl Pts',(2.19493586295698,-17.591587578194,-0.508845790077125));
#79409=CARTESIAN_POINT('Ctrl Pts',(2.2348493286428,-17.6144272106717,-0.504900376847478));
#79410=CARTESIAN_POINT('Ctrl Pts',(2.2743994614938,-17.6382785139004,-0.501993185534341));
#79411=CARTESIAN_POINT('Ctrl Pts',(2.30940842753783,-17.6593911980977,-0.499419799438559));
#79412=CARTESIAN_POINT('Ctrl Pts',(2.34413402145529,-17.6812972807239,-0.497659044491585));
#79413=CARTESIAN_POINT('Ctrl Pts',(2.37850602772258,-17.7040298852337,-0.496901452718552));
#79414=CARTESIAN_POINT('Ctrl Pts',(2.38296457167826,-17.7069786312465,-0.496803182160986));
#79415=CARTESIAN_POINT('Ctrl Pts',(2.38741712730049,-17.7099412802568,-0.496721852194651));
#79416=CARTESIAN_POINT('Ctrl Pts',(2.391863502787,-17.7129178995795,-0.496657937294923));
#79417=CARTESIAN_POINT('Ctrl Pts',(2.42231996126403,-17.7333069294936,-0.496220137676885));
#79418=CARTESIAN_POINT('Ctrl Pts',(2.45248265130698,-17.7543477183242,-0.496596256764844));
#79419=CARTESIAN_POINT('Ctrl Pts',(2.48227924085577,-17.7760614635646,-0.49795944147974));
#79420=CARTESIAN_POINT('Ctrl Pts',(2.50998408353963,-17.7962508847392,-0.499226929425411));
#79421=CARTESIAN_POINT('Ctrl Pts',(2.53737267544625,-17.8170222467782,-0.501347616208947));
#79422=CARTESIAN_POINT('Ctrl Pts',(2.56435886864359,-17.8383863148398,-0.504496619865039));
#79423=CARTESIAN_POINT('Ctrl Pts',(2.57208046746885,-17.8444992467988,-0.50539764887472));
#79424=CARTESIAN_POINT('Ctrl Pts',(2.57976892295044,-17.8506606552126,-0.506383113442942));
#79425=CARTESIAN_POINT('Ctrl Pts',(2.58742171090786,-17.8568706632281,-0.507457736027369));
#79426=CARTESIAN_POINT('Ctrl Pts',(2.60478336360009,-17.8709591239276,-0.509895700360085));
#79427=CARTESIAN_POINT('Ctrl Pts',(2.62196092287367,-17.8852970680121,-0.51279187018127));
#79428=CARTESIAN_POINT('Ctrl Pts',(2.63891856064913,-17.8998831585272,-0.516206737313588));
#79429=CARTESIAN_POINT('',(2.1547368415,-17.3799083486,1.05880473119));
#79430=CARTESIAN_POINT('Origin',(2.15473684211,-21.2594877202,0.729452270839));
#79431=CARTESIAN_POINT('',(2.19100518433701,-17.3987921046005,1.04094167631916));
#79432=CARTESIAN_POINT('Origin',(3.61628644811E-15,-19.5917976147,-1.03352917222));
#79433=CARTESIAN_POINT('Ctrl Pts',(3.3084919335,-18.2908119326,0.937647357484));
#79434=CARTESIAN_POINT('Ctrl Pts',(3.28842087131374,-18.267491590574,0.92407553187254));
#79435=CARTESIAN_POINT('Ctrl Pts',(3.26766831975679,-18.2440984957641,0.912142274172242));
#79436=CARTESIAN_POINT('Ctrl Pts',(3.24638447088638,-18.2207666805675,0.901668540341281));
#79437=CARTESIAN_POINT('Ctrl Pts',(3.22582983381185,-18.1982342431039,0.891553649983741));
#79438=CARTESIAN_POINT('Ctrl Pts',(3.20477919355986,-18.1757584417377,0.882800213314553));
#79439=CARTESIAN_POINT('Ctrl Pts',(3.18333873530386,-18.1534303030335,0.875266901786711));
#79440=CARTESIAN_POINT('Ctrl Pts',(3.15921334934978,-18.1283060749298,0.86679021505029));
#79441=CARTESIAN_POINT('Ctrl Pts',(3.13459444825019,-18.1033687343773,0.859858392732952));
#79442=CARTESIAN_POINT('Ctrl Pts',(3.10959055101215,-18.078705314789,0.8542965648595));
#79443=CARTESIAN_POINT('Ctrl Pts',(3.08938102407995,-18.0587709806464,0.849801189233425));
#79444=CARTESIAN_POINT('Ctrl Pts',(3.06891911829239,-18.0390147346841,0.846201455913727));
#79445=CARTESIAN_POINT('Ctrl Pts',(3.04824722283645,-18.0194683464823,0.843418598582527));
#79446=CARTESIAN_POINT('Ctrl Pts',(3.01899893748294,-17.9918125206788,0.839481184836674));
#79447=CARTESIAN_POINT('Ctrl Pts',(2.9893358395126,-17.9645820394152,0.837178062763207));
#79448=CARTESIAN_POINT('Ctrl Pts',(2.95935194210494,-17.9378418981739,0.836320919939276));
#79449=CARTESIAN_POINT('Ctrl Pts',(2.94584902770437,-17.9257997732517,0.835934915210697));
#79450=CARTESIAN_POINT('Ctrl Pts',(2.93228061517327,-17.9138566853508,0.835842668757733));
#79451=CARTESIAN_POINT('Ctrl Pts',(2.91865355127057,-17.9020170167149,0.836029309984174));
#79452=CARTESIAN_POINT('Ctrl Pts',(2.88360609593356,-17.871566564535,0.836509332687114));
#79453=CARTESIAN_POINT('Ctrl Pts',(2.84817892182265,-17.841806783168,0.838830763975885));
#79454=CARTESIAN_POINT('Ctrl Pts',(2.81246376430789,-17.8127931084377,0.842778052462115));
#79455=CARTESIAN_POINT('Ctrl Pts',(2.80346044077422,-17.8054791409607,0.843773112201319));
#79456=CARTESIAN_POINT('Ctrl Pts',(2.79443876466176,-17.7982125836861,0.844871750865417));
#79457=CARTESIAN_POINT('Ctrl Pts',(2.78540017354257,-17.7909943955887,0.846071009554622));
#79458=CARTESIAN_POINT('Ctrl Pts',(2.74590734069087,-17.75945555372,0.851310999098805));
#79459=CARTESIAN_POINT('Ctrl Pts',(2.70609545059395,-17.7288430232367,0.858467094085384));
#79460=CARTESIAN_POINT('Ctrl Pts',(2.66605514085442,-17.699203858655,0.867328013205092));
#79461=CARTESIAN_POINT('Ctrl Pts',(2.62526986382453,-17.6690132445897,0.876353793559632));
#79462=CARTESIAN_POINT('Ctrl Pts',(2.58424717397413,-17.6398322788716,0.887148373721119));
#79463=CARTESIAN_POINT('Ctrl Pts',(2.54306973129522,-17.6117030744451,0.899540127854758));
#79464=CARTESIAN_POINT('Ctrl Pts',(2.53280236413254,-17.6046892131887,0.902629943083738));
#79465=CARTESIAN_POINT('Ctrl Pts',(2.52252533030265,-17.5977407178926,0.905819307788507));
#79466=CARTESIAN_POINT('Ctrl Pts',(2.51223983513437,-17.590858201157,0.909106054093216));
#79467=CARTESIAN_POINT('Ctrl Pts',(2.47043606656942,-17.5628853002849,0.922464514683179));
#79468=CARTESIAN_POINT('Ctrl Pts',(2.42849188551327,-17.5360017282731,0.937427721947892));
#79469=CARTESIAN_POINT('Ctrl Pts',(2.38648356239168,-17.5102466215557,0.953884379719845));
#79470=CARTESIAN_POINT('Ctrl Pts',(2.36426604216151,-17.4966251636635,0.96258803889498));
#79471=CARTESIAN_POINT('Ctrl Pts',(2.34203054572053,-17.4833193629859,0.971710330389014));
#79472=CARTESIAN_POINT('Ctrl Pts',(2.31978854938119,-17.4703353212206,0.981240656882616));
#79473=CARTESIAN_POINT('Ctrl Pts',(2.27685569545361,-17.4452727342119,0.999636672644391));
#79474=CARTESIAN_POINT('Ctrl Pts',(2.23389755795098,-17.4214081160994,1.01954811987916));
#79475=CARTESIAN_POINT('Ctrl Pts',(2.19100518797971,-17.3987921063194,1.04094168467634));
#79476=CARTESIAN_POINT('',(3.69310715317639,-18.8681377509785,1.396464174652));
#79477=CARTESIAN_POINT('Ctrl Pts',(3.69310715296,-18.8681377502,1.39646417295));
#79478=CARTESIAN_POINT('Ctrl Pts',(3.69310715214544,-18.8646906714413,1.38410581980008));
#79479=CARTESIAN_POINT('Ctrl Pts',(3.69259177657766,-18.8606009274501,1.37192583995273));
#79480=CARTESIAN_POINT('Ctrl Pts',(3.69158230972186,-18.8559385497586,1.36006768999457));
#79481=CARTESIAN_POINT('Ctrl Pts',(3.69051045782158,-18.8509880371591,1.34747670645363));
#79482=CARTESIAN_POINT('Ctrl Pts',(3.68888179706811,-18.8453922761963,1.33524861672336));
#79483=CARTESIAN_POINT('Ctrl Pts',(3.68674368558374,-18.8392502571381,1.3234995562242));
#79484=CARTESIAN_POINT('Ctrl Pts',(3.68471107890988,-18.8334113151466,1.31233025146306));
#79485=CARTESIAN_POINT('Ctrl Pts',(3.6822185871438,-18.8270791977462,1.30159301515885));
#79486=CARTESIAN_POINT('Ctrl Pts',(3.67931974328277,-18.8203454871076,1.2913464747379));
#79487=CARTESIAN_POINT('Ctrl Pts',(3.67582593698265,-18.8122297410447,1.27899692119402));
#79488=CARTESIAN_POINT('Ctrl Pts',(3.67174917848949,-18.8035434413388,1.26736803909472));
#79489=CARTESIAN_POINT('Ctrl Pts',(3.66718993232582,-18.7944372259978,1.25649703253233));
#79490=CARTESIAN_POINT('Ctrl Pts',(3.66234651516983,-18.7847634338783,1.24494845239495));
#79491=CARTESIAN_POINT('Ctrl Pts',(3.65695962342466,-18.7746169626732,1.23425432847766));
#79492=CARTESIAN_POINT('Ctrl Pts',(3.65114867253215,-18.7641618421269,1.22440440488792));
#79493=CARTESIAN_POINT('Ctrl Pts',(3.64917857203113,-18.7606172177432,1.22106496186765));
#79494=CARTESIAN_POINT('Ctrl Pts',(3.64715964689312,-18.757036896294,1.2178221718728));
#79495=CARTESIAN_POINT('Ctrl Pts',(3.64509617810887,-18.7534264676304,1.21467461506629));
#79496=CARTESIAN_POINT('Ctrl Pts',(3.63944836659227,-18.7435445538637,1.20605960343313));
#79497=CARTESIAN_POINT('Ctrl Pts',(3.633460487968,-18.7334271310955,1.19815442516915));
#79498=CARTESIAN_POINT('Ctrl Pts',(3.62720830935474,-18.7231697043666,1.19091932962045));
#79499=CARTESIAN_POINT('Ctrl Pts',(3.62167996051964,-18.714099804638,1.18452185851114));
#79500=CARTESIAN_POINT('Ctrl Pts',(3.6159451061393,-18.7049204146876,1.17864749381264));
#79501=CARTESIAN_POINT('Ctrl Pts',(3.6100371140147,-18.6956695920241,1.17326377729281));
#79502=CARTESIAN_POINT('',(3.69310715887669,-18.9880798391386,1.73153298807645));
#79503=CARTESIAN_POINT('Origin',(3.69310715296,-21.2594877202,0.729452270839));
#79504=CARTESIAN_POINT('Ctrl Pts',(3.37113078856,-18.8600780815,2.3667703805));
#79505=CARTESIAN_POINT('Ctrl Pts',(3.38869201095644,-18.8750724420214,2.35258647558843));
#79506=CARTESIAN_POINT('Ctrl Pts',(3.40608515391958,-18.8895522416563,2.33732078134583));
#79507=CARTESIAN_POINT('Ctrl Pts',(3.42323107209452,-18.9033876245546,2.3209245028101));
#79508=CARTESIAN_POINT('Ctrl Pts',(3.43956662988178,-18.9165691115148,2.30530315475608));
#79509=CARTESIAN_POINT('Ctrl Pts',(3.45567875628968,-18.9291660813847,2.28865339509923));
#79510=CARTESIAN_POINT('Ctrl Pts',(3.47148097362641,-18.941031716602,2.27091454974452));
#79511=CARTESIAN_POINT('Ctrl Pts',(3.48145442077251,-18.9485206204168,2.25971881481643));
#79512=CARTESIAN_POINT('Ctrl Pts',(3.49130400916866,-18.9557174945842,2.24808899655903));
#79513=CARTESIAN_POINT('Ctrl Pts',(3.50100148868141,-18.9625766922123,2.23601134904976));
#79514=CARTESIAN_POINT('Ctrl Pts',(3.51433259176288,-18.9720060156272,2.21940823442436));
#79515=CARTESIAN_POINT('Ctrl Pts',(3.52737641560849,-18.9807981294339,2.20195966579905));
#79516=CARTESIAN_POINT('Ctrl Pts',(3.54003953644244,-18.9888089790747,2.18363951709586));
#79517=CARTESIAN_POINT('Ctrl Pts',(3.55176141000878,-18.9962243838457,2.16668110142319));
#79518=CARTESIAN_POINT('Ctrl Pts',(3.56315714645582,-19.0029702658348,2.14897543228294));
#79519=CARTESIAN_POINT('Ctrl Pts',(3.57412705154925,-19.0089055820898,2.13052377010484));
#79520=CARTESIAN_POINT('Ctrl Pts',(3.58434149779586,-19.0144321539542,2.1133428091144));
#79521=CARTESIAN_POINT('Ctrl Pts',(3.5941867472996,-19.0192558666883,2.09551485099505));
#79522=CARTESIAN_POINT('Ctrl Pts',(3.60355875961401,-19.0232399131184,2.07706497899717));
#79523=CARTESIAN_POINT('Ctrl Pts',(3.61170017077009,-19.0267008304716,2.0610376853197));
#79524=CARTESIAN_POINT('Ctrl Pts',(3.61948537973937,-19.0295289947164,2.04453960996809));
#79525=CARTESIAN_POINT('Ctrl Pts',(3.62683611450434,-19.0316290862057,2.02760646710804));
#79526=CARTESIAN_POINT('Ctrl Pts',(3.63154312600466,-19.0329738707896,2.01676340165577));
#79527=CARTESIAN_POINT('Ctrl Pts',(3.63607140171859,-19.0340197317384,2.00574295712455));
#79528=CARTESIAN_POINT('Ctrl Pts',(3.64039632492325,-19.0347403250418,1.99456470966233));
#79529=CARTESIAN_POINT('Ctrl Pts',(3.64746980999939,-19.0359188675816,1.97628249680911));
#79530=CARTESIAN_POINT('Ctrl Pts',(3.65400205458385,-19.0362261503123,1.95756779122123));
#79531=CARTESIAN_POINT('Ctrl Pts',(3.65987960155281,-19.0355527052212,1.93853802054784));
#79532=CARTESIAN_POINT('Ctrl Pts',(3.66321196102245,-19.0351708858774,1.9277488193992));
#79533=CARTESIAN_POINT('Ctrl Pts',(3.66633371725679,-19.0344740007227,1.91685925102004));
#79534=CARTESIAN_POINT('Ctrl Pts',(3.66922427296373,-19.0334452293648,1.90589752741063));
#79535=CARTESIAN_POINT('Ctrl Pts',(3.67389612842881,-19.0317824795068,1.88818066133241));
#79536=CARTESIAN_POINT('Ctrl Pts',(3.6779632719388,-19.0292505095148,1.87027265608766));
#79537=CARTESIAN_POINT('Ctrl Pts',(3.68134407166181,-19.0258010723225,1.85232717239278));
#79538=CARTESIAN_POINT('Ctrl Pts',(3.68472487138482,-19.0223516351301,1.83438168869789));
#79539=CARTESIAN_POINT('Ctrl Pts',(3.68741859100349,-19.0179838058214,1.81639899816153));
#79540=CARTESIAN_POINT('Ctrl Pts',(3.68936491766357,-19.0126923096433,1.79856209470954));
#79541=CARTESIAN_POINT('Ctrl Pts',(3.691175201474,-19.0077706744108,1.7819719414688));
#79542=CARTESIAN_POINT('Ctrl Pts',(3.692339054035,-19.002052117354,1.76551215189331));
#79543=CARTESIAN_POINT('Ctrl Pts',(3.6928332680798,-18.9955694742247,1.74933281835986));
#79544=CARTESIAN_POINT('Ctrl Pts',(3.69301576350472,-18.9931756678873,1.74335837392833));
#79545=CARTESIAN_POINT('Ctrl Pts',(3.69310717012609,-18.9906780722399,1.73742235791273));
#79546=CARTESIAN_POINT('Ctrl Pts',(3.69310716565,-18.9880798435563,1.73153298612752));
#79547=CARTESIAN_POINT('',(-3.69310712510398,-18.9880798224936,1.73153306834489));
#79548=CARTESIAN_POINT('Ctrl Pts',(-3.6931070974719,-18.9880797849051,1.73153308492801));
#79549=CARTESIAN_POINT('Ctrl Pts',(-3.69310712468246,-18.9952618512105,
1.74781251238661));
#79550=CARTESIAN_POINT('Ctrl Pts',(-3.69240312457171,-19.0016683605087,
1.76445127512417));
#79551=CARTESIAN_POINT('Ctrl Pts',(-3.69101646164415,-19.0072517991255,
1.78127248331884));
#79552=CARTESIAN_POINT('Ctrl Pts',(-3.68965395140338,-19.0127379862463,
1.79780070223347));
#79553=CARTESIAN_POINT('Ctrl Pts',(-3.68763275825615,-19.017430215499,1.81450532064328));
#79554=CARTESIAN_POINT('Ctrl Pts',(-3.68499110971516,-19.0213207375549,
1.83124459990243));
#79555=CARTESIAN_POINT('Ctrl Pts',(-3.68216847190293,-19.0254778139009,
1.8491307501049));
#79556=CARTESIAN_POINT('Ctrl Pts',(-3.67863801749283,-19.0287156564556,
1.86704641253439));
#79557=CARTESIAN_POINT('Ctrl Pts',(-3.67447191242615,-19.0310659770756,
1.88483002313483));
#79558=CARTESIAN_POINT('Ctrl Pts',(-3.67001185511461,-19.0335821317326,
1.90386841060097));
#79559=CARTESIAN_POINT('Ctrl Pts',(-3.66482382726056,-19.0350816807103,
1.92275500216907));
#79560=CARTESIAN_POINT('Ctrl Pts',(-3.65901330345387,-19.0356459181985,
1.94133377213654));
#79561=CARTESIAN_POINT('Ctrl Pts',(-3.65432965714411,-19.0361007289725,
1.95630942498522));
#79562=CARTESIAN_POINT('Ctrl Pts',(-3.64924205643322,-19.0359489177316,
1.97108592139919));
#79563=CARTESIAN_POINT('Ctrl Pts',(-3.64380874651171,-19.0352461876269,
1.98560194762267));
#79564=CARTESIAN_POINT('Ctrl Pts',(-3.636611460834,-19.0343153095082,2.00483073985879));
#79565=CARTESIAN_POINT('Ctrl Pts',(-3.62880017214108,-19.0324130278275,
2.02361561274625));
#79566=CARTESIAN_POINT('Ctrl Pts',(-3.62049718169822,-19.0296723870873,
2.04186416513173));
#79567=CARTESIAN_POINT('Ctrl Pts',(-3.61264412060128,-19.027080258465,2.05912384979597));
#79568=CARTESIAN_POINT('Ctrl Pts',(-3.60435188602754,-19.0237393408979,
2.07590422321751));
#79569=CARTESIAN_POINT('Ctrl Pts',(-3.59570735538278,-19.0197564272955,
2.09216768631108));
#79570=CARTESIAN_POINT('Ctrl Pts',(-3.58793996124586,-19.0161776488708,
2.10678094098853));
#79571=CARTESIAN_POINT('Ctrl Pts',(-3.57988831651865,-19.0120810419503,
2.12097740580257));
#79572=CARTESIAN_POINT('Ctrl Pts',(-3.57159642781692,-19.0075286801433,
2.13475630859865));
#79573=CARTESIAN_POINT('Ctrl Pts',(-3.56060098950043,-19.0014920321319,
2.15302778825944));
#79574=CARTESIAN_POINT('Ctrl Pts',(-3.5491896971999,-18.9946593716137,2.17055724509778));
#79575=CARTESIAN_POINT('Ctrl Pts',(-3.53746128646186,-18.987172096478,2.187346950558));
#79576=CARTESIAN_POINT('Ctrl Pts',(-3.52445129523402,-18.9788666759046,
2.2059712915394));
#79577=CARTESIAN_POINT('Ctrl Pts',(-3.5110510390571,-18.9697558575544,2.22368578081534));
#79578=CARTESIAN_POINT('Ctrl Pts',(-3.49735539490297,-18.9599880019219,
2.24052062372232));
#79579=CARTESIAN_POINT('Ctrl Pts',(-3.48177128506724,-18.9488732757123,
2.25967679030909));
#79580=CARTESIAN_POINT('Ctrl Pts',(-3.46580843265995,-18.9369119359418,
2.27769158122885));
#79581=CARTESIAN_POINT('Ctrl Pts',(-3.44957385322151,-18.9242777572026,
2.29462021847525));
#79582=CARTESIAN_POINT('Ctrl Pts',(-3.43869249211144,-18.9158095944324,
2.30596677757017));
#79583=CARTESIAN_POINT('Ctrl Pts',(-3.4276880862854,-18.9070380273395,2.31682600136214));
#79584=CARTESIAN_POINT('Ctrl Pts',(-3.41658548099764,-18.8980052477675,
2.32721594002643));
#79585=CARTESIAN_POINT('Ctrl Pts',(-3.40159501320036,-18.8858094083421,
2.34124418267092));
#79586=CARTESIAN_POINT('Ctrl Pts',(-3.38642762053579,-18.8731390420533,
2.35441545122519));
#79587=CARTESIAN_POINT('Ctrl Pts',(-3.37113079773101,-18.8600780989522,
2.36677042601625));
#79588=CARTESIAN_POINT('',(-3.69310717902964,-18.8681378087753,1.39646426604976));
#79589=CARTESIAN_POINT('Origin',(-3.69310715296,-21.2594877202,0.729452270839));
#79590=CARTESIAN_POINT('Ctrl Pts',(-3.6100371473659,-18.6956696732068,1.17326396103852));
#79591=CARTESIAN_POINT('Ctrl Pts',(-3.61657749559202,-18.705910653501,1.17922394382632));
#79592=CARTESIAN_POINT('Ctrl Pts',(-3.62290464780229,-18.7160628008001,
1.18578600728785));
#79593=CARTESIAN_POINT('Ctrl Pts',(-3.62897495461051,-18.7260771573293,
1.19299524943752));
#79594=CARTESIAN_POINT('Ctrl Pts',(-3.6355512914387,-18.7369263258697,1.20080546499171));
#79595=CARTESIAN_POINT('Ctrl Pts',(-3.64182562246628,-18.7476133476187,
1.20937651984719));
#79596=CARTESIAN_POINT('Ctrl Pts',(-3.64770746228359,-18.7580240682704,
1.21875450143649));
#79597=CARTESIAN_POINT('Ctrl Pts',(-3.65261309355745,-18.7667069223432,
1.22657602007674));
#79598=CARTESIAN_POINT('Ctrl Pts',(-3.65724475415457,-18.7751962949054,
1.23495899770559));
#79599=CARTESIAN_POINT('Ctrl Pts',(-3.66153876063084,-18.78340609774,1.24391468191898));
#79600=CARTESIAN_POINT('Ctrl Pts',(-3.66633688812616,-18.7925797403346,
1.25392177317539));
#79601=CARTESIAN_POINT('Ctrl Pts',(-3.67071998458647,-18.8014160030125,
1.26465261682475));
#79602=CARTESIAN_POINT('Ctrl Pts',(-3.67458836821826,-18.8097703758799,
1.2760889058583));
#79603=CARTESIAN_POINT('Ctrl Pts',(-3.67745768618513,-18.8159671118947,
1.2845716088996));
#79604=CARTESIAN_POINT('Ctrl Pts',(-3.6800436539183,-18.8218982880675,1.2934417126838));
#79605=CARTESIAN_POINT('Ctrl Pts',(-3.68230789365157,-18.8275029762944,
1.30267319568792));
#79606=CARTESIAN_POINT('Ctrl Pts',(-3.68499199445435,-18.8341469495223,
1.31361648520723));
#79607=CARTESIAN_POINT('Ctrl Pts',(-3.68722236982464,-18.8403304069624,
1.32506993521974));
#79608=CARTESIAN_POINT('Ctrl Pts',(-3.68894069456791,-18.8459471700852,
1.33694694132116));
#79609=CARTESIAN_POINT('Ctrl Pts',(-3.68931992656701,-18.8471867822806,
1.33956818086555));
#79610=CARTESIAN_POINT('Ctrl Pts',(-3.68967428152814,-18.84839882896,1.34220986509019));
#79611=CARTESIAN_POINT('Ctrl Pts',(-3.69000325102315,-18.8495822432019,
1.34487073876146));
#79612=CARTESIAN_POINT('Ctrl Pts',(-3.69147094096868,-18.8548620190185,
1.3567421663343));
#79613=CARTESIAN_POINT('Ctrl Pts',(-3.69243036931968,-18.8595676287777,
1.36899573143837));
#79614=CARTESIAN_POINT('Ctrl Pts',(-3.69285480927325,-18.8636259589294,
1.38150306134678));
#79615=CARTESIAN_POINT('Ctrl Pts',(-3.69302282682337,-18.8652324775522,
1.38645417613242));
#79616=CARTESIAN_POINT('Ctrl Pts',(-3.69310721706151,-18.8667377203947,
1.39144456789607));
#79617=CARTESIAN_POINT('Ctrl Pts',(-3.69310720833,-18.8681378362,1.39646425696));
#79618=CARTESIAN_POINT('',(-2.19100517774646,-17.3987921007756,1.04094166879275));
#79619=CARTESIAN_POINT('Ctrl Pts',(-2.19100517814,-17.398792101,1.04094166862));
#79620=CARTESIAN_POINT('Ctrl Pts',(-2.23340908046747,-17.4211505588617,
1.01979176987668));
#79621=CARTESIAN_POINT('Ctrl Pts',(-2.27587182040943,-17.4447260821378,
1.00009119561888));
#79622=CARTESIAN_POINT('Ctrl Pts',(-2.31831144523611,-17.4694731033439,
0.981872772926845));
#79623=CARTESIAN_POINT('Ctrl Pts',(-2.36028923173101,-17.4939508214391,
0.963852607546885));
#79624=CARTESIAN_POINT('Ctrl Pts',(-2.40224490185501,-17.5195750573229,
0.947282414042425));
#79625=CARTESIAN_POINT('Ctrl Pts',(-2.4441036705446,-17.5463069780681,0.932244093891202));
#79626=CARTESIAN_POINT('Ctrl Pts',(-2.4689116555243,-17.5621498972243,0.923331494880038));
#79627=CARTESIAN_POINT('Ctrl Pts',(-2.49368565427865,-17.5783819578072,
0.914957918947159));
#79628=CARTESIAN_POINT('Ctrl Pts',(-2.51840978812709,-17.5949951496287,
0.907149090937463));
#79629=CARTESIAN_POINT('Ctrl Pts',(-2.55914933281228,-17.62236977374,0.894281983050483));
#79630=CARTESIAN_POINT('Ctrl Pts',(-2.59975309442327,-17.6507789369978,
0.882945861082856));
#79631=CARTESIAN_POINT('Ctrl Pts',(-2.64014296081438,-17.6801826263446,
0.873295721186059));
#79632=CARTESIAN_POINT('Ctrl Pts',(-2.6795212705324,-17.708849905774,0.863887267243712));
#79633=CARTESIAN_POINT('Ctrl Pts',(-2.71869660392543,-17.7384627806698,
0.85608145628018));
#79634=CARTESIAN_POINT('Ctrl Pts',(-2.7575849771126,-17.7689766998058,0.85006896734053));
#79635=CARTESIAN_POINT('Ctrl Pts',(-2.7851804530791,-17.7906296015127,0.845802460916248));
#79636=CARTESIAN_POINT('Ctrl Pts',(-2.81263120385022,-17.812736071274,0.842439932418081));
#79637=CARTESIAN_POINT('Ctrl Pts',(-2.83990214642615,-17.8352767486052,
0.840064297938821));
#79638=CARTESIAN_POINT('Ctrl Pts',(-2.87328324226734,-17.8628677461742,
0.837156393966854));
#79639=CARTESIAN_POINT('Ctrl Pts',(-2.90639530240287,-17.891109212603,0.835726215071071));
#79640=CARTESIAN_POINT('Ctrl Pts',(-2.93914685009623,-17.9199408622635,
0.835961192073837));
#79641=CARTESIAN_POINT('Ctrl Pts',(-2.96947375622024,-17.9466380657312,
0.836178773409867));
#79642=CARTESIAN_POINT('Ctrl Pts',(-2.99949281327367,-17.9738427332933,
0.837824051866936));
#79643=CARTESIAN_POINT('Ctrl Pts',(-3.02911562216786,-18.0014956493843,
0.841081001191144));
#79644=CARTESIAN_POINT('Ctrl Pts',(-3.05593606414302,-18.0265325536872,
0.844029837700133));
#79645=CARTESIAN_POINT('Ctrl Pts',(-3.08242830728943,-18.0519338760314,
0.848299586612206));
#79646=CARTESIAN_POINT('Ctrl Pts',(-3.1085035339598,-18.0776339030635,0.854055690967447));
#79647=CARTESIAN_POINT('Ctrl Pts',(-3.13266890449484,-18.1014515551147,
0.859390194722339));
#79648=CARTESIAN_POINT('Ctrl Pts',(-3.15647636754392,-18.1255260738493,
0.866001401350056));
#79649=CARTESIAN_POINT('Ctrl Pts',(-3.17982784457826,-18.1497786992006,
0.874045427786549));
#79650=CARTESIAN_POINT('Ctrl Pts',(-3.18918972837626,-18.1595018640351,
0.877270373285958));
#79651=CARTESIAN_POINT('Ctrl Pts',(-3.19847797729243,-18.1692533183757,
0.880725897195602));
#79652=CARTESIAN_POINT('Ctrl Pts',(-3.20768476668501,-18.1790264993383,
0.884423229782778));
#79653=CARTESIAN_POINT('Ctrl Pts',(-3.22918262193891,-18.2018468790326,
0.893056502185938));
#79654=CARTESIAN_POINT('Ctrl Pts',(-3.25024132019591,-18.2247909364654,
0.903007502286362));
#79655=CARTESIAN_POINT('Ctrl Pts',(-3.27073539415306,-18.2477489410748,
0.914432724385656));
#79656=CARTESIAN_POINT('Ctrl Pts',(-3.28355491073038,-18.2621097031804,
0.921579464677882));
#79657=CARTESIAN_POINT('Ctrl Pts',(-3.2961529105563,-18.2764753126739,0.929303427275135));
#79658=CARTESIAN_POINT('Ctrl Pts',(-3.3084919913374,-18.2908119591701,0.937647026553946));
#79659=CARTESIAN_POINT('',(-2.15473684280641,-17.3799083491911,1.05880473008226));
#79660=CARTESIAN_POINT('Origin',(2.6645352591E-15,-19.5917976147,-1.03352917222));
#79661=CARTESIAN_POINT('',(-2.15473684927718,-17.5697153655739,-0.513604050767344));
#79662=CARTESIAN_POINT('Origin',(-2.15473684211,-21.2594877202,0.729452270839));
#79663=CARTESIAN_POINT('Ctrl Pts',(-2.63891667022851,-17.8998816183554,
-0.516206449710607));
#79664=CARTESIAN_POINT('Ctrl Pts',(-2.61310289645698,-17.8776779425526,
-0.511008230762591));
#79665=CARTESIAN_POINT('Ctrl Pts',(-2.58678584252352,-17.8560536455099,
-0.507010684885198));
#79666=CARTESIAN_POINT('Ctrl Pts',(-2.56007862673513,-17.8350057727795,
-0.504006626604018));
#79667=CARTESIAN_POINT('Ctrl Pts',(-2.54018464775287,-17.8193273905386,
-0.501768929017689));
#79668=CARTESIAN_POINT('Ctrl Pts',(-2.52007339480444,-17.8039686517226,
-0.500083506521339));
#79669=CARTESIAN_POINT('Ctrl Pts',(-2.49978049122198,-17.7889257868244,
-0.498879424947764));
#79670=CARTESIAN_POINT('Ctrl Pts',(-2.46921773238009,-17.7662700120947,
-0.497065980429606));
#79671=CARTESIAN_POINT('Ctrl Pts',(-2.43823442114583,-17.744323941143,-0.496342120194636));
#79672=CARTESIAN_POINT('Ctrl Pts',(-2.40693510521941,-17.7230793986878,
-0.496510632439663));
#79673=CARTESIAN_POINT('Ctrl Pts',(-2.38602396458181,-17.7088858739441,
-0.496623215834878));
#79674=CARTESIAN_POINT('Ctrl Pts',(-2.36497297898658,-17.6950065181827,
-0.497135038263675));
#79675=CARTESIAN_POINT('Ctrl Pts',(-2.34379920732961,-17.6814325355428,
-0.497997390597506));
#79676=CARTESIAN_POINT('Ctrl Pts',(-2.30607364552788,-17.6572476085834,
-0.499533854048225));
#79677=CARTESIAN_POINT('Ctrl Pts',(-2.26794946462982,-17.6340259944123,
-0.502181444449583));
#79678=CARTESIAN_POINT('Ctrl Pts',(-2.22952537353873,-17.6117366097388,
-0.505711726429428));
#79679=CARTESIAN_POINT('Ctrl Pts',(-2.2214515349402,-17.6070530664407,-0.506453524767481));
#79680=CARTESIAN_POINT('Ctrl Pts',(-2.21336435003307,-17.6024106613826,
-0.507234449505707));
#79681=CARTESIAN_POINT('Ctrl Pts',(-2.2052645934251,-17.5978090805389,-0.508052596842114));
#79682=CARTESIAN_POINT('Ctrl Pts',(-2.18847673544652,-17.5882716722659,
-0.509748319559959));
#79683=CARTESIAN_POINT('Ctrl Pts',(-2.17163270974699,-17.5789083811218,
-0.511604117245896));
#79684=CARTESIAN_POINT('Ctrl Pts',(-2.1547368444,-17.5697153922,-0.513604062953));
#79685=CARTESIAN_POINT('',(-3.69310715294,-19.4224990402,-0.940557353778));
#79686=CARTESIAN_POINT('Ctrl Pts',(-3.69310715294,-19.4224990402,-0.940557353778));
#79687=CARTESIAN_POINT('Ctrl Pts',(-3.69310715296,-19.4065320759,-0.922993902523));
#79688=CARTESIAN_POINT('Ctrl Pts',(-3.69165304038,-19.3892706346,-0.906800491528));
#79689=CARTESIAN_POINT('Ctrl Pts',(-3.6887805345,-19.3710481782,-0.89227543696));
#79690=CARTESIAN_POINT('Ctrl Pts',(-3.68066808926,-19.3340162227,-0.867105044941));
#79691=CARTESIAN_POINT('Ctrl Pts',(-3.66836754819,-19.2957464376,-0.84852225854));
#79692=CARTESIAN_POINT('Ctrl Pts',(-3.66145077635,-19.2768489319,-0.840929561713));
#79693=CARTESIAN_POINT('Ctrl Pts',(-3.65309699002,-19.2562736874,-0.834189818013));
#79694=CARTESIAN_POINT('Ctrl Pts',(-3.64401528261,-19.235933638,-0.82903655384));
#79695=CARTESIAN_POINT('Ctrl Pts',(-3.64322047583,-19.2341674975,-0.8286005087));
#79696=CARTESIAN_POINT('Ctrl Pts',(-3.64242036464,-19.2324033163,-0.828176257781));
#79697=CARTESIAN_POINT('Ctrl Pts',(-3.64161503967,-19.2306411737,-0.82776370433));
#79698=CARTESIAN_POINT('',(-3.69310715914368,-19.4536303579338,-0.974172892806444));
#79699=CARTESIAN_POINT('Origin',(-3.69310715296,-21.2594877202,0.729452270839));
#79700=CARTESIAN_POINT('Ctrl Pts',(-3.02151310328351,-19.2807402657353,
-1.87007020034346));
#79701=CARTESIAN_POINT('Ctrl Pts',(-3.09553406839226,-19.3510460935362,
-1.83754967268177));
#79702=CARTESIAN_POINT('Ctrl Pts',(-3.17165791739679,-19.4158556004616,
-1.79287227600525));
#79703=CARTESIAN_POINT('Ctrl Pts',(-3.24819012525093,-19.4734829893339,
-1.73672176875692));
#79704=CARTESIAN_POINT('Ctrl Pts',(-3.41578700005397,-19.5829245957743,
-1.58670170203268));
#79705=CARTESIAN_POINT('Ctrl Pts',(-3.56871476432,-19.6239406117,-1.37338573889));
#79706=CARTESIAN_POINT('Ctrl Pts',(-3.64775681814,-19.6269188806,-1.23837648486));
#79707=CARTESIAN_POINT('Ctrl Pts',(-3.69310705761,-19.5585539651,-1.08539296335));
#79708=CARTESIAN_POINT('Ctrl Pts',(-3.69310716493,-19.4536303642,-0.974172886895));
#79709=CARTESIAN_POINT('Origin',(-3.62140732971,-22.5742356128,-0.813060915858));
#79710=CARTESIAN_POINT('Origin',(-3.62140732971,-22.5742356128,-0.813060915858));
#79711=CARTESIAN_POINT('Origin',(-3.62140732971,-22.5742356128,-0.813060915858));
#79712=CARTESIAN_POINT('Origin',(3.06421554797E-14,-20.9451161625,-0.329359384015));
#79713=CARTESIAN_POINT('Origin',(-3.92508992491174,-21.6853542976041,-0.549143341414481));
#79714=CARTESIAN_POINT('Ctrl Pts',(-3.92508992147,-21.7707429986,-0.261552017256));
#79715=CARTESIAN_POINT('Ctrl Pts',(-4.03342461998,-21.7911739897,-0.267618178739));
#79716=CARTESIAN_POINT('Ctrl Pts',(-4.14175931848,-21.7971474542,-0.322377668836));
#79717=CARTESIAN_POINT('Ctrl Pts',(-4.21845505507,-21.7823881416,-0.425097625007));
#79718=CARTESIAN_POINT('Ctrl Pts',(-4.23766395197,-21.7518702125,-0.54115952752));
#79719=CARTESIAN_POINT('Ctrl Pts',(-4.20883136158,-21.7161398512,-0.641571945224));
#79720=CARTESIAN_POINT('Ctrl Pts',(-3.94759644554,-21.7159070143,-0.24527067605));
#79721=CARTESIAN_POINT('Ctrl Pts',(-4.05328464276,-21.7371102811,-0.255805200216));
#79722=CARTESIAN_POINT('Ctrl Pts',(-4.15897283998,-21.7351498417,-0.310328579867));
#79723=CARTESIAN_POINT('Ctrl Pts',(-4.23513914343,-21.7036118067,-0.406713304892));
#79724=CARTESIAN_POINT('Ctrl Pts',(-4.25724960966,-21.6529065911,-0.513996782083));
#79725=CARTESIAN_POINT('Ctrl Pts',(-4.23296486329,-21.5985397884,-0.606655333963));
#79726=CARTESIAN_POINT('Ctrl Pts',(-3.97344038914,-21.6649651461,-0.215923674571));
#79727=CARTESIAN_POINT('Ctrl Pts',(-4.07632734574,-21.6845810666,-0.231225393142));
#79728=CARTESIAN_POINT('Ctrl Pts',(-4.17921430233,-21.6739831683,-0.283645658503));
#79729=CARTESIAN_POINT('Ctrl Pts',(-4.25480701452,-21.6274260446,-0.369684305774));
#79730=CARTESIAN_POINT('Ctrl Pts',(-4.28000999959,-21.5595174516,-0.463325016282));
#79731=CARTESIAN_POINT('Ctrl Pts',(-4.26067703305,-21.4892929177,-0.543718994175));
#79732=CARTESIAN_POINT('Ctrl Pts',(-4.00108738171,-21.6214550864,-0.174510379657));
#79733=CARTESIAN_POINT('Ctrl Pts',(-4.10130066591,-21.6370722475,-0.193345955876));
#79734=CARTESIAN_POINT('Ctrl Pts',(-4.20151395011,-21.6177478772,-0.241119104285));
#79735=CARTESIAN_POINT('Ctrl Pts',(-4.27654182968,-21.5590499941,-0.31352875262));
#79736=CARTESIAN_POINT('Ctrl Pts',(-4.30472727966,-21.4781628509,-0.390049652199));
#79737=CARTESIAN_POINT('Ctrl Pts',(-4.2903226061,-21.3959799196,-0.454903382914));
#79738=CARTESIAN_POINT('Ctrl Pts',(-4.02839244452,-21.5894619149,-0.1235267805));
#79739=CARTESIAN_POINT('Ctrl Pts',(-4.1262158112,-21.6002037523,-0.143534649036));
#79740=CARTESIAN_POINT('Ctrl Pts',(-4.22403917788,-21.5735622712,-0.18407007299));
#79741=CARTESIAN_POINT('Ctrl Pts',(-4.2985508016,-21.5064407622,-0.240681885995));
#79742=CARTESIAN_POINT('Ctrl Pts',(-4.32942734489,-21.4172155069,-0.298160451165));
#79743=CARTESIAN_POINT('Ctrl Pts',(-4.31960153738,-21.3273684168,-0.345566059647));
#79744=CARTESIAN_POINT('Ctrl Pts',(-4.0532699684,-21.5710708632,-0.0674504949952));
#79745=CARTESIAN_POINT('Ctrl Pts',(-4.14906265325,-21.5773628865,-0.0866355663445));
#79746=CARTESIAN_POINT('Ctrl Pts',(-4.2448553381,-21.545710571,-0.11826504072));
#79747=CARTESIAN_POINT('Ctrl Pts',(-4.31892158577,-21.4741377326,-0.158167701262));
#79748=CARTESIAN_POINT('Ctrl Pts',(-4.35210057067,-21.3811601556,-0.196020790393));
#79749=CARTESIAN_POINT('Ctrl Pts',(-4.34627743719,-21.2879273681,-0.225306170569));
#79750=CARTESIAN_POINT('Origin',(4.36983782492E-13,-22.5742356128,0.729452270839));
#79751=CARTESIAN_POINT('Origin',(2.45,0.,0.));
#79752=CARTESIAN_POINT('',(2.45,-0.730765926094,-8.94930152316968E-17));
#79753=CARTESIAN_POINT('Origin',(2.45,0.,0.));
#79754=CARTESIAN_POINT('Origin',(0.,0.,0.));
#79755=CARTESIAN_POINT('',(4.,-0.730765926094,-8.94930152316968E-17));
#79756=CARTESIAN_POINT('',(0.,-0.730765926094,-8.94930152316968E-17));
#79757=CARTESIAN_POINT('Origin',(4.,0.,0.));
#79758=CARTESIAN_POINT('Origin',(4.,0.,0.));
#79759=CARTESIAN_POINT('',(4.,-6.41575007864,3.96554608849));
#79760=CARTESIAN_POINT('',(4.,-8.14391944342,-3.85542016568));
#79761=CARTESIAN_POINT('Origin',(4.,-9.17423561284,0.47366156039));
#79762=CARTESIAN_POINT('',(4.,2.8773238354,-3.85542016568));
#79763=CARTESIAN_POINT('',(4.,-3.42065492897,-3.85542016568));
#79764=CARTESIAN_POINT('',(4.,3.0773238354,-3.65542016568));
#79765=CARTESIAN_POINT('Origin',(4.,2.8773238354,-3.65542016568));
#79766=CARTESIAN_POINT('',(4.,3.0773238354,1.84387696505));
#79767=CARTESIAN_POINT('',(4.,3.0773238354,0.47366156039));
#79768=CARTESIAN_POINT('',(4.,2.8773238354,2.04387696505));
#79769=CARTESIAN_POINT('Origin',(4.,2.8773238354,1.84387696505));
#79770=CARTESIAN_POINT('',(4.,-2.12788809108,2.04387696505));
#79771=CARTESIAN_POINT('',(4.,-2.74845588872,2.04387696505));
#79772=CARTESIAN_POINT('',(4.,-2.69184369587,2.1725725316));
#79773=CARTESIAN_POINT('Origin',(4.,-2.12788809108,3.34387696505));
#79774=CARTESIAN_POINT('',(4.,-2.74845588872,2.19982997428));
#79775=CARTESIAN_POINT('Origin',(4.3,-2.74845588872,2.19982997428));
#79776=CARTESIAN_POINT('',(4.3,-2.56170009476,2.4428735547));
#79777=CARTESIAN_POINT('Origin',(4.3,-2.69184369587,2.1725725316));
#79778=CARTESIAN_POINT('',(4.3,-6.28560647753,4.2358471116));
#79779=CARTESIAN_POINT('',(4.3,-4.42365328615,3.33936033315));
#79780=CARTESIAN_POINT('Origin',(4.29787870950426,-6.41482982759964,3.96745737345475));
#79781=CARTESIAN_POINT('Origin',(4.3,-2.12788809108,3.34387696505));
#79782=CARTESIAN_POINT('',(4.3,-2.12788809108,2.34387696505));
#79783=CARTESIAN_POINT('Origin',(4.3,-2.12788809108,2.04387696505));
#79784=CARTESIAN_POINT('Origin',(4.3,-2.12788809108,3.34387696505));
#79785=CARTESIAN_POINT('Origin',(4.3,-2.74845588872,2.04387696505));
#79786=CARTESIAN_POINT('',(4.3,2.8773238354,2.34387696505));
#79787=CARTESIAN_POINT('Origin',(4.3,2.8773238354,2.04387696505));
#79788=CARTESIAN_POINT('',(4.3,0.374717872161,2.34387696505));
#79789=CARTESIAN_POINT('Ctrl Pts',(4.,3.0773238354,1.84387696505));
#79790=CARTESIAN_POINT('Ctrl Pts',(4.,3.0773238354,2.04387696505));
#79791=CARTESIAN_POINT('Ctrl Pts',(4.,2.8773238354,2.04387696505));
#79792=CARTESIAN_POINT('Ctrl Pts',(4.,3.3773238354,1.84387696505));
#79793=CARTESIAN_POINT('Ctrl Pts',(4.,3.3773238354,2.34387696505));
#79794=CARTESIAN_POINT('Ctrl Pts',(4.,2.8773238354,2.34387696505));
#79795=CARTESIAN_POINT('Ctrl Pts',(4.3,3.3773238354,1.84387696505));
#79796=CARTESIAN_POINT('Ctrl Pts',(4.3,3.3773238354,2.34387696505));
#79797=CARTESIAN_POINT('Ctrl Pts',(4.3,2.8773238354,2.34387696505));
#79798=CARTESIAN_POINT('',(4.3,3.3773238354,1.84387696505));
#79799=CARTESIAN_POINT('Origin',(4.3,3.0773238354,1.84387696505));
#79800=CARTESIAN_POINT('Origin',(4.3,2.8773238354,1.84387696505));
#79801=CARTESIAN_POINT('Origin',(4.3,3.0773238354,0.47366156039));
#79802=CARTESIAN_POINT('',(4.3,3.3773238354,-3.65542016568));
#79803=CARTESIAN_POINT('Origin',(4.3,3.0773238354,-3.65542016568));
#79804=CARTESIAN_POINT('',(4.3,3.3773238354,-0.905771600316));
#79805=CARTESIAN_POINT('Ctrl Pts',(4.,2.8773238354,-3.85542016568));
#79806=CARTESIAN_POINT('Ctrl Pts',(4.,3.0773238354,-3.85542016568));
#79807=CARTESIAN_POINT('Ctrl Pts',(4.,3.0773238354,-3.65542016568));
#79808=CARTESIAN_POINT('Ctrl Pts',(4.,2.8773238354,-4.15542016568));
#79809=CARTESIAN_POINT('Ctrl Pts',(4.,3.3773238354,-4.15542016568));
#79810=CARTESIAN_POINT('Ctrl Pts',(4.,3.3773238354,-3.65542016568));
#79811=CARTESIAN_POINT('Ctrl Pts',(4.3,2.8773238354,-4.15542016568));
#79812=CARTESIAN_POINT('Ctrl Pts',(4.3,3.3773238354,-4.15542016568));
#79813=CARTESIAN_POINT('Ctrl Pts',(4.3,3.3773238354,-3.65542016568));
#79814=CARTESIAN_POINT('',(4.3,2.8773238354,-4.15542016568));
#79815=CARTESIAN_POINT('Origin',(4.3,2.8773238354,-3.85542016568));
#79816=CARTESIAN_POINT('Origin',(4.3,2.8773238354,-3.65542016568));
#79817=CARTESIAN_POINT('Origin',(4.3,-3.42065492897,-3.85542016568));
#79818=CARTESIAN_POINT('',(4.3,-8.14391944342,-4.15542016568));
#79819=CARTESIAN_POINT('Origin',(4.3,-8.14391944342,-3.85542016568));
#79820=CARTESIAN_POINT('',(4.3,-2.63329780401,-4.15542016568));
#79821=CARTESIAN_POINT('Origin',(3.7,-9.17423561284,0.47366156039));
#79822=CARTESIAN_POINT('',(3.99616160125331,-8.70088467100253,-3.90297923453123));
#79823=CARTESIAN_POINT('Ctrl Pts',(4.,-8.14391944342,-3.85542016568));
#79824=CARTESIAN_POINT('Ctrl Pts',(4.,-8.22339027599,-3.86461668513));
#79825=CARTESIAN_POINT('Ctrl Pts',(3.99962763899,-8.3031200968,-3.87300735474));
#79826=CARTESIAN_POINT('Ctrl Pts',(3.99902875837,-8.38309753718,-3.88055924261));
#79827=CARTESIAN_POINT('Ctrl Pts',(3.99803977235,-8.49460012163,-3.88985328888));
#79828=CARTESIAN_POINT('Ctrl Pts',(3.99700563085,-8.6064155396,-3.89742302488));
#79829=CARTESIAN_POINT('Ctrl Pts',(3.99671653073,-8.63788417864,-3.89941416203));
#79830=CARTESIAN_POINT('Ctrl Pts',(3.99643383471,-8.66937471516,-3.90126651862));
#79831=CARTESIAN_POINT('Ctrl Pts',(3.99616160126,-8.700884671,-3.90297923457));
#79832=CARTESIAN_POINT('',(3.99951365737889,-8.00613533634358,4.74991748852224));
#79833=CARTESIAN_POINT('Ctrl Pts',(3.99951362599666,-8.00613533213075,4.74991748884671));
#79834=CARTESIAN_POINT('Ctrl Pts',(3.99912970651189,-7.93705421321271,4.72406529283756));
#79835=CARTESIAN_POINT('Ctrl Pts',(3.99857561954119,-7.86817196474413,4.69734499917644));
#79836=CARTESIAN_POINT('Ctrl Pts',(3.9980140143817,-7.79955119479,4.66974300961157));
#79837=CARTESIAN_POINT('Ctrl Pts',(3.99745667146121,-7.73145121442678,4.64235050223209));
#79838=CARTESIAN_POINT('Ctrl Pts',(3.99689185763882,-7.66360880560323,4.6140896699695));
#79839=CARTESIAN_POINT('Ctrl Pts',(3.99642772185445,-7.59608259133466,4.58495963619982));
#79840=CARTESIAN_POINT('Ctrl Pts',(3.99596348780259,-7.52854208031863,4.55582343497737));
#79841=CARTESIAN_POINT('Ctrl Pts',(3.99559997461198,-7.461317947509,4.52581768640237));
#79842=CARTESIAN_POINT('Ctrl Pts',(3.99539475488255,-7.39446554448369,4.49495354860779));
#79843=CARTESIAN_POINT('Ctrl Pts',(3.99518950133484,-7.32760212481346,4.46408432469467));
#79844=CARTESIAN_POINT('Ctrl Pts',(3.9951425932134,-7.26111060723937,4.43235645100427));
#79845=CARTESIAN_POINT('Ctrl Pts',(3.99526097596942,-7.1950423146551,4.39979279428734));
#79846=CARTESIAN_POINT('Ctrl Pts',(3.99538088048154,-7.12812474443087,4.36681054667843));
#79847=CARTESIAN_POINT('Ctrl Pts',(3.99567046299158,-7.06164141244719,4.33297088933084));
#79848=CARTESIAN_POINT('Ctrl Pts',(3.99608398850385,-6.99564062204421,4.29830946415507));
#79849=CARTESIAN_POINT('Ctrl Pts',(3.99649234912136,-6.93046417530672,4.26408095692022));
#79850=CARTESIAN_POINT('Ctrl Pts',(3.9970214669193,-6.86575833052573,4.22905112782395));
#79851=CARTESIAN_POINT('Ctrl Pts',(3.99757632607106,-6.80156401020727,4.19326539858406));
#79852=CARTESIAN_POINT('Ctrl Pts',(3.99814171190807,-6.73615180711144,4.15680074910478));
#79853=CARTESIAN_POINT('Ctrl Pts',(3.99873399116725,-6.67127079573283,4.11955123467727));
#79854=CARTESIAN_POINT('Ctrl Pts',(3.99919856363035,-6.6069575312888,4.08157632337734));
#79855=CARTESIAN_POINT('Ctrl Pts',(3.99966313609345,-6.54264426684478,4.04360141207741));
#79856=CARTESIAN_POINT('Ctrl Pts',(4.,-6.47889880397702,4.00490112886999));
#79857=CARTESIAN_POINT('Ctrl Pts',(4.,-6.41575007864,3.96554608849));
#79858=CARTESIAN_POINT('',(3.99944937669,-8.31076354672,4.82056300746));
#79859=CARTESIAN_POINT('Ctrl Pts',(3.99944937669,-8.31076354672,4.82056300746));
#79860=CARTESIAN_POINT('Ctrl Pts',(3.99959839809,-8.28592729564,4.81813395331));
#79861=CARTESIAN_POINT('Ctrl Pts',(3.99969341422,-8.26106714699,4.8150399126));
#79862=CARTESIAN_POINT('Ctrl Pts',(3.99975395169,-8.23622932864,4.81128563568));
#79863=CARTESIAN_POINT('Ctrl Pts',(3.99984876957,-8.17436353389,4.80027772376));
#79864=CARTESIAN_POINT('Ctrl Pts',(3.99983052524,-8.11319387748,4.78525185918));
#79865=CARTESIAN_POINT('Ctrl Pts',(3.99979379772,-8.07691196013,4.77482737361));
#79866=CARTESIAN_POINT('Ctrl Pts',(3.99970844997,-8.04117830882,4.76303153489));
#79867=CARTESIAN_POINT('Ctrl Pts',(3.99951367307,-8.00613533845,4.74991748836));
#79868=CARTESIAN_POINT('',(3.99616169506664,-8.70088460854749,4.85030293274176));
#79869=CARTESIAN_POINT('Ctrl Pts',(3.99616169511,-8.70088460852,4.850302933));
#79870=CARTESIAN_POINT('Ctrl Pts',(3.99683804383,-8.62256210931,4.84604483372));
#79871=CARTESIAN_POINT('Ctrl Pts',(3.99757933996,-8.54435185028,4.84092376899));
#79872=CARTESIAN_POINT('Ctrl Pts',(3.99832332564,-8.46629167717,4.83495432364));
#79873=CARTESIAN_POINT('Ctrl Pts',(3.99898336569,-8.38842527481,4.8281587616));
#79874=CARTESIAN_POINT('Ctrl Pts',(3.99944937669,-8.31076354672,4.82056300746));
#79875=CARTESIAN_POINT('',(3.7,-8.7279990537,4.59960059693));
#79876=CARTESIAN_POINT('Origin',(3.7,-8.69574098918,4.89786125018));
#79877=CARTESIAN_POINT('',(3.7,-8.7279990537,-3.65227747616));
#79878=CARTESIAN_POINT('Origin',(3.7,-9.17423561284,0.47366156039));
#79879=CARTESIAN_POINT('Origin',(3.7,-8.69574098918,-3.9505381294));
#79880=CARTESIAN_POINT('Origin',(0.,-2.35608968258,2.34387696505));
#79881=CARTESIAN_POINT('',(4.35,-2.56170009476,2.4428735547));
#79882=CARTESIAN_POINT('',(4.35,-7.88049121843,5.00374669681));
#79883=CARTESIAN_POINT('',(4.35,2.08731990915,0.204479493281));
#79884=CARTESIAN_POINT('',(4.2990272509,-7.88049121843,5.00374669681));
#79885=CARTESIAN_POINT('',(3.225,-7.88049121843,5.00374669681));
#79886=CARTESIAN_POINT('Ctrl Pts',(4.2990272509,-7.88049121843,5.00374669681));
#79887=CARTESIAN_POINT('Ctrl Pts',(4.29860194904898,-7.84336279989873,4.98587023435574));
#79888=CARTESIAN_POINT('Ctrl Pts',(4.29807036319667,-7.8063193049477,4.96803466061349));
#79889=CARTESIAN_POINT('Ctrl Pts',(4.29749123915026,-7.76934684031188,4.95023328629991));
#79890=CARTESIAN_POINT('Ctrl Pts',(4.29661357039136,-7.71331467008551,4.92325511090297));
#79891=CARTESIAN_POINT('Ctrl Pts',(4.29562842420427,-7.65745144851057,4.89635828031341));
#79892=CARTESIAN_POINT('Ctrl Pts',(4.29470009048654,-7.60171026056881,4.86952020595908));
#79893=CARTESIAN_POINT('Ctrl Pts',(4.29377028407366,-7.54588064561534,4.84263955607304));
#79894=CARTESIAN_POINT('Ctrl Pts',(4.29289746676361,-7.49017341724383,4.8158178323467));
#79895=CARTESIAN_POINT('Ctrl Pts',(4.29219442747521,-7.43454058879187,4.78903193034465));
#79896=CARTESIAN_POINT('Ctrl Pts',(4.29149095408814,-7.3788734092915,4.76222948911851));
#79897=CARTESIAN_POINT('Ctrl Pts',(4.29095746147181,-7.32328068911448,4.73546289822188));
#79898=CARTESIAN_POINT('Ctrl Pts',(4.29065473399492,-7.26771400724003,4.7087088442481));
#79899=CARTESIAN_POINT('Ctrl Pts',(4.29035187162506,-7.21212256529347,4.68194286888037));
#79900=CARTESIAN_POINT('Ctrl Pts',(4.29027997715909,-7.15655715410882,4.65518942682211));
#79901=CARTESIAN_POINT('Ctrl Pts',(4.29044774917812,-7.10096941674446,4.6284252355263));
#79902=CARTESIAN_POINT('Ctrl Pts',(4.29052775589753,-7.07446086941765,4.61566199195374));
#79903=CARTESIAN_POINT('Ctrl Pts',(4.29066150240974,-7.04794724961644,4.6028963061693));
#79904=CARTESIAN_POINT('Ctrl Pts',(4.29084575810665,-7.02142335390664,4.59012567283795));
#79905=CARTESIAN_POINT('Ctrl Pts',(4.29123152417027,-6.96589172578971,4.56338849709526));
#79906=CARTESIAN_POINT('Ctrl Pts',(4.29184075891047,-6.91031984610482,4.53663194126546));
#79907=CARTESIAN_POINT('Ctrl Pts',(4.29260245682323,-6.85466578564437,4.50983581716746));
#79908=CARTESIAN_POINT('Ctrl Pts',(4.29336407793749,-6.79901733652759,4.48304239479976));
#79909=CARTESIAN_POINT('Ctrl Pts',(4.29427813122767,-6.74328668363906,4.45620939309286));
#79910=CARTESIAN_POINT('Ctrl Pts',(4.29522152510374,-6.68743327543012,4.42931728747705));
#79911=CARTESIAN_POINT('Ctrl Pts',(4.29540155763234,-6.67677449274567,4.42418533369164));
#79912=CARTESIAN_POINT('Ctrl Pts',(4.29558250634003,-6.66611124458006,4.41905122987873));
#79913=CARTESIAN_POINT('Ctrl Pts',(4.29576330024143,-6.65544325666937,4.41391484398757));
#79914=CARTESIAN_POINT('Ctrl Pts',(4.29671133096125,-6.59950342584761,4.38698112788367));
#79915=CARTESIAN_POINT('Ctrl Pts',(4.29766075533132,-6.54342366948845,4.35998004088301));
#79916=CARTESIAN_POINT('Ctrl Pts',(4.29842842934662,-6.48716607127935,4.33289332720474));
#79917=CARTESIAN_POINT('Ctrl Pts',(4.29919717698267,-6.43082979472131,4.30576873174731));
#79918=CARTESIAN_POINT('Ctrl Pts',(4.29978365749905,-6.37431514200558,4.27855825235265));
#79919=CARTESIAN_POINT('Ctrl Pts',(4.29995176543971,-6.31758659819914,4.25124478941713));
#79920=CARTESIAN_POINT('Ctrl Pts',(4.29998333258852,-6.30693416633443,4.24611589339078));
#79921=CARTESIAN_POINT('Ctrl Pts',(4.3,-6.29627420060992,4.24098336998769));
#79922=CARTESIAN_POINT('Ctrl Pts',(4.3,-6.28560647753,4.2358471116));
#79923=CARTESIAN_POINT('',(4.225,-2.56170009476,2.4428735547));
#79924=CARTESIAN_POINT('Ctrl Pts',(4.2990272509,-7.88049121843,5.00374669681));
#79925=CARTESIAN_POINT('Ctrl Pts',(4.20814466399,-7.88133645067,5.00415365756));
#79926=CARTESIAN_POINT('Ctrl Pts',(4.11726207707,-7.8971129981,4.97354910689));
#79927=CARTESIAN_POINT('Ctrl Pts',(4.04405123536,-7.92782451085,4.91150498201));
#79928=CARTESIAN_POINT('Ctrl Pts',(4.00460089543,-7.96672185122,4.83165605064));
#79929=CARTESIAN_POINT('Ctrl Pts',(3.99951361632,-8.0061354071,4.74991733337));
#79930=CARTESIAN_POINT('Ctrl Pts',(4.29534152276,-7.55873090479,4.8488266546));
#79931=CARTESIAN_POINT('Ctrl Pts',(4.21089110293,-7.56075677108,4.84980205594));
#79932=CARTESIAN_POINT('Ctrl Pts',(4.12644068311,-7.57560508753,4.82414594128));
#79933=CARTESIAN_POINT('Ctrl Pts',(4.05583695285,-7.60300935451,4.77146524893));
#79934=CARTESIAN_POINT('Ctrl Pts',(4.01210473647,-7.6379921895,4.70122601239));
#79935=CARTESIAN_POINT('Ctrl Pts',(3.99767078695,-7.67454601586,4.62582683568));
#79936=CARTESIAN_POINT('Ctrl Pts',(4.28495419985,-7.24223776902,4.69644263496));
#79937=CARTESIAN_POINT('Ctrl Pts',(4.20364197507,-7.24265108624,4.69664162775));
#79938=CARTESIAN_POINT('Ctrl Pts',(4.12232975028,-7.25504442659,4.67195877864));
#79939=CARTESIAN_POINT('Ctrl Pts',(4.05372035815,-7.27955010958,4.62221233106));
#79940=CARTESIAN_POINT('Ctrl Pts',(4.00967965098,-7.31194178404,4.55622127864));
#79941=CARTESIAN_POINT('Ctrl Pts',(3.99247722227,-7.34677145748,4.48508959035));
#79942=CARTESIAN_POINT('Ctrl Pts',(4.28719359971,-6.92729615453,4.54480563642));
#79943=CARTESIAN_POINT('Ctrl Pts',(4.20516486744,-6.92619358841,4.54427477668));
#79944=CARTESIAN_POINT('Ctrl Pts',(4.12313613516,-6.93728087775,4.51842626492));
#79945=CARTESIAN_POINT('Ctrl Pts',(4.05411385932,-6.96067605503,4.46706057541));
#79946=CARTESIAN_POINT('Ctrl Pts',(4.01020087277,-6.99204699421,4.39931666036));
#79947=CARTESIAN_POINT('Ctrl Pts',(3.99359726714,-7.02607103842,4.32667666396));
#79948=CARTESIAN_POINT('Ctrl Pts',(4.3,-6.60947733541,4.39178333134));
#79949=CARTESIAN_POINT('Ctrl Pts',(4.21340350799,-6.60705721212,4.39061809876));
#79950=CARTESIAN_POINT('Ctrl Pts',(4.12680701597,-6.61808600203,4.3615202213));
#79951=CARTESIAN_POINT('Ctrl Pts',(4.0550389398,-6.64318599408,4.30449502667));
#79952=CARTESIAN_POINT('Ctrl Pts',(4.01201861445,-6.67775474512,4.23026617343));
#79953=CARTESIAN_POINT('Ctrl Pts',(4.,-6.71532134284,4.1522424388));
#79954=CARTESIAN_POINT('Ctrl Pts',(4.3,-6.28560647753,4.2358471116));
#79955=CARTESIAN_POINT('Ctrl Pts',(4.20575222039,-6.28560647753,4.2358471116));
#79956=CARTESIAN_POINT('Ctrl Pts',(4.11150444078,-6.30166230076,4.20250005951));
#79957=CARTESIAN_POINT('Ctrl Pts',(4.0370110165,-6.33397844241,4.13538123018));
#79958=CARTESIAN_POINT('Ctrl Pts',(4.,-6.37486426052,4.05046365934));
#79959=CARTESIAN_POINT('Ctrl Pts',(4.,-6.41575007864,3.96554608849));
#79960=CARTESIAN_POINT('Origin',(4.29708331441242,-8.00976085385706,4.7353069832235));
#79961=CARTESIAN_POINT('Origin',(4.225,-2.12788809108,3.34387696505));
#79962=CARTESIAN_POINT('',(4.35,-2.12788809108,2.34387696505));
#79963=CARTESIAN_POINT('',(4.325,-2.12788809108,2.34387696505));
#79964=CARTESIAN_POINT('Origin',(4.35,-2.12788809108,3.34387696505));
#79965=CARTESIAN_POINT('Origin',(0.,3.3773238354,2.34387696505));
#79966=CARTESIAN_POINT('',(4.35,2.8773238354,2.34387696505));
#79967=CARTESIAN_POINT('',(4.35,-1.95899712601,2.34387696505));
#79968=CARTESIAN_POINT('',(4.225,2.8773238354,2.34387696505));
#79969=CARTESIAN_POINT('Origin',(4.225,2.8773238354,1.84387696505));
#79970=CARTESIAN_POINT('',(4.35,3.3773238354,1.84387696505));
#79971=CARTESIAN_POINT('Origin',(4.35,2.8773238354,1.84387696505));
#79972=CARTESIAN_POINT('',(4.325,3.3773238354,1.84387696505));
#79973=CARTESIAN_POINT('Origin',(0.,3.3773238354,-4.15542016568));
#79974=CARTESIAN_POINT('',(4.35,3.3773238354,-3.65542016568));
#79975=CARTESIAN_POINT('',(4.35,3.3773238354,0.294579834316));
#79976=CARTESIAN_POINT('',(3.225,3.3773238354,-3.65542016568));
#79977=CARTESIAN_POINT('Origin',(3.225,2.8773238354,-3.65542016568));
#79978=CARTESIAN_POINT('',(4.35,2.8773238354,-4.15542016568));
#79979=CARTESIAN_POINT('Origin',(4.35,2.8773238354,-3.65542016568));
#79980=CARTESIAN_POINT('',(4.325,2.8773238354,-4.15542016568));
#79981=CARTESIAN_POINT('Ctrl Pts',(4.29232316291,-8.70602833393,-4.15542016568));
#79982=CARTESIAN_POINT('Ctrl Pts',(4.20764023978,-8.70455758206,-4.15542016896));
#79983=CARTESIAN_POINT('Ctrl Pts',(4.12295731665,-8.70308683019,-4.12553116451));
#79984=CARTESIAN_POINT('Ctrl Pts',(4.05251768323,-8.70186345223,-4.06549009434));
#79985=CARTESIAN_POINT('Ctrl Pts',(4.00958634297,-8.70111783143,-3.98660373227));
#79986=CARTESIAN_POINT('Ctrl Pts',(3.99616158804,-8.70088467363,-3.90297907486));
#79987=CARTESIAN_POINT('Ctrl Pts',(4.2942593567,-8.59454665965,-4.15542016568));
#79988=CARTESIAN_POINT('Ctrl Pts',(4.20834579354,-8.59289747109,-4.15542016627));
#79989=CARTESIAN_POINT('Ctrl Pts',(4.12243223039,-8.59124828254,-4.12466052278));
#79990=CARTESIAN_POINT('Ctrl Pts',(4.05139392587,-8.58988386074,-4.06285702325));
#79991=CARTESIAN_POINT('Ctrl Pts',(4.00903053768,-8.58906847866,-3.98200796497));
#79992=CARTESIAN_POINT('Ctrl Pts',(3.99712968313,-8.58883688841,-3.89688931333));
#79993=CARTESIAN_POINT('Ctrl Pts',(4.29645983294,-8.48273103918,-4.15542016568));
#79994=CARTESIAN_POINT('Ctrl Pts',(4.20896023779,-8.48105918371,-4.15542015758));
#79995=CARTESIAN_POINT('Ctrl Pts',(4.12146064264,-8.47938732823,-4.12352488429));
#79996=CARTESIAN_POINT('Ctrl Pts',(4.04967388507,-8.47801593608,-4.05942126033));
#79997=CARTESIAN_POINT('Ctrl Pts',(4.00810176319,-8.47722229641,-3.97603783242));
#79998=CARTESIAN_POINT('Ctrl Pts',(3.99822990786,-8.47703468918,-3.88903180855));
#79999=CARTESIAN_POINT('Ctrl Pts',(4.29855844641,-8.37042692805,-4.15542016568));
#80000=CARTESIAN_POINT('Ctrl Pts',(4.20912872342,-8.36895891499,-4.15542016568));
#80001=CARTESIAN_POINT('Ctrl Pts',(4.11969900043,-8.36749090194,-4.12211547602));
#80002=CARTESIAN_POINT('Ctrl Pts',(4.04704750378,-8.36630239191,-4.05515458588));
#80003=CARTESIAN_POINT('Ctrl Pts',(4.00655550671,-8.36564940222,-3.96867720994));
#80004=CARTESIAN_POINT('Ctrl Pts',(3.99927927276,-8.3655474023,-3.87944960348));
#80005=CARTESIAN_POINT('Ctrl Pts',(4.3,-8.25752787941,-4.15542016568));
#80006=CARTESIAN_POINT('Ctrl Pts',(4.20831114128,-8.25657123296,-4.15542016568));
#80007=CARTESIAN_POINT('Ctrl Pts',(4.11662228256,-8.2556145865,-4.12041892129));
#80008=CARTESIAN_POINT('Ctrl Pts',(4.04304033238,-8.25485845437,-4.05001401514));
#80009=CARTESIAN_POINT('Ctrl Pts',(4.00401954353,-8.25448277917,-3.95990362884));
#80010=CARTESIAN_POINT('Ctrl Pts',(4.,-8.25448277917,-3.86821477012));
#80011=CARTESIAN_POINT('Ctrl Pts',(4.3,-8.14391944342,-4.15542016568));
#80012=CARTESIAN_POINT('Ctrl Pts',(4.20575222039,-8.14391944342,-4.15542016568));
#80013=CARTESIAN_POINT('Ctrl Pts',(4.11150444078,-8.14391944342,-4.11840914918));
#80014=CARTESIAN_POINT('Ctrl Pts',(4.0370110165,-8.14391944342,-4.0439157249));
#80015=CARTESIAN_POINT('Ctrl Pts',(4.,-8.14391944342,-3.94966794529));
#80016=CARTESIAN_POINT('Ctrl Pts',(4.,-8.14391944342,-3.85542016568));
#80017=CARTESIAN_POINT('',(4.29232316258844,-8.70602835244453,-4.15542016568));
#80018=CARTESIAN_POINT('Origin',(4.29069091406768,-8.70599998041311,-3.85733575579212));
#80019=CARTESIAN_POINT('Ctrl Pts',(4.3,-8.14391944342,-4.15542016568));
#80020=CARTESIAN_POINT('Ctrl Pts',(4.3,-8.20648904053108,-4.15542016568));
#80021=CARTESIAN_POINT('Ctrl Pts',(4.29947971883186,-8.26880371250586,-4.15542016568));
#80022=CARTESIAN_POINT('Ctrl Pts',(4.29869536600186,-8.33090046659907,-4.15542016568));
#80023=CARTESIAN_POINT('Ctrl Pts',(4.29790074267177,-8.39381033016885,-4.15542016568));
#80024=CARTESIAN_POINT('Ctrl Pts',(4.29683500095811,-8.45649622088276,-4.15542016568));
#80025=CARTESIAN_POINT('Ctrl Pts',(4.29571075913684,-8.51899937638185,-4.15542016568));
#80026=CARTESIAN_POINT('Ctrl Pts',(4.29458651731557,-8.58150253188095,-4.15542016568));
#80027=CARTESIAN_POINT('Ctrl Pts',(4.2934034804918,-8.64382608258768,-4.15542016568));
#80028=CARTESIAN_POINT('Ctrl Pts',(4.29232316291,-8.70602833393,-4.15542016568));
#80029=CARTESIAN_POINT('Origin',(0.,3.3773238354,-4.15542016568));
#80030=CARTESIAN_POINT('',(3.69999999774,-9.41827086749,-4.15542016568));
#80031=CARTESIAN_POINT('Ctrl Pts',(4.29232316225885,-8.70602837142191,-4.15542016568));
#80032=CARTESIAN_POINT('Ctrl Pts',(4.29205120071452,-8.72168753702626,-4.15542016568));
#80033=CARTESIAN_POINT('Ctrl Pts',(4.29158720532918,-8.73740648674787,-4.15542016568278));
#80034=CARTESIAN_POINT('Ctrl Pts',(4.29086254081513,-8.75324772180714,-4.15542016514087));
#80035=CARTESIAN_POINT('Ctrl Pts',(4.29008645301039,-8.77021307488149,-4.15542016456051));
#80036=CARTESIAN_POINT('Ctrl Pts',(4.28901119399487,-8.7873184421748,-4.15542016334628));
#80037=CARTESIAN_POINT('Ctrl Pts',(4.28754966268177,-8.80457940448153,-4.15542016341833));
#80038=CARTESIAN_POINT('Ctrl Pts',(4.28677487233489,-8.81372982558667,-4.15542016345652));
#80039=CARTESIAN_POINT('Ctrl Pts',(4.28589150051295,-8.8229229964194,-4.15542016392521));
#80040=CARTESIAN_POINT('Ctrl Pts',(4.28488660862881,-8.83215545542406,-4.15542016457497));
#80041=CARTESIAN_POINT('Ctrl Pts',(4.28275134959082,-8.85177317932411,-4.15542016595563));
#80042=CARTESIAN_POINT('Ctrl Pts',(4.28003832504559,-8.87155237324264,-4.15542016566606));
#80043=CARTESIAN_POINT('Ctrl Pts',(4.27662963897357,-8.89139030340002,-4.15542016567672));
#80044=CARTESIAN_POINT('Ctrl Pts',(4.27453046995187,-8.90360708357898,-4.15542016568329));
#80045=CARTESIAN_POINT('Ctrl Pts',(4.27216774709283,-8.91584486940965,-4.15542016568));
#80046=CARTESIAN_POINT('Ctrl Pts',(4.26951780859382,-8.92807096217797,-4.15542016568));
#80047=CARTESIAN_POINT('Ctrl Pts',(4.26468368982784,-8.95037426638974,-4.15542016568));
#80048=CARTESIAN_POINT('Ctrl Pts',(4.25889294909336,-8.97263030125832,-4.15542016568));
#80049=CARTESIAN_POINT('Ctrl Pts',(4.25202546552033,-8.99462871319934,-4.15542016568));
#80050=CARTESIAN_POINT('Ctrl Pts',(4.24866331428397,-9.00539859522655,-4.15542016568));
#80051=CARTESIAN_POINT('Ctrl Pts',(4.24504378092221,-9.01610634900063,-4.15542016568));
#80052=CARTESIAN_POINT('Ctrl Pts',(4.24115737109246,-9.02672676812152,-4.15542016568));
#80053=CARTESIAN_POINT('Ctrl Pts',(4.23426685680616,-9.04555652434511,-4.15542016568));
#80054=CARTESIAN_POINT('Ctrl Pts',(4.22653159494977,-9.06411864425602,-4.15542016568));
#80055=CARTESIAN_POINT('Ctrl Pts',(4.21793147778923,-9.08227287068491,-4.15542016568));
#80056=CARTESIAN_POINT('Ctrl Pts',(4.2100789353958,-9.0988490207526,-4.15542016568));
#80057=CARTESIAN_POINT('Ctrl Pts',(4.2015054941613,-9.11508438284678,-4.15542016568));
#80058=CARTESIAN_POINT('Ctrl Pts',(4.1922309596074,-9.13089839049763,-4.15542016568));
#80059=CARTESIAN_POINT('Ctrl Pts',(4.18815592541805,-9.13784673075918,-4.15542016568));
#80060=CARTESIAN_POINT('Ctrl Pts',(4.1839460127474,-9.14471414658231,-4.15542016568));
#80061=CARTESIAN_POINT('Ctrl Pts',(4.17960523291625,-9.1514961102524,-4.15542016568));
#80062=CARTESIAN_POINT('Ctrl Pts',(4.16634611145727,-9.17221194554702,-4.15542016568));
#80063=CARTESIAN_POINT('Ctrl Pts',(4.15184518108592,-9.19211860151861,-4.15542016617984));
#80064=CARTESIAN_POINT('Ctrl Pts',(4.13618163257724,-9.21102766582222,-4.15542016179659));
#80065=CARTESIAN_POINT('Ctrl Pts',(4.11973553103685,-9.23088142957176,-4.15542015719435));
#80066=CARTESIAN_POINT('Ctrl Pts',(4.10200809428551,-9.24963529413492,-4.15542014577611));
#80067=CARTESIAN_POINT('Ctrl Pts',(4.08313350202983,-9.26711150454399,-4.15542013374396));
#80068=CARTESIAN_POINT('Ctrl Pts',(4.07176321009623,-9.27763939365293,-4.15542012649563));
#80069=CARTESIAN_POINT('Ctrl Pts',(4.05997740445791,-9.28770440729055,-4.15542011955517));
#80070=CARTESIAN_POINT('Ctrl Pts',(4.04781138042469,-9.29727441845877,-4.15542011643421));
#80071=CARTESIAN_POINT('Ctrl Pts',(4.02659799740219,-9.31396124333162,-4.15542011099231));
#80072=CARTESIAN_POINT('Ctrl Pts',(4.00423092936188,-9.32913206089668,-4.15542011535558));
#80073=CARTESIAN_POINT('Ctrl Pts',(3.98091614962384,-9.34262747027809,-4.15542012343284));
#80074=CARTESIAN_POINT('Ctrl Pts',(3.95650110095926,-9.3567597537694,-4.15542013189127));
#80075=CARTESIAN_POINT('Ctrl Pts',(3.93104736555546,-9.36905451674416,-4.15542014341187));
#80076=CARTESIAN_POINT('Ctrl Pts',(3.90483049009711,-9.37937035892166,-4.15542015118524));
#80077=CARTESIAN_POINT('Ctrl Pts',(3.89672696602562,-9.38255894161665,-4.15542015358796));
#80078=CARTESIAN_POINT('Ctrl Pts',(3.88855076480426,-9.38555876112294,-4.15542015568561));
#80079=CARTESIAN_POINT('Ctrl Pts',(3.88031058139973,-9.38836645220462,-4.1554201574361));
#80080=CARTESIAN_POINT('Ctrl Pts',(3.85132370712238,-9.39824319698063,-4.15542016359385));
#80081=CARTESIAN_POINT('Ctrl Pts',(3.82154088715569,-9.40573335220575,-4.15542016471136));
#80082=CARTESIAN_POINT('Ctrl Pts',(3.79135695696281,-9.41074020445555,-4.15542016528016));
#80083=CARTESIAN_POINT('Ctrl Pts',(3.76117302676992,-9.41574705670534,-4.15542016584896));
#80084=CARTESIAN_POINT('Ctrl Pts',(3.73058948857333,-9.41827087355667,-4.15542016568));
#80085=CARTESIAN_POINT('Ctrl Pts',(3.69999999774,-9.41827086749,-4.15542016568));
#80086=CARTESIAN_POINT('',(2.3,-9.41827086707,-4.15542016568));
#80087=CARTESIAN_POINT('',(3.225,-9.41827086707,-4.15542016568));
#80088=CARTESIAN_POINT('',(2.3,-10.0779006799,-4.15542016568));
#80089=CARTESIAN_POINT('',(2.3,-8.20939783898,-4.15542016568));
#80090=CARTESIAN_POINT('',(4.35,-10.0779006799,-4.15542016568));
#80091=CARTESIAN_POINT('',(3.225,-10.0779006799,-4.15542016568));
#80092=CARTESIAN_POINT('',(4.35,-1.95899712601,-4.15542016568));
#80093=CARTESIAN_POINT('Ctrl Pts',(4.29232279844,-8.70602816471,5.10274328646));
#80094=CARTESIAN_POINT('Ctrl Pts',(4.20763985549,-8.70455745139,5.10274332142));
#80095=CARTESIAN_POINT('Ctrl Pts',(4.12295691253,-8.70308673807,5.07285428042));
#80096=CARTESIAN_POINT('Ctrl Pts',(4.05251729593,-8.70186339274,5.01281309848));
#80097=CARTESIAN_POINT('Ctrl Pts',(4.00958603902,-8.70111779311,4.93392659864));
#80098=CARTESIAN_POINT('Ctrl Pts',(3.99616141568,-8.70088464377,4.85030182916));
#80099=CARTESIAN_POINT('Ctrl Pts',(4.29367604164,-8.62810126572,5.10274328646));
#80100=CARTESIAN_POINT('Ctrl Pts',(4.20813285855,-8.6265058463,5.10274333195));
#80101=CARTESIAN_POINT('Ctrl Pts',(4.12258967546,-8.62491042687,5.07224568401));
#80102=CARTESIAN_POINT('Ctrl Pts',(4.0517315901,-8.62358850977,5.01097248773));
#80103=CARTESIAN_POINT('Ctrl Pts',(4.00919737959,-8.62279415849,4.93071397417));
#80104=CARTESIAN_POINT('Ctrl Pts',(3.99683804383,-8.62256210931,4.84604483372));
#80105=CARTESIAN_POINT('Ctrl Pts',(4.29515862692,-8.55000353482,5.10274328646));
#80106=CARTESIAN_POINT('Ctrl Pts',(4.20858147867,-8.54835950303,5.10274332811));
#80107=CARTESIAN_POINT('Ctrl Pts',(4.12200433041,-8.54671547124,5.07150754218));
#80108=CARTESIAN_POINT('Ctrl Pts',(4.05065454881,-8.5453604781,5.00873951265));
#80109=CARTESIAN_POINT('Ctrl Pts',(4.0086265191,-8.54456207669,4.92682955987));
#80110=CARTESIAN_POINT('Ctrl Pts',(3.99757933996,-8.54435185028,4.84092376899));
#80111=CARTESIAN_POINT('Ctrl Pts',(4.2966466112,-8.47169636018,5.10274328646));
#80112=CARTESIAN_POINT('Ctrl Pts',(4.20886559395,-8.47010372313,5.10274328646));
#80113=CARTESIAN_POINT('Ctrl Pts',(4.12108457671,-8.46851108607,5.0706369892));
#80114=CARTESIAN_POINT('Ctrl Pts',(4.049181176,-8.4672075164,5.00610503411));
#80115=CARTESIAN_POINT('Ctrl Pts',(4.00779063879,-8.46645935943,4.92226864646));
#80116=CARTESIAN_POINT('Ctrl Pts',(3.99832332564,-8.46629167717,4.83495432364));
#80117=CARTESIAN_POINT('Ctrl Pts',(4.29796673138,-8.39314927373,5.10274328646));
#80118=CARTESIAN_POINT('Ctrl Pts',(4.20881731963,-8.39173518355,5.10274328646));
#80119=CARTESIAN_POINT('Ctrl Pts',(4.11966790787,-8.39032109337,5.06963007213));
#80120=CARTESIAN_POINT('Ctrl Pts',(4.04716501903,-8.3891735059,5.00305604873));
#80121=CARTESIAN_POINT('Ctrl Pts',(4.00657458492,-8.38853640885,4.91702461127));
#80122=CARTESIAN_POINT('Ctrl Pts',(3.99898336569,-8.38842527481,4.8281587616));
#80123=CARTESIAN_POINT('Ctrl Pts',(4.29889875178,-8.31430322211,5.10274328646));
#80124=CARTESIAN_POINT('Ctrl Pts',(4.20822334583,-8.31323136973,5.10274328646));
#80125=CARTESIAN_POINT('Ctrl Pts',(4.11754793987,-8.31215951735,5.06848004433));
#80126=CARTESIAN_POINT('Ctrl Pts',(4.04442178691,-8.31129511051,4.99957103487));
#80127=CARTESIAN_POINT('Ctrl Pts',(4.00483540394,-8.3108271693,4.91108461112));
#80128=CARTESIAN_POINT('Ctrl Pts',(3.99944937589,-8.31076350235,4.82056298519));
#80129=CARTESIAN_POINT('',(4.29889875895,-8.31430322211008,5.10274332057));
#80130=CARTESIAN_POINT('Origin',(4.29696586920653,-8.31428039305215,4.80479476356497));
#80131=CARTESIAN_POINT('',(4.29232279670749,-8.70602826446416,5.10274328645992));
#80132=CARTESIAN_POINT('Ctrl Pts',(4.29232279844,-8.70602816471,5.10274328646));
#80133=CARTESIAN_POINT('Ctrl Pts',(4.29367604164,-8.62810126572,5.10274328646));
#80134=CARTESIAN_POINT('Ctrl Pts',(4.29515862692,-8.55000353482,5.10274328646));
#80135=CARTESIAN_POINT('Ctrl Pts',(4.2966466112,-8.47169636018,5.10274328646));
#80136=CARTESIAN_POINT('Ctrl Pts',(4.29796673138,-8.39314927373,5.10274328646));
#80137=CARTESIAN_POINT('Ctrl Pts',(4.29889875178,-8.31430322211,5.10274328646));
#80138=CARTESIAN_POINT('Origin',(4.29068847369796,-8.70599943725965,4.80466191947753));
#80139=CARTESIAN_POINT('Ctrl Pts',(4.29889876134,-8.31430322282,5.1027434229));
#80140=CARTESIAN_POINT('Ctrl Pts',(4.2082233452,-8.31323138881,5.10274342246));
#80141=CARTESIAN_POINT('Ctrl Pts',(4.11754792907,-8.31215955225,5.0684801702));
#80142=CARTESIAN_POINT('Ctrl Pts',(4.04442177042,-8.31129515513,4.99957114081));
#80143=CARTESIAN_POINT('Ctrl Pts',(4.00483538997,-8.31082721545,4.91108469399));
#80144=CARTESIAN_POINT('Ctrl Pts',(3.99944937087,-8.31076354298,4.8205630482));
#80145=CARTESIAN_POINT('Ctrl Pts',(4.29964314059,-8.22434260602,5.1027436292));
#80146=CARTESIAN_POINT('Ctrl Pts',(4.20780699632,-8.22403023518,5.10264720521));
#80147=CARTESIAN_POINT('Ctrl Pts',(4.11597085206,-8.22680019636,5.06741723002));
#80148=CARTESIAN_POINT('Ctrl Pts',(4.0423682592,-8.23275280902,4.99666339283));
#80149=CARTESIAN_POINT('Ctrl Pts',(4.00353912359,-8.24059165767,4.90627699718));
#80150=CARTESIAN_POINT('Ctrl Pts',(3.99982155439,-8.24873700866,4.81449657867));
#80151=CARTESIAN_POINT('Ctrl Pts',(4.29971371834,-8.13469356333,5.09262744205));
#80152=CARTESIAN_POINT('Ctrl Pts',(4.20724144925,-8.13466365636,5.09260573663));
#80153=CARTESIAN_POINT('Ctrl Pts',(4.11476918016,-8.14098347585,5.05729879766));
#80154=CARTESIAN_POINT('Ctrl Pts',(4.04093270982,-8.15373242653,4.98629044613));
#80155=CARTESIAN_POINT('Ctrl Pts',(4.00258694952,-8.1700271987,4.89579754059));
#80156=CARTESIAN_POINT('Ctrl Pts',(3.99985686503,-8.18656139935,4.80428277208));
#80157=CARTESIAN_POINT('Ctrl Pts',(4.29971786827,-8.04665414995,5.07253279403));
#80158=CARTESIAN_POINT('Ctrl Pts',(4.20720101416,-8.04666571693,5.07252348963));
#80159=CARTESIAN_POINT('Ctrl Pts',(4.11468416006,-8.05626571803,5.0379315222));
#80160=CARTESIAN_POINT('Ctrl Pts',(4.04083150668,-8.07556834767,4.96834669024));
#80161=CARTESIAN_POINT('Ctrl Pts',(4.00251997495,-8.10013935979,4.87966809703));
#80162=CARTESIAN_POINT('Ctrl Pts',(3.9998589855,-8.12494698597,4.78999433407));
#80163=CARTESIAN_POINT('Ctrl Pts',(4.29967705707,-7.96150927709,5.0427549913));
#80164=CARTESIAN_POINT('Ctrl Pts',(4.20771171282,-7.96176972051,5.0427867655));
#80165=CARTESIAN_POINT('Ctrl Pts',(4.11574636857,-7.97452633141,5.00973042736));
#80166=CARTESIAN_POINT('Ctrl Pts',(4.04209470673,-7.99987188278,4.94319135382));
#80167=CARTESIAN_POINT('Ctrl Pts',(4.00335979512,-8.03206135592,4.85814590158));
#80168=CARTESIAN_POINT('Ctrl Pts',(3.99983852853,-8.06458049923,4.77178934946));
#80169=CARTESIAN_POINT('Ctrl Pts',(4.29902733552,-7.88049121843,5.00374669681));
#80170=CARTESIAN_POINT('Ctrl Pts',(4.20814475196,-7.88133646016,5.00415366088));
#80171=CARTESIAN_POINT('Ctrl Pts',(4.1172621684,-7.89711301226,4.97354912353));
#80172=CARTESIAN_POINT('Ctrl Pts',(4.04405132352,-7.92782452293,4.91150502168));
#80173=CARTESIAN_POINT('Ctrl Pts',(4.00460096887,-7.96672185729,4.83165611315));
#80174=CARTESIAN_POINT('Ctrl Pts',(3.99951366776,-8.00613540701,4.74991741048));
#80175=CARTESIAN_POINT('Ctrl Pts',(4.29889876134,-8.31430322211031,5.1027434229));
#80176=CARTESIAN_POINT('Ctrl Pts',(4.29920344163676,-8.27748162914417,5.10274350731409));
#80177=CARTESIAN_POINT('Ctrl Pts',(4.29937856313619,-8.24035941587499,5.10070757013621));
#80178=CARTESIAN_POINT('Ctrl Pts',(4.29948883773587,-8.2031747831764,5.09654944157962));
#80179=CARTESIAN_POINT('Ctrl Pts',(4.29959662290323,-8.16682958790246,5.09248518214244));
#80180=CARTESIAN_POINT('Ctrl Pts',(4.29964284554375,-8.13042504980527,5.08639342033935));
#80181=CARTESIAN_POINT('Ctrl Pts',(4.29965086041858,-8.09420012940637,5.0782197064064));
#80182=CARTESIAN_POINT('Ctrl Pts',(4.29965889627944,-8.05788035824006,5.07002459054819));
#80183=CARTESIAN_POINT('Ctrl Pts',(4.29962900470861,-8.02174138997864,5.05973647485076));
#80184=CARTESIAN_POINT('Ctrl Pts',(4.2995403127252,-7.98603700409252,5.04732841046897));
#80185=CARTESIAN_POINT('Ctrl Pts',(4.2994516207418,-7.9503326182064,5.03492034608718));
#80186=CARTESIAN_POINT('Ctrl Pts',(4.29930451946122,-7.91506308836291,5.02039224105907));
#80187=CARTESIAN_POINT('Ctrl Pts',(4.29902725090631,-7.88049121921695,5.00374669718888));
#80188=CARTESIAN_POINT('Ctrl Pts',(3.7,-9.1392576487296,4.91297769122882));
#80189=CARTESIAN_POINT('Ctrl Pts',(3.7,-9.0282774958267,4.63207689326605));
#80190=CARTESIAN_POINT('Ctrl Pts',(3.7,-8.72799905369119,4.59960059693865));
#80191=CARTESIAN_POINT('Ctrl Pts',(3.95543243199934,-9.1392576487296,4.91297769122882));
#80192=CARTESIAN_POINT('Ctrl Pts',(3.95543243199934,-9.0282774958267,4.63207689326605));
#80193=CARTESIAN_POINT('Ctrl Pts',(3.95543243199934,-8.72799905369119,4.59960059693865));
#80194=CARTESIAN_POINT('Ctrl Pts',(3.99616169510398,-8.90473369905756,5.00563497089039));
#80195=CARTESIAN_POINT('Ctrl Pts',(3.99616169510398,-8.84972402020801,4.86640050166025));
#80196=CARTESIAN_POINT('Ctrl Pts',(3.99616169510398,-8.70088460851816,4.85030293300078));
#80197=CARTESIAN_POINT('',(3.7,-9.13925764671,4.9129776861));
#80198=CARTESIAN_POINT('Origin',(3.7,-8.67423561284,5.09670168568));
#80199=CARTESIAN_POINT('Ctrl Pts',(3.7,-9.13925764671,4.9129776861));
#80200=CARTESIAN_POINT('Ctrl Pts',(3.75706459059,-9.13925765647,4.9129776858));
#80201=CARTESIAN_POINT('Ctrl Pts',(3.81411802643,-9.12422889542,4.91173129034));
#80202=CARTESIAN_POINT('Ctrl Pts',(3.86651403782,-9.0935734628,4.90972003087));
#80203=CARTESIAN_POINT('Ctrl Pts',(3.94373685893,-9.0162718551,4.90110872718));
#80204=CARTESIAN_POINT('Ctrl Pts',(3.98361771521,-8.90210958415,4.88238701109));
#80205=CARTESIAN_POINT('Ctrl Pts',(3.99224364397,-8.84501961539,4.86859296944));
#80206=CARTESIAN_POINT('Ctrl Pts',(3.99540042025,-8.7740131878,4.85347142938));
#80207=CARTESIAN_POINT('Ctrl Pts',(3.99616169511,-8.70088460852,4.850302933));
#80208=CARTESIAN_POINT('Origin',(0.,-9.17423561284,0.47366156039));
#80209=CARTESIAN_POINT('',(2.3,-8.7279990537,4.59960059693));
#80210=CARTESIAN_POINT('',(2.3,-8.7279990537,-3.65227747616));
#80211=CARTESIAN_POINT('Origin',(2.3,-9.17423561284,0.47366156039));
#80212=CARTESIAN_POINT('',(3.,-8.7279990537,-3.65227747616));
#80213=CARTESIAN_POINT('',(3.,-8.7279990537,4.59960059693));
#80214=CARTESIAN_POINT('Ctrl Pts',(3.7,-8.72799905369119,-3.65227747615864));
#80215=CARTESIAN_POINT('Ctrl Pts',(3.7,-9.0282774958225,-3.68475377248559));
#80216=CARTESIAN_POINT('Ctrl Pts',(3.7,-9.13925764872732,-3.96565457044306));
#80217=CARTESIAN_POINT('Ctrl Pts',(3.95543192438937,-8.72799905369119,-3.65227747615864));
#80218=CARTESIAN_POINT('Ctrl Pts',(3.95543192438937,-9.0282774958225,-3.68475377248559));
#80219=CARTESIAN_POINT('Ctrl Pts',(3.95543192438937,-9.13925764872732,-3.96565457044306));
#80220=CARTESIAN_POINT('Ctrl Pts',(3.99616160125782,-8.70088467099341,-3.90297923456964));
#80221=CARTESIAN_POINT('Ctrl Pts',(3.99616160125782,-8.84972443161661,-3.91907684096763));
#80222=CARTESIAN_POINT('Ctrl Pts',(3.99616160125782,-8.90473423943044,-4.05831163661298));
#80223=CARTESIAN_POINT('',(3.7,-9.13925764671,-3.96565456533));
#80224=CARTESIAN_POINT('Origin',(3.7,-8.67423561284,-4.1493785649));
#80225=CARTESIAN_POINT('Ctrl Pts',(3.99616160126,-8.700884671,-3.90297923457));
#80226=CARTESIAN_POINT('Ctrl Pts',(3.99540042025,-8.7740131878,-3.9061483086));
#80227=CARTESIAN_POINT('Ctrl Pts',(3.99224364397,-8.84501961539,-3.92126984866));
#80228=CARTESIAN_POINT('Ctrl Pts',(3.98361771521,-8.90210958415,-3.93506389031));
#80229=CARTESIAN_POINT('Ctrl Pts',(3.94373685893,-9.0162718551,-3.9537856064));
#80230=CARTESIAN_POINT('Ctrl Pts',(3.86651403782,-9.0935734628,-3.96239691009));
#80231=CARTESIAN_POINT('Ctrl Pts',(3.81411802643,-9.12422889542,-3.96440816956));
#80232=CARTESIAN_POINT('Ctrl Pts',(3.75706459059,-9.13925765647,-3.96565456502));
#80233=CARTESIAN_POINT('Ctrl Pts',(3.7,-9.13925764671,-3.96565456533));
#80234=CARTESIAN_POINT('Origin',(4.35,2.13070110951,0.294579834316));
#80235=CARTESIAN_POINT('',(4.45,-2.51831889439,2.53297389574));
#80236=CARTESIAN_POINT('Origin',(4.35,-2.51831889439,2.53297389574));
#80237=CARTESIAN_POINT('',(4.45,-7.83711001806,5.09384703785));
#80238=CARTESIAN_POINT('',(4.45,-5.17771445623,3.81341046679));
#80239=CARTESIAN_POINT('Origin',(4.35,-7.83711001806,5.09384703785));
#80240=CARTESIAN_POINT('Origin',(3.225,-8.31430322211,4.10274328646));
#80241=CARTESIAN_POINT('',(4.35,-8.31430322211,5.10274328646));
#80242=CARTESIAN_POINT('Origin',(4.35,-8.31430322211,4.10274328646));
#80243=CARTESIAN_POINT('',(4.32444937589,-8.31430322211,5.10274328646));
#80244=CARTESIAN_POINT('Origin',(4.35,-2.12788809108,3.34387696505));
#80245=CARTESIAN_POINT('',(4.45,-2.12788809108,2.44387696505));
#80246=CARTESIAN_POINT('Origin',(4.35,-2.12788809108,2.44387696505));
#80247=CARTESIAN_POINT('Origin',(4.45,-2.12788809108,3.34387696505));
#80248=CARTESIAN_POINT('Origin',(4.35,-1.95899712601,2.44387696505));
#80249=CARTESIAN_POINT('',(4.45,2.8773238354,2.44387696505));
#80250=CARTESIAN_POINT('Origin',(4.35,2.8773238354,2.44387696505));
#80251=CARTESIAN_POINT('',(4.45,0.374717872161,2.44387696505));
#80252=CARTESIAN_POINT('Origin',(4.35,2.8773238354,1.84387696505));
#80253=CARTESIAN_POINT('',(4.45,3.4773238354,1.84387696505));
#80254=CARTESIAN_POINT('Origin',(4.35,3.4773238354,1.84387696505));
#80255=CARTESIAN_POINT('Origin',(4.45,2.8773238354,1.84387696505));
#80256=CARTESIAN_POINT('Origin',(4.35,3.4773238354,0.294579834316));
#80257=CARTESIAN_POINT('',(4.45,3.4773238354,-3.65542016568));
#80258=CARTESIAN_POINT('Origin',(4.35,3.4773238354,-3.65542016568));
#80259=CARTESIAN_POINT('',(4.45,3.4773238354,-0.905771600316));
#80260=CARTESIAN_POINT('Origin',(4.35,2.8773238354,-3.65542016568));
#80261=CARTESIAN_POINT('',(4.45,2.8773238354,-4.25542016568));
#80262=CARTESIAN_POINT('Origin',(4.35,2.8773238354,-4.25542016568));
#80263=CARTESIAN_POINT('Origin',(4.45,2.8773238354,-3.65542016568));
#80264=CARTESIAN_POINT('Ctrl Pts',(3.69999999774,-9.41827086749,-4.15542016568));
#80265=CARTESIAN_POINT('Ctrl Pts',(3.69999999833,-9.34659890209,-4.15542016568));
#80266=CARTESIAN_POINT('Ctrl Pts',(3.69999999892,-9.2749269367,-4.13401653812));
#80267=CARTESIAN_POINT('Ctrl Pts',(3.69999999944,-9.21183540432,-4.09110601764));
#80268=CARTESIAN_POINT('Ctrl Pts',(3.69999999982,-9.16559336719,-4.03231265157));
#80269=CARTESIAN_POINT('Ctrl Pts',(3.70000000003,-9.13925764692,-3.96565456539));
#80270=CARTESIAN_POINT('Ctrl Pts',(3.81412909821,-9.41827089013,-4.15542016568));
#80271=CARTESIAN_POINT('Ctrl Pts',(3.79947056194,-9.34659892134,-4.15542016565));
#80272=CARTESIAN_POINT('Ctrl Pts',(3.78481202566,-9.27492695255,-4.13401653803));
#80273=CARTESIAN_POINT('Ctrl Pts',(3.77190837788,-9.21183541723,-4.09110601746));
#80274=CARTESIAN_POINT('Ctrl Pts',(3.76245084042,-9.16559337792,-4.03231265129));
#80275=CARTESIAN_POINT('Ctrl Pts',(3.75706459059,-9.13925765647,-3.96565456502));
#80276=CARTESIAN_POINT('Ctrl Pts',(3.92823594404,-9.38909765086,-4.15542016568));
#80277=CARTESIAN_POINT('Ctrl Pts',(3.89892199959,-9.32091627439,-4.15542016461));
#80278=CARTESIAN_POINT('Ctrl Pts',(3.86960805513,-9.25273489792,-4.13385699888));
#80279=CARTESIAN_POINT('Ctrl Pts',(3.84380320278,-9.19278171906,-4.0906252646));
#80280=CARTESIAN_POINT('Ctrl Pts',(3.82488943837,-9.14898176867,-4.03143501908));
#80281=CARTESIAN_POINT('Ctrl Pts',(3.81411802643,-9.12422889542,-3.96440816956));
#80282=CARTESIAN_POINT('Ctrl Pts',(4.03302804821,-9.33107957038,-4.15542016568));
#80283=CARTESIAN_POINT('Ctrl Pts',(3.99017706972,-9.2696193654,-4.1554201695));
#80284=CARTESIAN_POINT('Ctrl Pts',(3.94732609124,-9.20815916043,-4.13359925186));
#80285=CARTESIAN_POINT('Ctrl Pts',(3.90964076698,-9.15426319663,-4.0898484638));
#80286=CARTESIAN_POINT('Ctrl Pts',(3.8820963349,-9.11520770945,-4.03001850758));
#80287=CARTESIAN_POINT('Ctrl Pts',(3.86651403782,-9.0935734628,-3.96239691009));
#80288=CARTESIAN_POINT('Ctrl Pts',(4.18747374061,-9.18016437508,-4.15542016568));
#80289=CARTESIAN_POINT('Ctrl Pts',(4.12388018645,-9.13700016797,-4.15542016252));
#80290=CARTESIAN_POINT('Ctrl Pts',(4.0602866323,-9.09383596087,-4.13249096908));
#80291=CARTESIAN_POINT('Ctrl Pts',(4.00475631151,-9.05633061601,-4.08650843459));
#80292=CARTESIAN_POINT('Ctrl Pts',(3.96503122609,-9.029900996,-4.02393293739));
#80293=CARTESIAN_POINT('Ctrl Pts',(3.94373685893,-9.0162718551,-3.9537856064));
#80294=CARTESIAN_POINT('Ctrl Pts',(4.26723541157,-8.98063713586,-4.15542016568));
#80295=CARTESIAN_POINT('Ctrl Pts',(4.19077919927,-8.95915602901,-4.1554201683));
#80296=CARTESIAN_POINT('Ctrl Pts',(4.11432298698,-8.93767492216,-4.13000304884));
#80297=CARTESIAN_POINT('Ctrl Pts',(4.04869892936,-8.91937700045,-4.07900263159));
#80298=CARTESIAN_POINT('Ctrl Pts',(4.00420277032,-8.90727654877,-4.01043652908));
#80299=CARTESIAN_POINT('Ctrl Pts',(3.98361771521,-8.90210958415,-3.93506389031));
#80300=CARTESIAN_POINT('Ctrl Pts',(4.28448738522,-8.88291546038,-4.15542016568));
#80301=CARTESIAN_POINT('Ctrl Pts',(4.2038128468,-8.87211558957,-4.15542016079));
#80302=CARTESIAN_POINT('Ctrl Pts',(4.12313830838,-8.86131571876,-4.12815293378));
#80303=CARTESIAN_POINT('Ctrl Pts',(4.05474416619,-8.85231492765,-4.07341965826));
#80304=CARTESIAN_POINT('Ctrl Pts',(4.01023278232,-8.84679291313,-4.00043036345));
#80305=CARTESIAN_POINT('Ctrl Pts',(3.99224364397,-8.84501961539,-3.92126984866));
#80306=CARTESIAN_POINT('Ctrl Pts',(4.2908008405,-8.79368075155,-4.15542016568));
#80307=CARTESIAN_POINT('Ctrl Pts',(4.20683195096,-8.78806573108,-4.15542016568));
#80308=CARTESIAN_POINT('Ctrl Pts',(4.12286306143,-8.78245071061,-4.12598423857));
#80309=CARTESIAN_POINT('Ctrl Pts',(4.05279621082,-8.77777630692,-4.06686040464));
#80310=CARTESIAN_POINT('Ctrl Pts',(4.00960658253,-8.77491887358,-3.98899545804));
#80311=CARTESIAN_POINT('Ctrl Pts',(3.99540042025,-8.7740131878,-3.9061483086));
#80312=CARTESIAN_POINT('Ctrl Pts',(4.29232317424,-8.70602837163,-4.15542016568));
#80313=CARTESIAN_POINT('Ctrl Pts',(4.20764026079,-8.70455761115,-4.15542016568));
#80314=CARTESIAN_POINT('Ctrl Pts',(4.12295734733,-8.70308685067,-4.12553116999));
#80315=CARTESIAN_POINT('Ctrl Pts',(4.05251771609,-8.70186346543,-4.06549012145));
#80316=CARTESIAN_POINT('Ctrl Pts',(4.00958636427,-8.70111783998,-3.98660378483));
#80317=CARTESIAN_POINT('Ctrl Pts',(3.99616158712,-8.70088468041,-3.90297914754));
#80318=CARTESIAN_POINT('Origin',(3.69999999519659,-9.41833116541397,-3.85533150874716));
#80319=CARTESIAN_POINT('Origin',(3.225,-9.41827086707,-3.85542016568));
#80320=CARTESIAN_POINT('',(2.3,-9.13925764673,-3.96565456539));
#80321=CARTESIAN_POINT('Origin',(2.3,-9.41827086707,-3.85542016568));
#80322=CARTESIAN_POINT('',(3.,-9.13925764673,-3.96565456539));
#80323=CARTESIAN_POINT('Origin',(2.3,-8.20939783898,-3.85542016568));
#80324=CARTESIAN_POINT('',(2.,-9.41827086707,-3.85542016568));
#80325=CARTESIAN_POINT('',(2.,-10.0779006799,-3.85542016568));
#80326=CARTESIAN_POINT('',(2.,-9.7480857735,-3.85542016568));
#80327=CARTESIAN_POINT('Origin',(2.3,-10.0779006799,-3.85542016568));
#80328=CARTESIAN_POINT('Origin',(2.3,-9.41827086707,-3.85542016568));
#80329=CARTESIAN_POINT('Origin',(3.225,-10.0779006799,-3.15542016568));
#80330=CARTESIAN_POINT('',(4.35,-10.4977210429,-4.06302738404));
#80331=CARTESIAN_POINT('Origin',(4.35,-10.0779006799,-3.15542016568));
#80332=CARTESIAN_POINT('',(2.3,-10.4977210429,-4.06302738404));
#80333=CARTESIAN_POINT('Origin',(2.3,-10.0779006799,-3.15542016568));
#80334=CARTESIAN_POINT('',(3.325,-10.4977210429,-4.06302738404));
#80335=CARTESIAN_POINT('Origin',(4.35,-1.95899712601,-4.25542016568));
#80336=CARTESIAN_POINT('',(4.45,-10.0779006799,-4.25542016568));
#80337=CARTESIAN_POINT('Origin',(4.35,-10.0779006799,-4.25542016568));
#80338=CARTESIAN_POINT('',(4.45,-3.60028842226,-4.25542016568));
#80339=CARTESIAN_POINT('Origin',(0.,-8.08610163061,5.10274328646));
#80340=CARTESIAN_POINT('',(4.35,-12.9053426461,5.10274328646));
#80341=CARTESIAN_POINT('',(4.35,-1.95899712601,5.10274328646));
#80342=CARTESIAN_POINT('',(2.3,-12.9053426461,5.10274328646));
#80343=CARTESIAN_POINT('',(3.225,-12.9053426461,5.10274328646));
#80344=CARTESIAN_POINT('',(2.3,-9.41827086707,5.10274328646));
#80345=CARTESIAN_POINT('',(2.3,-12.0504559477,5.10274328646));
#80346=CARTESIAN_POINT('',(3.69999999774,-9.41827086749,5.10274328646));
#80347=CARTESIAN_POINT('',(3.225,-9.41827086707,5.10274328646));
#80348=CARTESIAN_POINT('Ctrl Pts',(3.69999999774,-9.41827086749,5.10274328646));
#80349=CARTESIAN_POINT('Ctrl Pts',(3.73058948857333,-9.41827087355667,5.10274328646));
#80350=CARTESIAN_POINT('Ctrl Pts',(3.76117302676985,-9.41574705670535,5.10274328662896));
#80351=CARTESIAN_POINT('Ctrl Pts',(3.79135695696247,-9.41074020445563,5.10274328606016));
#80352=CARTESIAN_POINT('Ctrl Pts',(3.8215408871551,-9.40573335220591,5.10274328549136));
#80353=CARTESIAN_POINT('Ctrl Pts',(3.85132370712135,-9.39824319698092,5.10274328437385));
#80354=CARTESIAN_POINT('Ctrl Pts',(3.880310581398,-9.38836645220521,5.1027432782161));
#80355=CARTESIAN_POINT('Ctrl Pts',(3.90707199290093,-9.37924799297674,5.1027432725311));
#80356=CARTESIAN_POINT('Ctrl Pts',(3.93315644396342,-9.36809987699747,5.10274326252178));
#80357=CARTESIAN_POINT('Ctrl Pts',(3.95827561771127,-9.35505208010836,5.10274325269434));
#80358=CARTESIAN_POINT('Ctrl Pts',(3.98223829836866,-9.34260500707664,5.10274324331936));
#80359=CARTESIAN_POINT('Ctrl Pts',(4.00532196797495,-9.32842939224294,5.10274323477061));
#80360=CARTESIAN_POINT('Ctrl Pts',(4.02730698337273,-9.31267452069528,5.10274323470365));
#80361=CARTESIAN_POINT('Ctrl Pts',(4.0342532243783,-9.30769671500346,5.1027432346825));
#80362=CARTESIAN_POINT('Ctrl Pts',(4.04109006204254,-9.30256152719756,5.10274323548998));
#80363=CARTESIAN_POINT('Ctrl Pts',(4.04781138042469,-9.29727441845877,5.10274323721421));
#80364=CARTESIAN_POINT('Ctrl Pts',(4.06816544935236,-9.28126354535637,5.10274324243566));
#80365=CARTESIAN_POINT('Ctrl Pts',(4.08745353683921,-9.26386507535306,5.10274325797042));
#80366=CARTESIAN_POINT('Ctrl Pts',(4.1055168903408,-9.24523724841711,5.10274326872092));
#80367=CARTESIAN_POINT('Ctrl Pts',(4.12268030159011,-9.22753748661184,5.10274327893581));
#80368=CARTESIAN_POINT('Ctrl Pts',(4.13873762061326,-9.20872790766285,5.10274328434029));
#80369=CARTESIAN_POINT('Ctrl Pts',(4.1535845819758,-9.18897826222551,5.10274328574875));
#80370=CARTESIAN_POINT('Ctrl Pts',(4.16272152564545,-9.17682416594611,5.10274328661553));
#80371=CARTESIAN_POINT('Ctrl Pts',(4.17140072073273,-9.16431470638581,5.10274328646));
#80372=CARTESIAN_POINT('Ctrl Pts',(4.17960523291625,-9.15149611025241,5.10274328646));
#80373=CARTESIAN_POINT('Ctrl Pts',(4.18942766527051,-9.13614970201014,5.10274328646));
#80374=CARTESIAN_POINT('Ctrl Pts',(4.19857745049624,-9.12036311945856,5.10274328646));
#80375=CARTESIAN_POINT('Ctrl Pts',(4.20701878194007,-9.10419983822068,5.10274328646));
#80376=CARTESIAN_POINT('Ctrl Pts',(4.21621021747847,-9.08660027367622,5.10274328646));
#80377=CARTESIAN_POINT('Ctrl Pts',(4.22456152722091,-9.06855481897592,5.10274328646));
#80378=CARTESIAN_POINT('Ctrl Pts',(4.2320738661817,-9.05018712924208,5.10274328646));
#80379=CARTESIAN_POINT('Ctrl Pts',(4.23525034335279,-9.04242063368992,5.10274328646));
#80380=CARTESIAN_POINT('Ctrl Pts',(4.23827738137825,-9.03459693600601,5.10274328646));
#80381=CARTESIAN_POINT('Ctrl Pts',(4.24115737109239,-9.02672676812149,5.10274328646));
#80382=CARTESIAN_POINT('Ctrl Pts',(4.24909569801083,-9.00503364704426,5.10274328646));
#80383=CARTESIAN_POINT('Ctrl Pts',(4.25591706153315,-8.98297603570749,5.10274328646));
#80384=CARTESIAN_POINT('Ctrl Pts',(4.26171659160653,-8.96076940630961,5.10274328646));
#80385=CARTESIAN_POINT('Ctrl Pts',(4.26455589904718,-8.94989758613051,5.10274328646));
#80386=CARTESIAN_POINT('Ctrl Pts',(4.26715114281098,-8.93899011197066,5.10274328646));
#80387=CARTESIAN_POINT('Ctrl Pts',(4.26951780859379,-8.92807096217797,5.10274328646));
#80388=CARTESIAN_POINT('Ctrl Pts',(4.27382084868247,-8.90821790999222,5.10274328646));
#80389=CARTESIAN_POINT('Ctrl Pts',(4.27736537389317,-8.88833607622953,5.10274328652144));
#80390=CARTESIAN_POINT('Ctrl Pts',(4.28025710062774,-8.868557900564,5.10274328639925));
#80391=CARTESIAN_POINT('Ctrl Pts',(4.28203791090249,-8.85637791895645,5.102743286324));
#80392=CARTESIAN_POINT('Ctrl Pts',(4.2835716533847,-8.84423662612072,5.10274328620522));
#80393=CARTESIAN_POINT('Ctrl Pts',(4.2848866086288,-8.83215545542406,5.10274328535497));
#80394=CARTESIAN_POINT('Ctrl Pts',(4.28680275059482,-8.81455087285411,5.102743284116));
#80395=CARTESIAN_POINT('Ctrl Pts',(4.28827698219617,-8.79709218114212,5.10274328404483));
#80396=CARTESIAN_POINT('Ctrl Pts',(4.28939927179632,-8.77979151596189,5.10274328478464));
#80397=CARTESIAN_POINT('Ctrl Pts',(4.29044254900022,-8.76370886706949,5.10274328547236));
#80398=CARTESIAN_POINT('Ctrl Pts',(4.29118189695424,-8.74776302279939,5.10274328622038));
#80399=CARTESIAN_POINT('Ctrl Pts',(4.29168885063704,-8.73191886459746,5.1027432863823));
#80400=CARTESIAN_POINT('Ctrl Pts',(4.29196579590166,-8.72326331136879,5.10274328647075));
#80401=CARTESIAN_POINT('Ctrl Pts',(4.29217335586042,-8.71463728288328,5.10274328645986));
#80402=CARTESIAN_POINT('Ctrl Pts',(4.29232279496067,-8.70602836504273,5.10274328645976));
#80403=CARTESIAN_POINT('Ctrl Pts',(3.69999999774,-9.41827086749,5.10274328646));
#80404=CARTESIAN_POINT('Ctrl Pts',(3.69999999833,-9.34659890209,5.10274328646));
#80405=CARTESIAN_POINT('Ctrl Pts',(3.69999999892,-9.2749269367,5.0813396589));
#80406=CARTESIAN_POINT('Ctrl Pts',(3.69999999944,-9.21183540432,5.03842913842));
#80407=CARTESIAN_POINT('Ctrl Pts',(3.69999999982,-9.16559336719,4.97963577235));
#80408=CARTESIAN_POINT('Ctrl Pts',(3.70000000003,-9.13925764692,4.91297768617));
#80409=CARTESIAN_POINT('Ctrl Pts',(3.81412909821,-9.41827089013,5.10274328646));
#80410=CARTESIAN_POINT('Ctrl Pts',(3.79947056194,-9.34659892134,5.10274328643));
#80411=CARTESIAN_POINT('Ctrl Pts',(3.78481202566,-9.27492695255,5.08133965881));
#80412=CARTESIAN_POINT('Ctrl Pts',(3.77190837788,-9.21183541723,5.03842913824));
#80413=CARTESIAN_POINT('Ctrl Pts',(3.76245084042,-9.16559337792,4.97963577207));
#80414=CARTESIAN_POINT('Ctrl Pts',(3.75706459059,-9.13925765647,4.9129776858));
#80415=CARTESIAN_POINT('Ctrl Pts',(3.92823594404,-9.38909765086,5.10274328646));
#80416=CARTESIAN_POINT('Ctrl Pts',(3.89892199959,-9.32091627439,5.10274328539));
#80417=CARTESIAN_POINT('Ctrl Pts',(3.86960805513,-9.25273489792,5.08118011966));
#80418=CARTESIAN_POINT('Ctrl Pts',(3.84380320278,-9.19278171906,5.03794838538));
#80419=CARTESIAN_POINT('Ctrl Pts',(3.82488943837,-9.14898176867,4.97875813986));
#80420=CARTESIAN_POINT('Ctrl Pts',(3.81411802643,-9.12422889542,4.91173129034));
#80421=CARTESIAN_POINT('Ctrl Pts',(4.03302804821,-9.33107957038,5.10274328646));
#80422=CARTESIAN_POINT('Ctrl Pts',(3.99017706972,-9.2696193654,5.10274329028));
#80423=CARTESIAN_POINT('Ctrl Pts',(3.94732609124,-9.20815916043,5.08092237264));
#80424=CARTESIAN_POINT('Ctrl Pts',(3.90964076698,-9.15426319663,5.03717158458));
#80425=CARTESIAN_POINT('Ctrl Pts',(3.8820963349,-9.11520770945,4.97734162836));
#80426=CARTESIAN_POINT('Ctrl Pts',(3.86651403782,-9.0935734628,4.90972003087));
#80427=CARTESIAN_POINT('Ctrl Pts',(4.18747374061,-9.18016437508,5.10274328646));
#80428=CARTESIAN_POINT('Ctrl Pts',(4.12388018645,-9.13700016797,5.1027432833));
#80429=CARTESIAN_POINT('Ctrl Pts',(4.0602866323,-9.09383596087,5.07981408986));
#80430=CARTESIAN_POINT('Ctrl Pts',(4.00475631151,-9.05633061601,5.03383155537));
#80431=CARTESIAN_POINT('Ctrl Pts',(3.96503122609,-9.029900996,4.97125605817));
#80432=CARTESIAN_POINT('Ctrl Pts',(3.94373685893,-9.0162718551,4.90110872718));
#80433=CARTESIAN_POINT('Ctrl Pts',(4.26723541157,-8.98063713586,5.10274328646));
#80434=CARTESIAN_POINT('Ctrl Pts',(4.19077919927,-8.95915602901,5.10274328908));
#80435=CARTESIAN_POINT('Ctrl Pts',(4.11432298698,-8.93767492216,5.07732616962));
#80436=CARTESIAN_POINT('Ctrl Pts',(4.04869892936,-8.91937700045,5.02632575237));
#80437=CARTESIAN_POINT('Ctrl Pts',(4.00420277032,-8.90727654877,4.95775964986));
#80438=CARTESIAN_POINT('Ctrl Pts',(3.98361771521,-8.90210958415,4.88238701109));
#80439=CARTESIAN_POINT('Ctrl Pts',(4.28448738522,-8.88291546038,5.10274328646));
#80440=CARTESIAN_POINT('Ctrl Pts',(4.2038128468,-8.87211558957,5.10274328157));
#80441=CARTESIAN_POINT('Ctrl Pts',(4.12313830838,-8.86131571876,5.07547605456));
#80442=CARTESIAN_POINT('Ctrl Pts',(4.05474416619,-8.85231492765,5.02074277903));
#80443=CARTESIAN_POINT('Ctrl Pts',(4.01023278232,-8.84679291313,4.94775348423));
#80444=CARTESIAN_POINT('Ctrl Pts',(3.99224364397,-8.84501961539,4.86859296944));
#80445=CARTESIAN_POINT('Ctrl Pts',(4.2908008405,-8.79368075155,5.10274328646));
#80446=CARTESIAN_POINT('Ctrl Pts',(4.20683195096,-8.78806573108,5.10274328646));
#80447=CARTESIAN_POINT('Ctrl Pts',(4.12286306143,-8.78245071061,5.07330735934));
#80448=CARTESIAN_POINT('Ctrl Pts',(4.05279621082,-8.77777630692,5.01418352542));
#80449=CARTESIAN_POINT('Ctrl Pts',(4.00960658253,-8.77491887358,4.93631857882));
#80450=CARTESIAN_POINT('Ctrl Pts',(3.99540042025,-8.7740131878,4.85347142938));
#80451=CARTESIAN_POINT('Ctrl Pts',(4.29232317424,-8.70602837163,5.10274328646));
#80452=CARTESIAN_POINT('Ctrl Pts',(4.20764026079,-8.70455761115,5.10274328646));
#80453=CARTESIAN_POINT('Ctrl Pts',(4.12295734733,-8.70308685067,5.07285429077));
#80454=CARTESIAN_POINT('Ctrl Pts',(4.05251771609,-8.70186346543,5.01281324223));
#80455=CARTESIAN_POINT('Ctrl Pts',(4.00958636427,-8.70111783998,4.93392690561));
#80456=CARTESIAN_POINT('Ctrl Pts',(3.99616158712,-8.70088468041,4.85030226832));
#80457=CARTESIAN_POINT('Origin',(3.69999999356454,-9.41833116526676,4.80265463001755));
#80458=CARTESIAN_POINT('Origin',(3.,-8.67423561284,5.09670168568));
#80459=CARTESIAN_POINT('',(2.3,-9.13925764673,4.91297768617));
#80460=CARTESIAN_POINT('',(3.225,-9.13925764673,4.91297768617));
#80461=CARTESIAN_POINT('Origin',(2.3,-8.67423561284,5.09670168568));
#80462=CARTESIAN_POINT('Origin',(2.3,-9.17423561284,0.47366156039));
#80463=CARTESIAN_POINT('',(2.,-8.76025711822,4.30133994369));
#80464=CARTESIAN_POINT('',(2.,-8.76025711822,-3.35401682291));
#80465=CARTESIAN_POINT('Origin',(2.,-9.17423561284,0.47366156039));
#80466=CARTESIAN_POINT('Origin',(2.3,-8.76025711822,-3.35401682291));
#80467=CARTESIAN_POINT('Origin',(2.3,-8.76025711822,4.30133994369));
#80468=CARTESIAN_POINT('Origin',(3.,-8.67423561284,-4.1493785649));
#80469=CARTESIAN_POINT('Origin',(2.3,-8.67423561284,-4.1493785649));
#80470=CARTESIAN_POINT('Origin',(4.35,-8.31430322211,4.10274328646));
#80471=CARTESIAN_POINT('',(4.45,-8.31430322211,5.20274328646));
#80472=CARTESIAN_POINT('Origin',(4.45,-8.31430322211,4.10274328646));
#80473=CARTESIAN_POINT('Origin',(4.35,-8.31430322211,5.20274328646));
#80474=CARTESIAN_POINT('Origin',(4.45,0.,0.));
#80475=CARTESIAN_POINT('',(4.45,4.7773238354,-4.87121911588));
#80476=CARTESIAN_POINT('',(4.45,4.7773238354,-5.55542016568));
#80477=CARTESIAN_POINT('',(4.45,4.7773238354,0.294579834316));
#80478=CARTESIAN_POINT('',(4.45,4.9773238354,-4.67121911588));
#80479=CARTESIAN_POINT('Origin',(4.45,4.9773238354,-4.87121911588));
#80480=CARTESIAN_POINT('',(4.45,15.177455061,-4.67121911588));
#80481=CARTESIAN_POINT('',(4.45,-1.95899712601,-4.67121911588));
#80482=CARTESIAN_POINT('',(4.45,15.177455061,4.02878088412));
#80483=CARTESIAN_POINT('',(4.45,15.177455061,0.294579834316));
#80484=CARTESIAN_POINT('',(4.45,4.9773238354,4.02878088412));
#80485=CARTESIAN_POINT('',(4.45,-1.95899712601,4.02878088412));
#80486=CARTESIAN_POINT('',(4.45,4.7773238354,4.22878088412));
#80487=CARTESIAN_POINT('Origin',(4.45,4.9773238354,4.22878088412));
#80488=CARTESIAN_POINT('',(4.45,4.7773238354,5.90191320834));
#80489=CARTESIAN_POINT('',(4.45,4.7773238354,0.294579834316));
#80490=CARTESIAN_POINT('',(4.45,4.32269078618,5.90191320834));
#80491=CARTESIAN_POINT('',(4.45,-1.95899712601,5.90191320834));
#80492=CARTESIAN_POINT('',(4.45,2.97160656206,4.00332568658));
#80493=CARTESIAN_POINT('',(4.45,0.332366624557,0.294579834316));
#80494=CARTESIAN_POINT('',(4.45,2.48275227055,3.75120710557));
#80495=CARTESIAN_POINT('Origin',(4.45,2.48275227055,4.35120710557));
#80496=CARTESIAN_POINT('',(4.45,-2.24076213014,3.75120710557));
#80497=CARTESIAN_POINT('',(4.45,-1.95899712601,3.75120710557));
#80498=CARTESIAN_POINT('',(4.45,-2.49116133917,3.80595465384));
#80499=CARTESIAN_POINT('Origin',(4.45,-2.24076213014,4.35120710557));
#80500=CARTESIAN_POINT('',(4.45,-7.50411762961,6.1080814688));
#80501=CARTESIAN_POINT('',(4.45,4.59408048322,0.552161034916));
#80502=CARTESIAN_POINT('',(4.45,-7.67105043563,6.14457983432));
#80503=CARTESIAN_POINT('Origin',(4.45,-7.67105043563,5.74457983432));
#80504=CARTESIAN_POINT('',(4.45,-13.881029587,6.14457983432));
#80505=CARTESIAN_POINT('',(4.45,-1.95899712601,6.14457983432));
#80506=CARTESIAN_POINT('',(4.45,-14.4995104256,5.89840049188));
#80507=CARTESIAN_POINT('Origin',(4.45,-13.881029587,5.24457983432));
#80508=CARTESIAN_POINT('',(4.45,-18.4234397556,2.18656441774));
#80509=CARTESIAN_POINT('',(4.45,-18.85379408,1.77947127938));
#80510=CARTESIAN_POINT('',(4.45,-18.4689834555,1.96054363567));
#80511=CARTESIAN_POINT('Origin',(4.45,-18.2859995693,2.04127093829));
#80512=CARTESIAN_POINT('',(4.45,-18.3216303794,1.54889979527));
#80513=CARTESIAN_POINT('Origin',(4.45,-21.2594877202,0.729452270839));
#80514=CARTESIAN_POINT('',(4.45,-17.889478859,1.2973989265));
#80515=CARTESIAN_POINT('',(4.45,-13.9715079445,-0.982757551184));
#80516=CARTESIAN_POINT('',(4.45,-17.4134008589,1.35252791278));
#80517=CARTESIAN_POINT('Origin',(4.45,-17.6882812316,1.64311487169));
#80518=CARTESIAN_POINT('',(4.45,-13.661263671,4.90185742348));
#80519=CARTESIAN_POINT('',(4.45,-17.907928075,0.88473050722));
#80520=CARTESIAN_POINT('',(4.45,-12.9053426461,5.20274328646));
#80521=CARTESIAN_POINT('Origin',(4.45,-12.9053426461,4.10274328646));
#80522=CARTESIAN_POINT('',(4.45,-1.95899712601,5.20274328646));
#80523=CARTESIAN_POINT('',(4.45,-10.5397030792,-4.15378810588));
#80524=CARTESIAN_POINT('Origin',(4.45,-10.0779006799,-3.15542016568));
#80525=CARTESIAN_POINT('',(4.45,-17.3231001714,-1.01607812301));
#80526=CARTESIAN_POINT('',(4.45,-14.1190276664,-2.49814531564));
#80527=CARTESIAN_POINT('',(4.45,-17.582210652,-0.989652421484));
#80528=CARTESIAN_POINT('Origin',(4.45,-17.4910283166,-1.37912101035));
#80529=CARTESIAN_POINT('',(4.45,-19.0026826744,-1.32221314666));
#80530=CARTESIAN_POINT('',(4.45,-1.95899712601,2.6680522976));
#80531=CARTESIAN_POINT('',(4.45,-19.0409285996,-1.36351104187));
#80532=CARTESIAN_POINT('Origin',(4.45,-21.2594877202,0.729452270839));
#80533=CARTESIAN_POINT('',(4.45,-18.9794133856,-1.68227598146));
#80534=CARTESIAN_POINT('Origin',(4.45,-18.895449313,-1.50075453779));
#80535=CARTESIAN_POINT('',(4.45,-10.7858544195,-5.47226666221));
#80536=CARTESIAN_POINT('',(4.45,-15.667308925,-3.214314146));
#80537=CARTESIAN_POINT('',(4.45,-10.4080160928,-5.55542016568));
#80538=CARTESIAN_POINT('Origin',(4.45,-10.4080160928,-4.65542016568));
#80539=CARTESIAN_POINT('',(4.45,-1.95899712601,-5.55542016568));
#80540=CARTESIAN_POINT('Origin',(2.3,-9.41827086707,-3.85542016568));
#80541=CARTESIAN_POINT('Origin',(2.3,-9.41827086707,-3.85542016568));
#80542=CARTESIAN_POINT('Origin',(2.3,-21.2594877202,0.729452270839));
#80543=CARTESIAN_POINT('',(2.,-17.3209666442,-0.597405571358));
#80544=CARTESIAN_POINT('Origin',(2.3,-17.3209666442,-0.597405571358));
#80545=CARTESIAN_POINT('',(2.,-17.1183636721,1.08100826706));
#80546=CARTESIAN_POINT('Origin',(2.,-21.2594877202,0.729452270839));
#80547=CARTESIAN_POINT('Origin',(2.3,-17.1183636721,1.08100826706));
#80548=CARTESIAN_POINT('Origin',(2.,0.,0.));
#80549=CARTESIAN_POINT('',(2.,-17.1551720262,-0.653035235664));
#80550=CARTESIAN_POINT('Origin',(2.,-17.4910283166,-1.37912101035));
#80551=CARTESIAN_POINT('',(2.,-10.371774934,-3.79074521854));
#80552=CARTESIAN_POINT('',(2.,-13.7337583338,-2.23563518556));
#80553=CARTESIAN_POINT('Origin',(2.,-10.0779006799,-3.15542016568));
#80554=CARTESIAN_POINT('Origin',(2.,-8.67423561284,-4.1493785649));
#80555=CARTESIAN_POINT('',(2.,-9.41827086707,4.80274328646));
#80556=CARTESIAN_POINT('Origin',(2.,-8.67423561284,5.09670168568));
#80557=CARTESIAN_POINT('',(2.,-12.9053426461,4.80274328646));
#80558=CARTESIAN_POINT('',(2.,-12.0504559477,4.80274328646));
#80559=CARTESIAN_POINT('',(2.,-13.3863832983,4.61127046457));
#80560=CARTESIAN_POINT('Origin',(2.,-12.9053426461,4.10274328646));
#80561=CARTESIAN_POINT('',(2.,-16.3982789105,1.76217155265));
#80562=CARTESIAN_POINT('',(2.,-6.22423561284,0.47366156039));
#80563=CARTESIAN_POINT('Origin',(2.,-9.17423561284,0.47366156039));
#80564=CARTESIAN_POINT('Origin',(2.3,-10.0779006799,-3.15542016568));
#80565=CARTESIAN_POINT('Origin',(2.3,-10.371774934,-3.79074521854));
#80566=CARTESIAN_POINT('Origin',(0.,-10.2979776218,-4.15542016568));
#80567=CARTESIAN_POINT('',(2.3,-17.2811181351,-0.925317401172));
#80568=CARTESIAN_POINT('',(2.3,-13.8597044427,-2.50791735107));
#80569=CARTESIAN_POINT('',(4.35,-17.2811181351,-0.925317401172));
#80570=CARTESIAN_POINT('',(3.225,-17.2811181351,-0.925317401172));
#80571=CARTESIAN_POINT('',(4.35,-14.0770456301,-2.4073845938));
#80572=CARTESIAN_POINT('Origin',(4.35,-10.0779006799,-3.15542016568));
#80573=CARTESIAN_POINT('Origin',(4.35,-10.5397030792,-4.15378810588));
#80574=CARTESIAN_POINT('Origin',(2.3,-12.0504559477,4.80274328646));
#80575=CARTESIAN_POINT('Origin',(2.3,-9.41827086707,4.80274328646));
#80576=CARTESIAN_POINT('Origin',(2.3,-12.9053426461,4.80274328646));
#80577=CARTESIAN_POINT('Origin',(3.225,-9.41827086707,4.80274328646));
#80578=CARTESIAN_POINT('Origin',(2.3,-9.41827086707,4.80274328646));
#80579=CARTESIAN_POINT('Origin',(3.225,-12.9053426461,4.10274328646));
#80580=CARTESIAN_POINT('',(4.35,-13.5925435779,4.82921068375));
#80581=CARTESIAN_POINT('Origin',(4.35,-12.9053426461,4.10274328646));
#80582=CARTESIAN_POINT('',(2.3,-13.5925435779,4.82921068375));
#80583=CARTESIAN_POINT('',(3.325,-13.5925435779,4.82921068375));
#80584=CARTESIAN_POINT('Origin',(2.3,-12.9053426461,4.10274328646));
#80585=CARTESIAN_POINT('Origin',(4.35,-1.95899712601,5.20274328646));
#80586=CARTESIAN_POINT('Origin',(4.35,-12.9053426461,5.20274328646));
#80587=CARTESIAN_POINT('Origin',(2.3,-8.67423561284,5.09670168568));
#80588=CARTESIAN_POINT('Origin',(2.3,-9.41827086707,4.80274328646));
#80589=CARTESIAN_POINT('Origin',(2.3,-8.67423561284,-4.1493785649));
#80590=CARTESIAN_POINT('Origin',(4.35,-1.95899712601,-5.55542016568));
#80591=CARTESIAN_POINT('',(4.35,-10.4080160928,-5.65542016568));
#80592=CARTESIAN_POINT('Origin',(4.35,-10.4080160928,-5.55542016568));
#80593=CARTESIAN_POINT('',(4.35,4.8773238354,-5.65542016568));
#80594=CARTESIAN_POINT('',(4.35,-2.7653461287,-5.65542016568));
#80595=CARTESIAN_POINT('Origin',(4.35,4.7773238354,-5.55542016568));
#80596=CARTESIAN_POINT('Origin',(4.35,-10.4080160928,-4.65542016568));
#80597=CARTESIAN_POINT('',(4.35,-10.8278364558,-5.56302738404));
#80598=CARTESIAN_POINT('Origin',(4.35,-10.7858544195,-5.47226666221));
#80599=CARTESIAN_POINT('Origin',(4.35,-10.4080160928,-4.65542016568));
#80600=CARTESIAN_POINT('Origin',(4.35,-15.667308925,-3.214314146));
#80601=CARTESIAN_POINT('',(4.35,-19.0213954219,-1.7730367033));
#80602=CARTESIAN_POINT('Origin',(4.35,-18.9794133856,-1.68227598146));
#80603=CARTESIAN_POINT('',(4.35,-14.9246159388,-3.66803204367));
#80604=CARTESIAN_POINT('Origin',(4.35,-18.895449313,-1.50075453779));
#80605=CARTESIAN_POINT('',(4.35,-19.1136682429,-1.29488929392));
#80606=CARTESIAN_POINT('Origin',(4.35,-19.0409285996,-1.36351104187));
#80607=CARTESIAN_POINT('Origin',(4.35,-18.895449313,-1.50075453779));
#80608=CARTESIAN_POINT('Origin',(4.35,-21.2594877202,0.729452270839));
#80609=CARTESIAN_POINT('',(4.35,-19.0766762825,-1.25494542806));
#80610=CARTESIAN_POINT('Origin',(4.35,-19.0026826744,-1.32221314666));
#80611=CARTESIAN_POINT('Origin',(4.35,-21.2594877202,0.729452270839));
#80612=CARTESIAN_POINT('Origin',(4.35,-1.95899712601,2.6680522976));
#80613=CARTESIAN_POINT('',(4.35,-19.0254782583,-1.22484599945));
#80614=CARTESIAN_POINT('Origin',(4.35,-19.0026826744,-1.32221314666));
#80615=CARTESIAN_POINT('',(4.35,-17.6050062358,-0.892285274267));
#80616=CARTESIAN_POINT('Origin',(4.35,-17.582210652,-0.989652421484));
#80617=CARTESIAN_POINT('',(4.35,-18.246704933,-1.04251968981));
#80618=CARTESIAN_POINT('Origin',(4.35,-17.4910283166,-1.37912101035));
#80619=CARTESIAN_POINT('Origin',(4.35,-17.3231001714,-1.01607812301));
#80620=CARTESIAN_POINT('Origin',(4.35,-17.4910283166,-1.37912101035));
#80621=CARTESIAN_POINT('Origin',(4.35,-14.1190276664,-2.49814531564));
#80622=CARTESIAN_POINT('Origin',(4.35,-12.9053426461,4.10274328646));
#80623=CARTESIAN_POINT('Origin',(4.35,-13.661263671,4.90185742348));
#80624=CARTESIAN_POINT('Origin',(4.35,-17.907928075,0.88473050722));
#80625=CARTESIAN_POINT('',(4.35,-17.3446807657,1.27988117305));
#80626=CARTESIAN_POINT('Origin',(4.35,-17.4134008589,1.35252791278));
#80627=CARTESIAN_POINT('',(4.35,-15.4686121718,3.0545459284));
#80628=CARTESIAN_POINT('Origin',(4.35,-17.6882812316,1.64311487169));
#80629=CARTESIAN_POINT('',(4.35,-17.9397782658,1.2109699402));
#80630=CARTESIAN_POINT('Origin',(4.35,-17.889478859,1.2973989265));
#80631=CARTESIAN_POINT('Origin',(4.35,-17.6882812316,1.64311487169));
#80632=CARTESIAN_POINT('Origin',(4.35,-13.9715079445,-0.982757551184));
#80633=CARTESIAN_POINT('',(4.35,-18.3719297863,1.46247080897));
#80634=CARTESIAN_POINT('Origin',(4.35,-18.3216303794,1.54889979527));
#80635=CARTESIAN_POINT('',(4.35,-18.0119156597,1.25295201451));
#80636=CARTESIAN_POINT('Origin',(4.35,-21.2594877202,0.729452270839));
#80637=CARTESIAN_POINT('',(4.35,-18.4179535709,1.52203266332));
#80638=CARTESIAN_POINT('Origin',(4.35,-18.3216303794,1.54889979527));
#80639=CARTESIAN_POINT('',(4.35,-18.5604753986,1.92017998437));
#80640=CARTESIAN_POINT('Origin',(4.35,-18.4689834555,1.96054363567));
#80641=CARTESIAN_POINT('Origin',(4.35,-21.2594877202,0.729452270839));
#80642=CARTESIAN_POINT('Origin',(4.35,-18.2859995693,2.04127093829));
#80643=CARTESIAN_POINT('',(4.35,-18.4921598488,2.25921115747));
#80644=CARTESIAN_POINT('Origin',(4.35,-18.4234397556,2.18656441774));
#80645=CARTESIAN_POINT('Origin',(4.35,-18.2859995693,2.04127093829));
#80646=CARTESIAN_POINT('Origin',(4.35,-18.85379408,1.77947127938));
#80647=CARTESIAN_POINT('',(4.35,-14.5682305188,5.97104723161));
#80648=CARTESIAN_POINT('Origin',(4.35,-14.4995104256,5.89840049188));
#80649=CARTESIAN_POINT('',(4.35,-16.5301951838,4.11512919454));
#80650=CARTESIAN_POINT('Origin',(4.35,-13.881029587,5.24457983432));
#80651=CARTESIAN_POINT('',(4.35,-13.881029587,6.24457983432));
#80652=CARTESIAN_POINT('Origin',(4.35,-13.881029587,6.14457983432));
#80653=CARTESIAN_POINT('Origin',(4.35,-13.881029587,5.24457983432));
#80654=CARTESIAN_POINT('Origin',(4.35,-1.95899712601,6.14457983432));
#80655=CARTESIAN_POINT('',(4.35,-7.67105043563,6.24457983432));
#80656=CARTESIAN_POINT('Origin',(4.35,-7.67105043563,6.14457983432));
#80657=CARTESIAN_POINT('',(4.35,-10.7760400113,6.24457983432));
#80658=CARTESIAN_POINT('Origin',(4.35,-7.67105043563,5.74457983432));
#80659=CARTESIAN_POINT('',(4.35,-7.46238442811,6.19895687742));
#80660=CARTESIAN_POINT('Origin',(4.35,-7.50411762961,6.1080814688));
#80661=CARTESIAN_POINT('Origin',(4.35,-7.67105043563,5.74457983432));
#80662=CARTESIAN_POINT('Origin',(4.35,4.59408048322,0.552161034916));
#80663=CARTESIAN_POINT('',(4.35,-2.44942813767,3.89683006246));
#80664=CARTESIAN_POINT('Origin',(4.35,-2.49116133917,3.80595465384));
#80665=CARTESIAN_POINT('',(4.35,-4.95590628289,5.04789346994));
#80666=CARTESIAN_POINT('Origin',(4.35,-2.24076213014,4.35120710557));
#80667=CARTESIAN_POINT('',(4.35,-2.24076213014,3.85120710557));
#80668=CARTESIAN_POINT('Origin',(4.35,-2.24076213014,3.75120710557));
#80669=CARTESIAN_POINT('Origin',(4.35,-2.24076213014,4.35120710557));
#80670=CARTESIAN_POINT('Origin',(4.35,-1.95899712601,3.75120710557));
#80671=CARTESIAN_POINT('',(4.35,2.48275227055,3.85120710557));
#80672=CARTESIAN_POINT('Origin',(4.35,2.48275227055,3.75120710557));
#80673=CARTESIAN_POINT('',(4.35,0.120995070207,3.85120710557));
#80674=CARTESIAN_POINT('Origin',(4.35,2.48275227055,4.35120710557));
#80675=CARTESIAN_POINT('',(4.35,2.89013084681,4.06130592308));
#80676=CARTESIAN_POINT('Origin',(4.35,2.97160656206,4.00332568658));
#80677=CARTESIAN_POINT('Origin',(4.35,2.48275227055,4.35120710557));
#80678=CARTESIAN_POINT('Origin',(4.35,0.332366624557,0.294579834316));
#80679=CARTESIAN_POINT('',(4.35,4.24121507093,5.95989344484));
#80680=CARTESIAN_POINT('Origin',(4.35,4.32269078618,5.90191320834));
#80681=CARTESIAN_POINT('',(4.35,3.56567295887,5.01059968396));
#80682=CARTESIAN_POINT('Origin',(4.35,-1.95899712601,5.90191320834));
#80683=CARTESIAN_POINT('',(4.35,4.32269078618,6.00191320834));
#80684=CARTESIAN_POINT('Origin',(4.35,4.32269078618,5.90191320834));
#80685=CARTESIAN_POINT('',(4.35,4.7773238354,6.00191320834));
#80686=CARTESIAN_POINT('Origin',(4.35,4.7773238354,5.90191320834));
#80687=CARTESIAN_POINT('',(4.35,4.55000731079,6.00191320834));
#80688=CARTESIAN_POINT('Origin',(4.35,4.7773238354,0.294579834316));
#80689=CARTESIAN_POINT('',(4.35,4.8773238354,5.90191320834));
#80690=CARTESIAN_POINT('Origin',(4.35,4.7773238354,5.90191320834));
#80691=CARTESIAN_POINT('',(4.35,4.8773238354,4.22878088412));
#80692=CARTESIAN_POINT('Origin',(4.35,4.7773238354,4.22878088412));
#80693=CARTESIAN_POINT('',(4.35,4.8773238354,5.06534704623));
#80694=CARTESIAN_POINT('Origin',(4.35,4.9773238354,4.22878088412));
#80695=CARTESIAN_POINT('',(4.35,4.9773238354,4.12878088412));
#80696=CARTESIAN_POINT('Origin',(4.35,4.9773238354,4.02878088412));
#80697=CARTESIAN_POINT('Origin',(4.35,4.9773238354,4.22878088412));
#80698=CARTESIAN_POINT('Origin',(4.35,-1.95899712601,4.02878088412));
#80699=CARTESIAN_POINT('',(4.35,15.177455061,4.12878088412));
#80700=CARTESIAN_POINT('Origin',(4.35,15.177455061,4.02878088412));
#80701=CARTESIAN_POINT('',(4.35,10.0773894482,4.12878088412));
#80702=CARTESIAN_POINT('Origin',(4.35,15.177455061,0.294579834316));
#80703=CARTESIAN_POINT('',(4.35,15.277455061,4.02878088412));
#80704=CARTESIAN_POINT('Origin',(4.35,15.177455061,4.02878088412));
#80705=CARTESIAN_POINT('',(4.35,15.277455061,-4.67121911588));
#80706=CARTESIAN_POINT('Origin',(4.35,15.177455061,-4.67121911588));
#80707=CARTESIAN_POINT('',(4.35,15.277455061,-0.32121911588));
#80708=CARTESIAN_POINT('Origin',(4.35,-1.95899712601,-4.67121911588));
#80709=CARTESIAN_POINT('',(4.35,15.177455061,-4.77121911588));
#80710=CARTESIAN_POINT('Origin',(4.35,15.177455061,-4.67121911588));
#80711=CARTESIAN_POINT('',(4.35,4.9773238354,-4.77121911588));
#80712=CARTESIAN_POINT('Origin',(4.35,4.9773238354,-4.67121911588));
#80713=CARTESIAN_POINT('',(4.35,10.0773894482,-4.77121911588));
#80714=CARTESIAN_POINT('Origin',(4.35,4.9773238354,-4.87121911588));
#80715=CARTESIAN_POINT('',(4.35,4.8773238354,-4.87121911588));
#80716=CARTESIAN_POINT('Origin',(4.35,4.7773238354,-4.87121911588));
#80717=CARTESIAN_POINT('Origin',(4.35,4.9773238354,-4.87121911588));
#80718=CARTESIAN_POINT('Origin',(4.35,4.7773238354,0.294579834316));
#80719=CARTESIAN_POINT('',(4.35,4.8773238354,-5.26331964078));
#80720=CARTESIAN_POINT('Origin',(2.3,-9.17423561284,0.47366156039));
#80721=CARTESIAN_POINT('',(2.3,-6.52423561284,0.47366156039));
#80722=CARTESIAN_POINT('',(2.3,-11.82423561284,0.47366156039));
#80723=CARTESIAN_POINT('Origin',(2.3,-9.17423561284,0.47366156039));
#80724=CARTESIAN_POINT('Origin',(2.3,-9.17423561284,0.47366156039));
#80725=CARTESIAN_POINT('Origin',(2.3,-6.22423561284,0.473661560390001));
#80726=CARTESIAN_POINT('Origin',(2.3,-12.9053426461,4.10274328646));
#80727=CARTESIAN_POINT('Origin',(2.3,-13.3863832983,4.61127046457));
#80728=CARTESIAN_POINT('Origin',(3.94208066889,-21.2594877202,0.729452270839));
#80729=CARTESIAN_POINT('',(3.94208066889,-18.4179535709,1.52203266332));
#80730=CARTESIAN_POINT('Origin',(3.94208066889002,-18.7069231459878,1.44143126945959));
#80731=CARTESIAN_POINT('',(3.94208067709125,-18.560475400287,1.92017998362573));
#80732=CARTESIAN_POINT('Origin',(3.94208066889,-21.2594877202,0.729452270839));
#80733=CARTESIAN_POINT('Origin',(3.94208070435522,-18.8349512373474,1.79908900499315));
#80734=CARTESIAN_POINT('Origin',(-0.660000000086,-21.2594877202,0.729452270839));
#80735=CARTESIAN_POINT('',(2.225,-18.4179535709,1.52203266332));
#80736=CARTESIAN_POINT('',(2.225,-18.5604753986,1.92017998437));
#80737=CARTESIAN_POINT('Origin',(-3.94208066889,-21.2594877202,0.729452270839));
#80738=CARTESIAN_POINT('',(-3.94208066889,-18.5604753986,1.92017998437));
#80739=CARTESIAN_POINT('Origin',(-3.94208066888998,-18.8349512391587,1.79908905596751));
#80740=CARTESIAN_POINT('',(-3.94208069869828,-18.4179535709075,1.5220326633179));
#80741=CARTESIAN_POINT('Origin',(-3.94208066889,-21.2594877202,0.729452270839));
#80742=CARTESIAN_POINT('Origin',(-3.94208081057025,-18.7069232411033,1.44143132952455));
#80743=CARTESIAN_POINT('Origin',(-0.660000000086,-21.2594877202,0.729452270839));
#80744=CARTESIAN_POINT('',(-4.35,-18.5604753986,1.92017998437));
#80745=CARTESIAN_POINT('',(2.225,-18.5604753986,1.92017998437));
#80746=CARTESIAN_POINT('',(-4.35,-18.4179535709,1.52203266332));
#80747=CARTESIAN_POINT('Origin',(-4.35,-21.2594877202,0.729452270839));
#80748=CARTESIAN_POINT('',(-2.225,-18.4179535709,1.52203266332));
#80749=CARTESIAN_POINT('Origin',(3.94208066889,-21.2594877202,0.729452270839));
#80750=CARTESIAN_POINT('',(3.94208066889,-19.1136682429,-1.29488929392));
#80751=CARTESIAN_POINT('Origin',(3.94208066888998,-19.3318871727915,-1.089024050049));
#80752=CARTESIAN_POINT('',(3.94208068754125,-19.076676282417,-1.25494542798173));
#80753=CARTESIAN_POINT('Origin',(3.94208066889,-21.2594877202,0.729452270839));
#80754=CARTESIAN_POINT('Ctrl Pts',(3.69310716476821,-19.4224990726068,-0.940557363285379));
#80755=CARTESIAN_POINT('Ctrl Pts',(3.62071554431345,-19.3428165984805,-1.0129966546369));
#80756=CARTESIAN_POINT('Ctrl Pts',(3.60654669651459,-19.2341736857703,-1.11176422863347));
#80757=CARTESIAN_POINT('Ctrl Pts',(3.68256352205708,-19.1285867907532,-1.20775351544384));
#80758=CARTESIAN_POINT('Ctrl Pts',(3.81232210935313,-19.0766762800567,-1.25494542441243));
#80759=CARTESIAN_POINT('Ctrl Pts',(3.94208069665,-19.0766762825,-1.25494542806));
#80760=CARTESIAN_POINT('Origin',(-0.660000000086,-21.2594877202,0.729452270839));
#80761=CARTESIAN_POINT('',(2.225,-19.1136682429,-1.29488929392));
#80762=CARTESIAN_POINT('',(2.225,-19.0766762825,-1.25494542806));
#80763=CARTESIAN_POINT('Origin',(-3.94208066889,-21.2594877202,0.729452270839));
#80764=CARTESIAN_POINT('',(-3.94208066889,-19.0766762825,-1.25494542806));
#80765=CARTESIAN_POINT('Ctrl Pts',(-3.69310715294,-19.4224990402,-0.940557353778));
#80766=CARTESIAN_POINT('Ctrl Pts',(-3.66294397113573,-19.3892980535193,
-0.970740428832556));
#80767=CARTESIAN_POINT('Ctrl Pts',(-3.64523980863271,-19.3499675246131,
-1.00649588150467));
#80768=CARTESIAN_POINT('Ctrl Pts',(-3.63970736237874,-19.2700614290135,
-1.07913865288026));
#80769=CARTESIAN_POINT('Ctrl Pts',(-3.65188684851974,-19.229598084238,-1.1159239504417));
#80770=CARTESIAN_POINT('Ctrl Pts',(-3.70272651915015,-19.1589820790244,
-1.18012108438481));
#80771=CARTESIAN_POINT('Ctrl Pts',(-3.74131530326262,-19.1289285932923,
-1.20744276086762));
#80772=CARTESIAN_POINT('Ctrl Pts',(-3.834024439204,-19.087746776693,-1.24488122241778));
#80773=CARTESIAN_POINT('Ctrl Pts',(-3.88801458823712,-19.0766762824954,
-1.25494542806764));
#80774=CARTESIAN_POINT('Ctrl Pts',(-3.94208066889,-19.0766762825,-1.25494542806));
#80775=CARTESIAN_POINT('',(-3.94208067884,-19.1136682460366,-1.2948892935186));
#80776=CARTESIAN_POINT('Origin',(-3.94208066889,-21.2594877202,0.729452270839));
#80777=CARTESIAN_POINT('Origin',(-3.94208070251596,-19.3318871781364,-1.08902402959631));
#80778=CARTESIAN_POINT('Origin',(-0.660000000086,-21.2594877202,0.729452270839));
#80779=CARTESIAN_POINT('',(-4.35,-19.0766762825,-1.25494542806));
#80780=CARTESIAN_POINT('',(-2.225,-19.0766762825,-1.25494542806));
#80781=CARTESIAN_POINT('',(-4.35,-19.1136682429,-1.29488929392));
#80782=CARTESIAN_POINT('Origin',(-4.35,-21.2594877202,0.729452270839));
#80783=CARTESIAN_POINT('',(2.225,-19.1136682429,-1.29488929392));
#80784=CARTESIAN_POINT('Origin',(2.3,-17.1183636721,1.08100826706));
#80785=CARTESIAN_POINT('',(2.3,-17.3245239517,1.29894848625));
#80786=CARTESIAN_POINT('Origin',(2.3,-17.1183636721,1.08100826706));
#80787=CARTESIAN_POINT('Origin',(2.3,-17.1183636721,1.08100826706));
#80788=CARTESIAN_POINT('Origin',(2.3,-16.3982789105,1.76217155265));
#80789=CARTESIAN_POINT('',(2.3,-15.4585337648,3.064079585));
#80790=CARTESIAN_POINT('Origin',(2.3,-17.3209666442,-0.597405571358));
#80791=CARTESIAN_POINT('',(2.3,-17.3847397713,-0.890548860981));
#80792=CARTESIAN_POINT('Ctrl Pts',(2.15473698243741,-17.5697154200519,-0.5136040068197));
#80793=CARTESIAN_POINT('Ctrl Pts',(2.153925136701,-17.5747914639389,-0.530078530556508));
#80794=CARTESIAN_POINT('Ctrl Pts',(2.15383645219206,-17.5786293167837,-0.546970861777752));
#80795=CARTESIAN_POINT('Ctrl Pts',(2.15447419324571,-17.5811678664151,-0.56402768389419));
#80796=CARTESIAN_POINT('Ctrl Pts',(2.15512887051018,-17.5837738312011,-0.581537476590885));
#80797=CARTESIAN_POINT('Ctrl Pts',(2.15654900948215,-17.5850105747796,-0.599220153813188));
#80798=CARTESIAN_POINT('Ctrl Pts',(2.1587115129593,-17.5848603759444,-0.616799144345278));
#80799=CARTESIAN_POINT('Ctrl Pts',(2.16090081423076,-17.5847083158416,-0.634595974144406));
#80800=CARTESIAN_POINT('Ctrl Pts',(2.16385085219413,-17.5831348715607,-0.652286011369867));
#80801=CARTESIAN_POINT('Ctrl Pts',(2.167512339514,-17.5801692679682,-0.669587219172914));
#80802=CARTESIAN_POINT('Ctrl Pts',(2.17122230575012,-17.5771643991166,-0.687117498861475));
#80803=CARTESIAN_POINT('Ctrl Pts',(2.17566252859434,-17.5727304261426,-0.704248013442034));
#80804=CARTESIAN_POINT('Ctrl Pts',(2.18075816140222,-17.5669439862781,-0.720698733481176));
#80805=CARTESIAN_POINT('Ctrl Pts',(2.18420668827234,-17.5630279479552,-0.731831943472297));
#80806=CARTESIAN_POINT('Ctrl Pts',(2.18795490743752,-17.5584934329078,-0.742654087325353));
#80807=CARTESIAN_POINT('Ctrl Pts',(2.19197420126701,-17.5533753341438,-0.753083793143141));
#80808=CARTESIAN_POINT('Ctrl Pts',(2.19792273800431,-17.5458005710601,-0.768519710706872));
#80809=CARTESIAN_POINT('Ctrl Pts',(2.20446775346183,-17.5369433267012,-0.783099680208059));
#80810=CARTESIAN_POINT('Ctrl Pts',(2.21150225048338,-17.526947526872,-0.796581344453743));
#80811=CARTESIAN_POINT('Ctrl Pts',(2.21844404117408,-17.5170834598339,-0.809885336348122));
#80812=CARTESIAN_POINT('Ctrl Pts',(2.22586226006111,-17.5061109844372,-0.822119321309216));
#80813=CARTESIAN_POINT('Ctrl Pts',(2.23363909862176,-17.4942031712295,-0.833083573826689));
#80814=CARTESIAN_POINT('Ctrl Pts',(2.24132171377096,-17.482439631916,-0.843914984538571));
#80815=CARTESIAN_POINT('Ctrl Pts',(2.24935409459707,-17.4697635897432,-0.85350682681502));
#80816=CARTESIAN_POINT('Ctrl Pts',(2.2576112830013,-17.4563713159729,-0.861705619751016));
#80817=CARTESIAN_POINT('Ctrl Pts',(2.26568317060648,-17.4432795802197,-0.869720422349396));
#80818=CARTESIAN_POINT('Ctrl Pts',(2.27396968242377,-17.4295037165625,-0.876403714059283));
#80819=CARTESIAN_POINT('Ctrl Pts',(2.28234627169755,-17.4152507016175,-0.881654697950748));
#80820=CARTESIAN_POINT('Ctrl Pts',(2.28820169603079,-17.4052875235503,-0.885325253811452));
#80821=CARTESIAN_POINT('Ctrl Pts',(2.29410097189801,-17.3950916835449,-0.888296809376953));
#80822=CARTESIAN_POINT('Ctrl Pts',(2.3,-17.3847397713,-0.890548860981));
#80823=CARTESIAN_POINT('Origin',(2.3,-17.3209666442,-0.597405571358));
#80824=CARTESIAN_POINT('Origin',(2.3,-17.4910283166,-1.37912101035));
#80825=CARTESIAN_POINT('Origin',(2.3,-17.4910283166,-1.37912101035));
#80826=CARTESIAN_POINT('Origin',(2.3,-17.1551720262,-0.653035235664));
#80827=CARTESIAN_POINT('Origin',(2.3,-13.7337583338,-2.23563518556));
#80828=CARTESIAN_POINT('Ctrl Pts',(2.81682319433,-17.6050062023,-0.8922852285));
#80829=CARTESIAN_POINT('Ctrl Pts',(2.73612057106,-17.6939545409,-0.913109799));
#80830=CARTESIAN_POINT('Ctrl Pts',(2.65541794779,-17.7970156063,-0.873654435323));
#80831=CARTESIAN_POINT('Ctrl Pts',(2.60386284676,-17.8824681957,-0.76467039312));
#80832=CARTESIAN_POINT('Ctrl Pts',(2.60303393697,-17.9145456614,-0.631773538218));
#80833=CARTESIAN_POINT('Ctrl Pts',(2.6389185661,-17.8998831563,-0.516206719759));
#80834=CARTESIAN_POINT('Ctrl Pts',(2.72069356298,-17.5533276597,-0.880186363154));
#80835=CARTESIAN_POINT('Ctrl Pts',(2.6490925352,-17.6461138775,-0.891949880027));
#80836=CARTESIAN_POINT('Ctrl Pts',(2.57749150742,-17.7455086998,-0.846656393229));
#80837=CARTESIAN_POINT('Ctrl Pts',(2.52927175372,-17.8208769651,-0.739254396207));
#80838=CARTESIAN_POINT('Ctrl Pts',(2.52277338275,-17.8437268617,-0.610802571589));
#80839=CARTESIAN_POINT('Ctrl Pts',(2.54886029091,-17.8224196827,-0.498071213161));
#80840=CARTESIAN_POINT('Ctrl Pts',(2.61903613259,-17.5055395511,-0.876231590027));
#80841=CARTESIAN_POINT('Ctrl Pts',(2.55466919521,-17.5985472492,-0.878691004377));
#80842=CARTESIAN_POINT('Ctrl Pts',(2.49030225783,-17.6924862639,-0.828223972158));
#80843=CARTESIAN_POINT('Ctrl Pts',(2.44518237715,-17.7592388707,-0.723287859423));
#80844=CARTESIAN_POINT('Ctrl Pts',(2.43496771469,-17.7758070822,-0.600493912801));
#80845=CARTESIAN_POINT('Ctrl Pts',(2.45362336528,-17.7507876789,-0.492143392024));
#80846=CARTESIAN_POINT('Ctrl Pts',(2.51472500067,-17.4617307335,-0.877425549754));
#80847=CARTESIAN_POINT('Ctrl Pts',(2.45636381292,-17.5531913881,-0.871873917305));
#80848=CARTESIAN_POINT('Ctrl Pts',(2.39800262518,-17.6413431422,-0.817577061761));
#80849=CARTESIAN_POINT('Ctrl Pts',(2.35572686839,-17.7007047271,-0.715372409906));
#80850=CARTESIAN_POINT('Ctrl Pts',(2.34300336711,-17.7124820027,-0.59796369171));
#80851=CARTESIAN_POINT('Ctrl Pts',(2.35590021222,-17.685120806,-0.493932666461));
#80852=CARTESIAN_POINT('Ctrl Pts',(2.40817475382,-17.4215258268,-0.882546079144));
#80853=CARTESIAN_POINT('Ctrl Pts',(2.35497665859,-17.5103013085,-0.869969077284));
#80854=CARTESIAN_POINT('Ctrl Pts',(2.30177856336,-17.5925785463,-0.812746623601));
#80855=CARTESIAN_POINT('Ctrl Pts',(2.26216009393,-17.6454952576,-0.713450485069));
#80856=CARTESIAN_POINT('Ctrl Pts',(2.24774850121,-17.6535758491,-0.601299591245));
#80857=CARTESIAN_POINT('Ctrl Pts',(2.25607950621,-17.6248557047,-0.501608274656));
#80858=CARTESIAN_POINT('Ctrl Pts',(2.3,-17.3847397713,-0.890548860981));
#80859=CARTESIAN_POINT('Ctrl Pts',(2.25132255745,-17.4701614043,-0.871965441699));
#80860=CARTESIAN_POINT('Ctrl Pts',(2.20264511489,-17.5467153022,-0.812620072364));
#80861=CARTESIAN_POINT('Ctrl Pts',(2.16552232472,-17.5939868159,-0.716289768713));
#80862=CARTESIAN_POINT('Ctrl Pts',(2.15003006929,-17.5991454925,-0.609120539761));
#80863=CARTESIAN_POINT('Ctrl Pts',(2.15473684211,-17.5697153437,-0.51360402343));
#80864=CARTESIAN_POINT('Ctrl Pts',(2.3,-17.3847397713,-0.890548860981));
#80865=CARTESIAN_POINT('Ctrl Pts',(2.35860678773143,-17.4046696761071,-0.886213123483853));
#80866=CARTESIAN_POINT('Ctrl Pts',(2.41441920873521,-17.4250473814612,-0.883061314204722));
#80867=CARTESIAN_POINT('Ctrl Pts',(2.4674733429775,-17.4457070088102,-0.881183259835285));
#80868=CARTESIAN_POINT('Ctrl Pts',(2.52048805585001,-17.4663512852195,-0.879306600936282));
#80869=CARTESIAN_POINT('Ctrl Pts',(2.5707537492287,-17.4872788063911,-0.878699456805005));
#80870=CARTESIAN_POINT('Ctrl Pts',(2.61828660044749,-17.5083273649553,-0.879426979284592));
#80871=CARTESIAN_POINT('Ctrl Pts',(2.66936649605086,-17.5309466302949,-0.880208791680725));
#80872=CARTESIAN_POINT('Ctrl Pts',(2.71729027753892,-17.5537057811945,-0.882532787234766));
#80873=CARTESIAN_POINT('Ctrl Pts',(2.76201517433812,-17.5763925505084,-0.886462553872128));
#80874=CARTESIAN_POINT('Ctrl Pts',(2.78085443261086,-17.5859487918207,-0.888117871020545));
#80875=CARTESIAN_POINT('Ctrl Pts',(2.79912544466328,-17.5954920661211,-0.890057799537561));
#80876=CARTESIAN_POINT('Ctrl Pts',(2.81682316876698,-17.6050062304749,-0.8922852350963));
#80877=CARTESIAN_POINT('Origin',(3.225,-17.4910283166,-1.37912101035));
#80878=CARTESIAN_POINT('',(0.,-17.6050062358,-0.892285274267));
#80879=CARTESIAN_POINT('Origin',(2.3,-9.41827086707,4.80274328646));
#80880=CARTESIAN_POINT('Origin',(3.5527136788E-15,-19.4793690683,-1.15238185378));
#80881=CARTESIAN_POINT('',(2.33871339884049,-17.3446807699512,1.27988117280792));
#80882=CARTESIAN_POINT('Origin',(-7.3871464501E-14,-19.6855293478,-0.934441634591));
#80883=CARTESIAN_POINT('Origin',(2.33871339630113,-17.1385204882708,1.06194095191296));
#80884=CARTESIAN_POINT('Origin',(0.,-13.3033814002,5.10274328646));
#80885=CARTESIAN_POINT('',(3.225,-17.3446807657,1.27988117305));
#80886=CARTESIAN_POINT('Origin',(0.,4.8773238354,-5.65542016568));
#80887=CARTESIAN_POINT('',(-4.35,-10.4080160928,-5.65542016568));
#80888=CARTESIAN_POINT('',(2.225,-10.4080160928,-5.65542016568));
#80889=CARTESIAN_POINT('',(-4.35,4.8773238354,-5.65542016568));
#80890=CARTESIAN_POINT('',(-4.35,-1.95899712601,-5.65542016568));
#80891=CARTESIAN_POINT('',(0.,4.8773238354,-5.65542016568));
#80892=CARTESIAN_POINT('Origin',(2.225,-10.4080160928,-4.65542016568));
#80893=CARTESIAN_POINT('',(-4.35,-10.8278364558,-5.56302738404));
#80894=CARTESIAN_POINT('',(0.,-10.8278364558,-5.56302738404));
#80895=CARTESIAN_POINT('Origin',(-4.35,-10.4080160928,-4.65542016568));
#80896=CARTESIAN_POINT('Origin',(-7.89279752667E-12,-21.944500351,-0.751472579896));
#80897=CARTESIAN_POINT('',(-3.22521062834,-19.0213954219,-1.7730367033));
#80898=CARTESIAN_POINT('Origin',(-3.22521062833671,-19.1473415307962,-2.04531886881308));
#80899=CARTESIAN_POINT('',(3.22521062098,-19.021395423127,-1.77303669765361));
#80900=CARTESIAN_POINT('Origin',(1.8168799798E-13,-21.8185542421,-0.479190414391));
#80901=CARTESIAN_POINT('Origin',(3.22521057681892,-19.147341526537,-2.04531877209608));
#80902=CARTESIAN_POINT('Origin',(0.,-10.6280930347,-5.65542016568));
#80903=CARTESIAN_POINT('',(-4.35,-19.0213954219,-1.7730367033));
#80904=CARTESIAN_POINT('',(2.225,-19.0213954219,-1.7730367033));
#80905=CARTESIAN_POINT('',(-4.35,-15.7092909613,-3.30507486784));
#80906=CARTESIAN_POINT('',(2.225,-19.0213954219,-1.7730367033));
#80907=CARTESIAN_POINT('Ctrl Pts',(-3.94208068481,-19.1136682541,-1.29488929088));
#80908=CARTESIAN_POINT('Ctrl Pts',(-3.87720138886,-19.1136682521,-1.29488929001));
#80909=CARTESIAN_POINT('Ctrl Pts',(-3.81231526299,-19.1264162883,-1.28286293457));
#80910=CARTESIAN_POINT('Ctrl Pts',(-3.75378202546,-19.1519793642,-1.2587470166));
#80911=CARTESIAN_POINT('Ctrl Pts',(-3.66183898411,-19.2232952003,-1.1914684627));
#80912=CARTESIAN_POINT('Ctrl Pts',(-3.63176681562,-19.3185856291,-1.10157255296));
#80913=CARTESIAN_POINT('Ctrl Pts',(-3.63525640094,-19.3681821774,-1.0547837327));
#80914=CARTESIAN_POINT('Ctrl Pts',(-3.65691135058,-19.4144643621,-1.01112164612));
#80915=CARTESIAN_POINT('Ctrl Pts',(-3.69310716742,-19.4536303609,-0.974172889134));
#80916=CARTESIAN_POINT('Ctrl Pts',(-3.94208056753,-19.1696667267,-1.35424827581));
#80917=CARTESIAN_POINT('Ctrl Pts',(-3.87720126336,-19.159682392,-1.34366478855));
#80918=CARTESIAN_POINT('Ctrl Pts',(-3.81231512925,-19.1657164022,-1.32452150068));
#80919=CARTESIAN_POINT('Ctrl Pts',(-3.7537818851,-19.1888316549,-1.29781086364));
#80920=CARTESIAN_POINT('Ctrl Pts',(-3.66183883688,-19.2642991186,-1.23493306563));
#80921=CARTESIAN_POINT('Ctrl Pts',(-3.63176667561,-19.3794148126,-1.16605211769));
#80922=CARTESIAN_POINT('Ctrl Pts',(-3.63525626847,-19.4422756684,-1.13332358746));
#80923=CARTESIAN_POINT('Ctrl Pts',(-3.65691122872,-19.5037671225,-1.10578347233));
#80924=CARTESIAN_POINT('Ctrl Pts',(-3.69310705761,-19.5585539651,-1.08539296335));
#80925=CARTESIAN_POINT('Ctrl Pts',(-3.89367300212,-19.2061538294,-1.43589684659));
#80926=CARTESIAN_POINT('Ctrl Pts',(-3.83628934638,-19.1945998508,-1.40628312124));
#80927=CARTESIAN_POINT('Ctrl Pts',(-3.77890147363,-19.200140113,-1.37392209869));
#80928=CARTESIAN_POINT('Ctrl Pts',(-3.72658265001,-19.2238991299,-1.34173819539));
#80929=CARTESIAN_POINT('Ctrl Pts',(-3.64204616206,-19.3031632688,-1.28411031556));
#80930=CARTESIAN_POINT('Ctrl Pts',(-3.60813176427,-19.4272069341,-1.24772986945));
#80931=CARTESIAN_POINT('Ctrl Pts',(-3.60653309604,-19.4958412996,-1.23685475493));
#80932=CARTESIAN_POINT('Ctrl Pts',(-3.62053660286,-19.5643236317,-1.23399666395));
#80933=CARTESIAN_POINT('Ctrl Pts',(-3.64775681814,-19.6269188806,-1.23837648486));
#80934=CARTESIAN_POINT('Ctrl Pts',(-3.80930230156,-19.2045641287,-1.50795234761));
#80935=CARTESIAN_POINT('Ctrl Pts',(-3.75987784682,-19.2054688076,-1.4752752232));
#80936=CARTESIAN_POINT('Ctrl Pts',(-3.71045096623,-19.2208549013,-1.44349482057));
#80937=CARTESIAN_POINT('Ctrl Pts',(-3.66483648247,-19.250546929,-1.41519005469));
#80938=CARTESIAN_POINT('Ctrl Pts',(-3.58875746632,-19.3333975541,-1.37014271634));
#80939=CARTESIAN_POINT('Ctrl Pts',(-3.5517176612,-19.4476835822,-1.35267289918));
#80940=CARTESIAN_POINT('Ctrl Pts',(-3.54520036865,-19.5088551603,-1.35199065903));
#80941=CARTESIAN_POINT('Ctrl Pts',(-3.55129886954,-19.5690125364,-1.35930367043));
#80942=CARTESIAN_POINT('Ctrl Pts',(-3.56871476432,-19.6239406117,-1.37338573889));
#80943=CARTESIAN_POINT('Ctrl Pts',(-3.64606474778,-19.1826736184,-1.62180070384));
#80944=CARTESIAN_POINT('Ctrl Pts',(-3.60648671327,-19.1958948229,-1.58929946191));
#80945=CARTESIAN_POINT('Ctrl Pts',(-3.56690777206,-19.2195650029,-1.56181889209));
#80946=CARTESIAN_POINT('Ctrl Pts',(-3.52971312193,-19.2528311608,-1.5413518596));
#80947=CARTESIAN_POINT('Ctrl Pts',(-3.46482449341,-19.3342203712,-1.5169589309));
#80948=CARTESIAN_POINT('Ctrl Pts',(-3.42528173585,-19.4342377637,-1.52616144186));
#80949=CARTESIAN_POINT('Ctrl Pts',(-3.41345573834,-19.4861495298,-1.53932474796));
#80950=CARTESIAN_POINT('Ctrl Pts',(-3.41038172025,-19.5366455777,-1.56008532149));
#80951=CARTESIAN_POINT('Ctrl Pts',(-3.41578699493,-19.5829245944,-1.58670170918));
#80952=CARTESIAN_POINT('Ctrl Pts',(-3.4671692423,-19.1242637155,-1.70186764332));
#80953=CARTESIAN_POINT('Ctrl Pts',(-3.43450859846,-19.1460253867,-1.67828450814));
#80954=CARTESIAN_POINT('Ctrl Pts',(-3.40184766079,-19.1740199682,-1.6606153876));
#80955=CARTESIAN_POINT('Ctrl Pts',(-3.37068117107,-19.2071483267,-1.64991354979));
#80956=CARTESIAN_POINT('Ctrl Pts',(-3.31431449303,-19.2803854864,-1.64335673091));
#80957=CARTESIAN_POINT('Ctrl Pts',(-3.27435380127,-19.3605444526,-1.6655744582));
#80958=CARTESIAN_POINT('Ctrl Pts',(-3.2596011797,-19.4005949558,-1.68366210416));
#80959=CARTESIAN_POINT('Ctrl Pts',(-3.25082353853,-19.4387529418,-1.70783034438));
#80960=CARTESIAN_POINT('Ctrl Pts',(-3.24819011402,-19.473482982,-1.73672177881));
#80961=CARTESIAN_POINT('Ctrl Pts',(-3.38547751269,-19.0935072946,-1.73183570145));
#80962=CARTESIAN_POINT('Ctrl Pts',(-3.35512154584,-19.1165078816,-1.71264403289));
#80963=CARTESIAN_POINT('Ctrl Pts',(-3.32476535702,-19.1442415397,-1.69929570405));
#80964=CARTESIAN_POINT('Ctrl Pts',(-3.29564414506,-19.1757570958,-1.69255186303));
#80965=CARTESIAN_POINT('Ctrl Pts',(-3.24233287408,-19.2436848784,-1.6927859443));
#80966=CARTESIAN_POINT('Ctrl Pts',(-3.20268173876,-19.3157439579,-1.71926217841));
#80967=CARTESIAN_POINT('Ctrl Pts',(-3.18722650592,-19.3513922741,-1.73877210954));
#80968=CARTESIAN_POINT('Ctrl Pts',(-3.17680955904,-19.3851723952,-1.76371055191));
#80969=CARTESIAN_POINT('Ctrl Pts',(-3.17165790098,-19.4158555881,-1.79287228805));
#80970=CARTESIAN_POINT('Ctrl Pts',(-3.30422173516,-19.0589182003,-1.75568026745));
#80971=CARTESIAN_POINT('Ctrl Pts',(-3.27596559888,-19.0824576484,-1.74095218972));
#80972=CARTESIAN_POINT('Ctrl Pts',(-3.24770931985,-19.1094046865,-1.73175819756));
#80973=CARTESIAN_POINT('Ctrl Pts',(-3.22045811805,-19.1389197877,-1.72861076563));
#80974=CARTESIAN_POINT('Ctrl Pts',(-3.16997041597,-19.2009235168,-1.73461137249));
#80975=CARTESIAN_POINT('Ctrl Pts',(-3.13070946984,-19.2644437842,-1.7638921058));
#80976=CARTESIAN_POINT('Ctrl Pts',(-3.11468881656,-19.2954758049,-1.78403275906));
#80977=CARTESIAN_POINT('Ctrl Pts',(-3.10287409283,-19.3246516908,-1.80892678684));
#80978=CARTESIAN_POINT('Ctrl Pts',(-3.09553404662,-19.351046075,-1.83754968546));
#80979=CARTESIAN_POINT('Ctrl Pts',(-3.22521062834,-19.0213954219,-1.7730367033));
#80980=CARTESIAN_POINT('Ctrl Pts',(-3.19874622208,-19.044347457,-1.76242007146));
#80981=CARTESIAN_POINT('Ctrl Pts',(-3.17228172271,-19.0696431519,-1.75686997245));
#80982=CARTESIAN_POINT('Ctrl Pts',(-3.14663842378,-19.096571511,-1.75671868196));
#80983=CARTESIAN_POINT('Ctrl Pts',(-3.09863298495,-19.1519725754,-1.76722316791));
#80984=CARTESIAN_POINT('Ctrl Pts',(-3.05987676099,-19.2070352425,-1.79804851641));
#80985=CARTESIAN_POINT('Ctrl Pts',(-3.04348517182,-19.2336251131,-1.81822356982));
#80986=CARTESIAN_POINT('Ctrl Pts',(-3.03060394682,-19.2584238423,-1.84251642021));
#80987=CARTESIAN_POINT('Ctrl Pts',(-3.02151311497,-19.2807402375,-1.87007016525));
#80988=CARTESIAN_POINT('Ctrl Pts',(-3.22521062834,-19.0213954219,-1.7730367033));
#80989=CARTESIAN_POINT('Ctrl Pts',(-3.24772444597292,-19.0320873489464,
-1.76809107416998));
#80990=CARTESIAN_POINT('Ctrl Pts',(-3.27028135195154,-19.0424883596232,
-1.76251507821921));
#80991=CARTESIAN_POINT('Ctrl Pts',(-3.2928662202311,-19.0525235172448,-1.75634535752002));
#80992=CARTESIAN_POINT('Ctrl Pts',(-3.30614125710113,-19.0584220279545,
-1.75271889095197));
#80993=CARTESIAN_POINT('Ctrl Pts',(-3.31942721657902,-19.064194344846,-1.74888731162803));
#80994=CARTESIAN_POINT('Ctrl Pts',(-3.33272883036821,-19.0698263727899,
-1.74485946562232));
#80995=CARTESIAN_POINT('Ctrl Pts',(-3.35069467910696,-19.0774332815256,
-1.73941924812477));
#80996=CARTESIAN_POINT('Ctrl Pts',(-3.36868359493464,-19.0847837961097,
-1.7336209772335));
#80997=CARTESIAN_POINT('Ctrl Pts',(-3.38669558519312,-19.0918460227535,
-1.72749125982607));
#80998=CARTESIAN_POINT('Ctrl Pts',(-3.39570158032236,-19.0953771360754,
-1.72442640112235));
#80999=CARTESIAN_POINT('Ctrl Pts',(-3.40431105974672,-19.0986840050788,
-1.72141745792359));
#81000=CARTESIAN_POINT('Ctrl Pts',(-3.41311378877424,-19.1020038683847,
-1.71825795819223));
#81001=CARTESIAN_POINT('Ctrl Pts',(-3.42128496560172,-19.1050855479446,
-1.71532513691481));
#81002=CARTESIAN_POINT('Ctrl Pts',(-3.4296228773541,-19.1081784742,-1.71226240285957));
#81003=CARTESIAN_POINT('Ctrl Pts',(-3.43860354554371,-19.111447523279,-1.70886309082487));
#81004=CARTESIAN_POINT('Ctrl Pts',(-3.43929766352361,-19.1117001888596,
-1.70860035718938));
#81005=CARTESIAN_POINT('Ctrl Pts',(-3.43999562251229,-19.1119538925657,
-1.70833559083555));
#81006=CARTESIAN_POINT('Ctrl Pts',(-3.44069764286074,-19.1122087031213,
-1.70806868482413));
#81007=CARTESIAN_POINT('Ctrl Pts',(-3.4661961713137,-19.1214638396967,-1.69837422149201));
#81008=CARTESIAN_POINT('Ctrl Pts',(-3.49111096758992,-19.130046569157,-1.68809291431738));
#81009=CARTESIAN_POINT('Ctrl Pts',(-3.51542366771508,-19.1379196799265,
-1.67729049519577));
#81010=CARTESIAN_POINT('Ctrl Pts',(-3.52843047035992,-19.1421316348904,
-1.67151141953251));
#81011=CARTESIAN_POINT('Ctrl Pts',(-3.5412644137341,-19.1461398298069,-1.66558344175602));
#81012=CARTESIAN_POINT('Ctrl Pts',(-3.55391844673925,-19.1499344256496,
-1.65951839712039));
#81013=CARTESIAN_POINT('Ctrl Pts',(-3.57553475391646,-19.1564165605797,
-1.64915775811827));
#81014=CARTESIAN_POINT('Ctrl Pts',(-3.59663453427806,-19.1622797228512,
-1.63839506557308));
#81015=CARTESIAN_POINT('Ctrl Pts',(-3.6171612881736,-19.1674726055405,-1.62725042901185));
#81016=CARTESIAN_POINT('Ctrl Pts',(-3.62193563094114,-19.1686804244698,
-1.62465828437789));
#81017=CARTESIAN_POINT('Ctrl Pts',(-3.62667885762862,-19.1698518313957,
-1.62204542253218));
#81018=CARTESIAN_POINT('Ctrl Pts',(-3.63138996488376,-19.1709858783566,
-1.61941203301298));
#81019=CARTESIAN_POINT('Ctrl Pts',(-3.63591728936824,-19.1720756855493,
-1.61688137340329));
#81020=CARTESIAN_POINT('Ctrl Pts',(-3.64041501866186,-19.1731310191457,
-1.61433172446812));
#81021=CARTESIAN_POINT('Ctrl Pts',(-3.64488244879203,-19.1741521328984,
-1.61176395184423));
#81022=CARTESIAN_POINT('Ctrl Pts',(-3.64540287798236,-19.1742710866118,
-1.61146482151904));
#81023=CARTESIAN_POINT('Ctrl Pts',(-3.64592666721413,-19.1743904272115,
-1.61116326385945));
#81024=CARTESIAN_POINT('Ctrl Pts',(-3.64643164572595,-19.1745051343925,
-1.61087208357338));
#81025=CARTESIAN_POINT('Ctrl Pts',(-3.64916151036296,-19.1751252302375,
-1.60929799131533));
#81026=CARTESIAN_POINT('Ctrl Pts',(-3.65147817017146,-19.1756436403,-1.60795197344029));
#81027=CARTESIAN_POINT('Ctrl Pts',(-3.65436417184066,-19.1762780377711,
-1.60626030924236));
#81028=CARTESIAN_POINT('Ctrl Pts',(-3.6555270412225,-19.1765336583422,-1.60557867952568));
#81029=CARTESIAN_POINT('Ctrl Pts',(-3.65678220408794,-19.1768077686339,
-1.60484061205229));
#81030=CARTESIAN_POINT('Ctrl Pts',(-3.6581932018563,-19.1771128584525,-1.60400694268519));
#81031=CARTESIAN_POINT('Ctrl Pts',(-3.6742877471575,-19.1805928653082,-1.59449769348881));
#81032=CARTESIAN_POINT('Ctrl Pts',(-3.68966114213862,-19.1835569868908,
-1.58492691989271));
#81033=CARTESIAN_POINT('Ctrl Pts',(-3.70433248725225,-19.1860351129862,
-1.57533948257634));
#81034=CARTESIAN_POINT('Ctrl Pts',(-3.72775122383417,-19.1899907545306,
-1.56003579588171));
#81035=CARTESIAN_POINT('Ctrl Pts',(-3.74937546375535,-19.1927024574446,
-1.54469005867433));
#81036=CARTESIAN_POINT('Ctrl Pts',(-3.76916732977652,-19.1942216676716,
-1.52951153228472));
#81037=CARTESIAN_POINT('Ctrl Pts',(-3.78526285634382,-19.1954571493864,
-1.51716775557892));
#81038=CARTESIAN_POINT('Ctrl Pts',(-3.80015850434429,-19.1959035366658,
-1.50492975762664));
#81039=CARTESIAN_POINT('Ctrl Pts',(-3.81385444633577,-19.1956091287661,
-1.49289560584265));
#81040=CARTESIAN_POINT('Ctrl Pts',(-3.82070241733151,-19.1954619248163,
-1.48687852995065));
#81041=CARTESIAN_POINT('Ctrl Pts',(-3.82725045890622,-19.1951299577511,
-1.48091230974744));
#81042=CARTESIAN_POINT('Ctrl Pts',(-3.83349856779365,-19.1946218274872,
-1.47500806817809));
#81043=CARTESIAN_POINT('Ctrl Pts',(-3.83662262223736,-19.1943677623552,
-1.47205594739341));
#81044=CARTESIAN_POINT('Ctrl Pts',(-3.83967169317361,-19.1940696838623,
-1.4691193204789));
#81045=CARTESIAN_POINT('Ctrl Pts',(-3.84264577876859,-19.1937288068363,
-1.46619944749653));
#81046=CARTESIAN_POINT('Ctrl Pts',(-3.84427530786577,-19.1935420371504,
-1.46459962199289));
#81047=CARTESIAN_POINT('Ctrl Pts',(-3.84558853566292,-19.1933790227199,
-1.46329651293835));
#81048=CARTESIAN_POINT('Ctrl Pts',(-3.84707135142737,-19.1931828234745,
-1.46181166623411));
#81049=CARTESIAN_POINT('Ctrl Pts',(-3.84829485186967,-19.1930209356195,
-1.46058649002345));
#81050=CARTESIAN_POINT('Ctrl Pts',(-3.84963382677702,-19.192836412323,-1.45923751109255));
#81051=CARTESIAN_POINT('Ctrl Pts',(-3.85134307689286,-19.1925790828302,
-1.45749132327324));
#81052=CARTESIAN_POINT('Ctrl Pts',(-3.86750161951162,-19.1901463963916,
-1.44098358690551));
#81053=CARTESIAN_POINT('Ctrl Pts',(-3.88146163353687,-19.1863177603114,
-1.42482655476048));
#81054=CARTESIAN_POINT('Ctrl Pts',(-3.8932591846746,-19.1812263066711,-1.40917519080981));
#81055=CARTESIAN_POINT('Ctrl Pts',(-3.90503537655242,-19.1761440710185,
-1.39355216337972));
#81056=CARTESIAN_POINT('Ctrl Pts',(-3.91466188565638,-19.1698056445851,
-1.37843033478599));
#81057=CARTESIAN_POINT('Ctrl Pts',(-3.9221775305533,-19.1623488557789,-1.36395201741712));
#81058=CARTESIAN_POINT('Ctrl Pts',(-3.92828814640728,-19.1562860930322,
-1.35218038146748));
#81059=CARTESIAN_POINT('Ctrl Pts',(-3.93300430884911,-19.1494837461493,
-1.34083267762417));
#81060=CARTESIAN_POINT('Ctrl Pts',(-3.93631580667821,-19.1420117931894,
-1.33000380907411));
#81061=CARTESIAN_POINT('Ctrl Pts',(-3.93919658915514,-19.1355116919464,
-1.320583414928));
#81062=CARTESIAN_POINT('Ctrl Pts',(-3.94101431043189,-19.1285042561885,
-1.31155499950984));
#81063=CARTESIAN_POINT('Ctrl Pts',(-3.94173213759005,-19.1210385047908,
-1.30300892857622));
#81064=CARTESIAN_POINT('Ctrl Pts',(-3.94196382899028,-19.1186288015978,
-1.30025053316233));
#81065=CARTESIAN_POINT('Ctrl Pts',(-3.9420806794518,-19.1161714145093,-1.29754266791182));
#81066=CARTESIAN_POINT('Ctrl Pts',(-3.94208068480999,-19.1136682541,-1.29488929088));
#81067=CARTESIAN_POINT('Origin',(2.225,-18.895449313,-1.50075453779));
#81068=CARTESIAN_POINT('Origin',(-4.35,-18.895449313,-1.50075453779));
#81069=CARTESIAN_POINT('Ctrl Pts',(3.22521062098,-19.0213954214,-1.77303668325));
#81070=CARTESIAN_POINT('Ctrl Pts',(3.19874621439,-19.0443474533,-1.7624200523));
#81071=CARTESIAN_POINT('Ctrl Pts',(3.1722817147,-19.0696431447,-1.75686995397));
#81072=CARTESIAN_POINT('Ctrl Pts',(3.14663841544,-19.0965715001,-1.75671866391));
#81073=CARTESIAN_POINT('Ctrl Pts',(3.09863297604,-19.1519725569,-1.76722315022));
#81074=CARTESIAN_POINT('Ctrl Pts',(3.05987675166,-19.2070352164,-1.79804849807));
#81075=CARTESIAN_POINT('Ctrl Pts',(3.04348516232,-19.2336250834,-1.81822355091));
#81076=CARTESIAN_POINT('Ctrl Pts',(3.03060393721,-19.2584238091,-1.84251640048));
#81077=CARTESIAN_POINT('Ctrl Pts',(3.0215131053,-19.2807402012,-1.87007014451));
#81078=CARTESIAN_POINT('Ctrl Pts',(3.31887229845,-19.0658758373,-1.75246199623));
#81079=CARTESIAN_POINT('Ctrl Pts',(3.29028393291,-19.089524209,-1.73697155779));
#81080=CARTESIAN_POINT('Ctrl Pts',(3.2616954154,-19.1167774494,-1.72710190069));
#81081=CARTESIAN_POINT('Ctrl Pts',(3.23414607027,-19.1467721985,-1.72339891277));
#81082=CARTESIAN_POINT('Ctrl Pts',(3.18319809785,-19.2100002284,-1.72856439386));
#81083=CARTESIAN_POINT('Ctrl Pts',(3.14384356469,-19.2750887468,-1.75755872073));
#81084=CARTESIAN_POINT('Ctrl Pts',(3.12789169205,-19.3069444531,-1.77769299668));
#81085=CARTESIAN_POINT('Ctrl Pts',(3.11627472338,-19.3369319732,-1.80269849863));
#81086=CARTESIAN_POINT('Ctrl Pts',(3.10925931489,-19.3640825186,-1.83151964554));
#81087=CARTESIAN_POINT('Ctrl Pts',(3.41573924533,-19.1062581898,-1.72274306856));
#81088=CARTESIAN_POINT('Ctrl Pts',(3.38458474557,-19.1289876528,-1.70187932147));
#81089=CARTESIAN_POINT('Ctrl Pts',(3.3534299924,-19.1569566778,-1.68696468886));
#81090=CARTESIAN_POINT('Ctrl Pts',(3.32359852403,-19.1891775057,-1.67885768802));
#81091=CARTESIAN_POINT('Ctrl Pts',(3.26921872731,-19.2592689985,-1.67689652144));
#81092=CARTESIAN_POINT('Ctrl Pts',(3.22943107032,-19.334526867,-1.70228745871));
#81093=CARTESIAN_POINT('Ctrl Pts',(3.21419840626,-19.3719160959,-1.72154573558));
#81094=CARTESIAN_POINT('Ctrl Pts',(3.20432114725,-19.4074383872,-1.74648676951));
#81095=CARTESIAN_POINT('Ctrl Pts',(3.20000833496,-19.4397458552,-1.77583596615));
#81096=CARTESIAN_POINT('Ctrl Pts',(3.51291896248,-19.1413289289,-1.68469422833));
#81097=CARTESIAN_POINT('Ctrl Pts',(3.4789462662,-19.1620682059,-1.65842751755));
#81098=CARTESIAN_POINT('Ctrl Pts',(3.44497324706,-19.1899424465,-1.63811566301));
#81099=CARTESIAN_POINT('Ctrl Pts',(3.41264252321,-19.2237987455,-1.62501908412));
#81100=CARTESIAN_POINT('Ctrl Pts',(3.35453777244,-19.2998586458,-1.61444987467));
#81101=CARTESIAN_POINT('Ctrl Pts',(3.31440978178,-19.3847471634,-1.63435949598));
#81102=CARTESIAN_POINT('Ctrl Pts',(3.30006468822,-19.4274328561,-1.65176034228));
#81103=CARTESIAN_POINT('Ctrl Pts',(3.2922329623,-19.4682507262,-1.67564817155));
#81104=CARTESIAN_POINT('Ctrl Pts',(3.29105041121,-19.5054576982,-1.70454430458));
#81105=CARTESIAN_POINT('Ctrl Pts',(3.69283515033,-19.1942585079,-1.59547606027));
#81106=CARTESIAN_POINT('Ctrl Pts',(3.65105292983,-19.2042463076,-1.56116545001));
#81107=CARTESIAN_POINT('Ctrl Pts',(3.60926958339,-19.2259574623,-1.5312745857));
#81108=CARTESIAN_POINT('Ctrl Pts',(3.57016835315,-19.258655952,-1.50808432834));
#81109=CARTESIAN_POINT('Ctrl Pts',(3.50264897247,-19.341385442,-1.47818397612));
#81110=CARTESIAN_POINT('Ctrl Pts',(3.46343047149,-19.446443377,-1.48240833377));
#81111=CARTESIAN_POINT('Ctrl Pts',(3.45265831019,-19.501492664,-1.49338380489));
#81112=CARTESIAN_POINT('Ctrl Pts',(3.45153181921,-19.5552861337,-1.51230581401));
#81113=CARTESIAN_POINT('Ctrl Pts',(3.4596034448,-19.6046311185,-1.53737756014));
#81114=CARTESIAN_POINT('Ctrl Pts',(3.84656205857,-19.2016706385,-1.47236182198));
#81115=CARTESIAN_POINT('Ctrl Pts',(3.79361941084,-19.1984204408,-1.44241491043));
#81116=CARTESIAN_POINT('Ctrl Pts',(3.74067352441,-19.2105079959,-1.41147096078));
#81117=CARTESIAN_POINT('Ctrl Pts',(3.69209672656,-19.2381656965,-1.38207884));
#81118=CARTESIAN_POINT('Ctrl Pts',(3.61228551508,-19.3195355041,-1.33161378879));
#81119=CARTESIAN_POINT('Ctrl Pts',(3.57663385678,-19.4363429733,-1.30393743154));
#81120=CARTESIAN_POINT('Ctrl Pts',(3.57229261138,-19.4994985456,-1.29737816529));
#81121=CARTESIAN_POINT('Ctrl Pts',(3.58188180677,-19.5617860447,-1.29857025048));
#81122=CARTESIAN_POINT('Ctrl Pts',(3.60362130644,-19.6185190275,-1.30670041311));
#81123=CARTESIAN_POINT('Ctrl Pts',(3.90904845134,-19.1941294458,-1.40944736849));
#81124=CARTESIAN_POINT('Ctrl Pts',(3.84915166913,-19.1827174766,-1.3858993254));
#81125=CARTESIAN_POINT('Ctrl Pts',(3.78924978079,-19.1880794399,-1.35771639625));
#81126=CARTESIAN_POINT('Ctrl Pts',(3.734849471,-19.2113827948,-1.32722087289));
#81127=CARTESIAN_POINT('Ctrl Pts',(3.64784164979,-19.2891777792,-1.2678039989));
#81128=CARTESIAN_POINT('Ctrl Pts',(3.61523677607,-19.410557809,-1.22097222058));
#81129=CARTESIAN_POINT('Ctrl Pts',(3.61535581634,-19.4775453686,-1.20309998859));
#81130=CARTESIAN_POINT('Ctrl Pts',(3.63193270005,-19.5440428904,-1.19235380158));
#81131=CARTESIAN_POINT('Ctrl Pts',(3.66216118733,-19.6043893474,-1.18881869517));
#81132=CARTESIAN_POINT('Ctrl Pts',(3.94208066889,-19.1605170316,-1.34454941301));
#81133=CARTESIAN_POINT('Ctrl Pts',(3.87720137211,-19.1521640582,-1.33569518932));
#81134=CARTESIAN_POINT('Ctrl Pts',(3.81231524539,-19.1592950835,-1.31771475291));
#81135=CARTESIAN_POINT('Ctrl Pts',(3.7537820072,-19.1828102836,-1.29142806828));
#81136=CARTESIAN_POINT('Ctrl Pts',(3.66183896524,-19.2575993834,-1.2278312033));
#81137=CARTESIAN_POINT('Ctrl Pts',(3.63176679768,-19.3694757596,-1.15551654247));
#81138=CARTESIAN_POINT('Ctrl Pts',(3.6352563839,-19.4301693195,-1.12049065176));
#81139=CARTESIAN_POINT('Ctrl Pts',(3.65691133475,-19.4891756884,-1.09031631225));
#81140=CARTESIAN_POINT('Ctrl Pts',(3.69310715296,-19.5414102009,-1.06722029503));
#81141=CARTESIAN_POINT('Ctrl Pts',(3.94208066889,-19.1136682429,-1.29488929392));
#81142=CARTESIAN_POINT('Ctrl Pts',(3.87720137211,-19.1136682429,-1.29488929392));
#81143=CARTESIAN_POINT('Ctrl Pts',(3.81231524539,-19.1264162816,-1.28286293996));
#81144=CARTESIAN_POINT('Ctrl Pts',(3.7537820072,-19.15197936,-1.258747024));
#81145=CARTESIAN_POINT('Ctrl Pts',(3.66183896524,-19.223295201,-1.19146847485));
#81146=CARTESIAN_POINT('Ctrl Pts',(3.63176679768,-19.3185856331,-1.10157257054));
#81147=CARTESIAN_POINT('Ctrl Pts',(3.6352563839,-19.3681821823,-1.05478375298));
#81148=CARTESIAN_POINT('Ctrl Pts',(3.65691133475,-19.4144643672,-1.01112166887));
#81149=CARTESIAN_POINT('Ctrl Pts',(3.69310715296,-19.4536303653,-0.974172913988));
#81150=CARTESIAN_POINT('Ctrl Pts',(3.94208066889,-19.1136682429,-1.29488929392));
#81151=CARTESIAN_POINT('Ctrl Pts',(3.94208066889,-19.1213935505688,-1.30307818651436));
#81152=CARTESIAN_POINT('Ctrl Pts',(3.94100547669129,-19.1286717217873,-1.31174595495687));
#81153=CARTESIAN_POINT('Ctrl Pts',(3.93888533927808,-19.1354553093415,-1.32081024079185));
#81154=CARTESIAN_POINT('Ctrl Pts',(3.93647580748577,-19.1431648425896,-1.33111178292677));
#81155=CARTESIAN_POINT('Ctrl Pts',(3.93271701109205,-19.1502369295743,-1.34192670736547));
#81156=CARTESIAN_POINT('Ctrl Pts',(3.92760682263043,-19.1566129713568,-1.35318346930748));
#81157=CARTESIAN_POINT('Ctrl Pts',(3.92418283215508,-19.160885124233,-1.360725861523));
#81158=CARTESIAN_POINT('Ctrl Pts',(3.9201493937171,-19.1648460281206,-1.36847027143733));
#81159=CARTESIAN_POINT('Ctrl Pts',(3.91550264816662,-19.1684724142439,-1.37639078404052));
#81160=CARTESIAN_POINT('Ctrl Pts',(3.90804917436684,-19.1742892108954,-1.38909544637408));
#81161=CARTESIAN_POINT('Ctrl Pts',(3.89901903058555,-19.1792414439433,-1.40224844154212));
#81162=CARTESIAN_POINT('Ctrl Pts',(3.88841602773183,-19.1832466824446,-1.41573314937972));
#81163=CARTESIAN_POINT('Ctrl Pts',(3.88311452630497,-19.1852493016953,-1.42247550329852));
#81164=CARTESIAN_POINT('Ctrl Pts',(3.87742029106335,-19.1870154827717,-1.42930055218608));
#81165=CARTESIAN_POINT('Ctrl Pts',(3.87133657591744,-19.1885374657265,-1.43619304513296));
#81166=CARTESIAN_POINT('Ctrl Pts',(3.86981564713096,-19.1889179614652,-1.43791616836967));
#81167=CARTESIAN_POINT('Ctrl Pts',(3.86827038117942,-19.1892832054479,-1.43964351009775));
#81168=CARTESIAN_POINT('Ctrl Pts',(3.86670084145296,-19.1896330966815,-1.44137483565682));
#81169=CARTESIAN_POINT('Ctrl Pts',(3.8655236866581,-19.1898955151067,-1.44267332982611));
#81170=CARTESIAN_POINT('Ctrl Pts',(3.86433287805002,-19.1901492977467,-1.44397406482564));
#81171=CARTESIAN_POINT('Ctrl Pts',(3.86312844582096,-19.1903944045625,-1.44527694032169));
#81172=CARTESIAN_POINT('Ctrl Pts',(3.862820679794,-19.1904570361901,-1.44560986134903));
#81173=CARTESIAN_POINT('Ctrl Pts',(3.86251175890315,-19.1905191679455,-1.44594322302894));
#81174=CARTESIAN_POINT('Ctrl Pts',(3.86219392101923,-19.1905822995663,-1.44628533346112));
#81175=CARTESIAN_POINT('Ctrl Pts',(3.86025365777512,-19.1909676908916,-1.44837377014711));
#81176=CARTESIAN_POINT('Ctrl Pts',(3.85806644600599,-19.1913687357961,-1.45069123929498));
#81177=CARTESIAN_POINT('Ctrl Pts',(3.85604432062616,-19.191709360832,-1.45280045778785));
#81178=CARTESIAN_POINT('Ctrl Pts',(3.85450871101005,-19.191968032765,-1.45440220624145));
#81179=CARTESIAN_POINT('Ctrl Pts',(3.85306958970826,-19.1921930668317,-1.45588408049776));
#81180=CARTESIAN_POINT('Ctrl Pts',(3.85192149540446,-19.1923651413728,-1.4570580131927));
#81181=CARTESIAN_POINT('Ctrl Pts',(3.84000156819927,-19.1941516810292,-1.46924620385017));
#81182=CARTESIAN_POINT('Ctrl Pts',(3.82674560647647,-19.1952061457583,-1.48176044555951));
#81183=CARTESIAN_POINT('Ctrl Pts',(3.81213319489629,-19.1954494376464,-1.49450176335358));
#81184=CARTESIAN_POINT('Ctrl Pts',(3.79903811735577,-19.1956674664175,-1.50592003908214));
#81185=CARTESIAN_POINT('Ctrl Pts',(3.78485595743091,-19.1952349372733,-1.51751939205409));
#81186=CARTESIAN_POINT('Ctrl Pts',(3.7695910419071,-19.194107055607,-1.52921902692643));
#81187=CARTESIAN_POINT('Ctrl Pts',(3.7565253000351,-19.1931416646952,-1.5392331281509));
#81188=CARTESIAN_POINT('Ctrl Pts',(3.74266668945736,-19.1916672093887,-1.54932575197495));
#81189=CARTESIAN_POINT('Ctrl Pts',(3.72802076749187,-19.1896517157489,-1.55943647497926));
#81190=CARTESIAN_POINT('Ctrl Pts',(3.72456428981541,-19.1891760537326,-1.56182263328596));
#81191=CARTESIAN_POINT('Ctrl Pts',(3.72106378520022,-19.1886701887527,-1.56420988691519));
#81192=CARTESIAN_POINT('Ctrl Pts',(3.71751888906543,-19.1881335052326,-1.56659763778155));
#81193=CARTESIAN_POINT('Ctrl Pts',(3.71330638744845,-19.187495748833,-1.56943507053078));
#81194=CARTESIAN_POINT('Ctrl Pts',(3.70903224195872,-19.1868146164059,-1.57227260091458));
#81195=CARTESIAN_POINT('Ctrl Pts',(3.70469541744933,-19.186088937794,-1.57510915486651));
#81196=CARTESIAN_POINT('Ctrl Pts',(3.69947554797873,-19.1852154997234,-1.57852327534644));
#81197=CARTESIAN_POINT('Ctrl Pts',(3.69416478422523,-19.1842774765037,-1.58193601403412));
#81198=CARTESIAN_POINT('Ctrl Pts',(3.68876462401809,-19.1832745138145,-1.5853441458696));
#81199=CARTESIAN_POINT('Ctrl Pts',(3.68382123617734,-19.18235638669,-1.58846400099036));
#81200=CARTESIAN_POINT('Ctrl Pts',(3.6788023431847,-19.1813837619823,-1.59158029219753));
#81201=CARTESIAN_POINT('Ctrl Pts',(3.67370794478431,-19.180356266959,-1.59469101971277));
#81202=CARTESIAN_POINT('Ctrl Pts',(3.67073041486801,-19.1797557255544,-1.59650915082662));
#81203=CARTESIAN_POINT('Ctrl Pts',(3.66714567548281,-19.1790161110558,-1.59867569128098));
#81204=CARTESIAN_POINT('Ctrl Pts',(3.66397164750743,-19.1783453305908,-1.60057321268494));
#81205=CARTESIAN_POINT('Ctrl Pts',(3.66171507915125,-19.1778684406632,-1.60192225144219));
#81206=CARTESIAN_POINT('Ctrl Pts',(3.65966673795962,-19.1774276304334,-1.60313640354589));
#81207=CARTESIAN_POINT('Ctrl Pts',(3.65819753823164,-19.1771090035203,-1.60400401677888));
#81208=CARTESIAN_POINT('Ctrl Pts',(3.64039240413172,-19.1732475850841,-1.61451856402934));
#81209=CARTESIAN_POINT('Ctrl Pts',(3.62101617997714,-19.1686042876446,-1.62534500838972));
#81210=CARTESIAN_POINT('Ctrl Pts',(3.60005819365773,-19.1630368846854,-1.63633013020167));
#81211=CARTESIAN_POINT('Ctrl Pts',(3.58772155265733,-19.1597597066891,-1.64279637662794));
#81212=CARTESIAN_POINT('Ctrl Pts',(3.57483761059001,-19.1561624128229,-1.64931684911771));
#81213=CARTESIAN_POINT('Ctrl Pts',(3.56140967667491,-19.1522164502068,-1.65585401051031));
#81214=CARTESIAN_POINT('Ctrl Pts',(3.54328975021503,-19.1468916881943,-1.66467538872375));
#81215=CARTESIAN_POINT('Ctrl Pts',(3.52417557959925,-19.1409320159719,-1.6735269623939));
#81216=CARTESIAN_POINT('Ctrl Pts',(3.50406715587264,-19.1342760287435,-1.68229465773077));
#81217=CARTESIAN_POINT('Ctrl Pts',(3.49401294400934,-19.1309480351293,-1.6866785053992));
#81218=CARTESIAN_POINT('Ctrl Pts',(3.48371016856777,-19.127446123929,-1.69104102801887));
#81219=CARTESIAN_POINT('Ctrl Pts',(3.4731588282599,-19.1237639580102,-1.69536587194679));
#81220=CARTESIAN_POINT('Ctrl Pts',(3.46788315810597,-19.1219228750509,-1.69752829391075));
#81221=CARTESIAN_POINT('Ctrl Pts',(3.4625453467471,-19.1200367283689,-1.69968129414405));
#81222=CARTESIAN_POINT('Ctrl Pts',(3.45714539413792,-19.1181048645026,-1.70182267645465));
#81223=CARTESIAN_POINT('Ctrl Pts',(3.4533090413257,-19.1167323873879,-1.70334400425951));
#81224=CARTESIAN_POINT('Ctrl Pts',(3.44887872706727,-19.1151331100681,-1.70507852129202));
#81225=CARTESIAN_POINT('Ctrl Pts',(3.4450536379338,-19.1137401653745,-1.70655720634178));
#81226=CARTESIAN_POINT('Ctrl Pts',(3.44349462892571,-19.1131724365584,-1.7071598807455));
#81227=CARTESIAN_POINT('Ctrl Pts',(3.44203611491941,-19.112639349284,-1.70772063898745));
#81228=CARTESIAN_POINT('Ctrl Pts',(3.44075911260381,-19.1121714939915,-1.70820976488904));
#81229=CARTESIAN_POINT('Ctrl Pts',(3.40930114555862,-19.1006462397352,-1.72025900419344));
#81230=CARTESIAN_POINT('Ctrl Pts',(3.37748624251822,-19.0881949128326,-1.73126263301116));
#81231=CARTESIAN_POINT('Ctrl Pts',(3.34544565726412,-19.0748903340227,-1.74118643674611));
#81232=CARTESIAN_POINT('Ctrl Pts',(3.3214711174372,-19.0649351115439,-1.74861197613596));
#81233=CARTESIAN_POINT('Ctrl Pts',(3.29736784319479,-19.0545004799544,-1.75543361106648));
#81234=CARTESIAN_POINT('Ctrl Pts',(3.27320280002085,-19.0436061687958,-1.76161889253852));
#81235=CARTESIAN_POINT('Ctrl Pts',(3.25722224928904,-19.036401667198,-1.76570927233396));
#81236=CARTESIAN_POINT('Ctrl Pts',(3.2412149341913,-19.0289959526638,-1.76952101126774));
#81237=CARTESIAN_POINT('Ctrl Pts',(3.22521062098,-19.0213954214,-1.77303668325));
#81238=CARTESIAN_POINT('Origin',(2.225,-18.895449313,-1.50075453779));
#81239=CARTESIAN_POINT('Origin',(4.35,-19.0026826744,-1.32221314666));
#81240=CARTESIAN_POINT('Origin',(4.35,-19.0026826744,-1.32221314666));
#81241=CARTESIAN_POINT('Origin',(-4.4408920985E-16,-17.4373752488,-0.853039529372));
#81242=CARTESIAN_POINT('',(2.225,-19.0254782583,-1.22484599945));
#81243=CARTESIAN_POINT('Ctrl Pts',(2.33871339945,-17.3446807781,1.27988117638));
#81244=CARTESIAN_POINT('Ctrl Pts',(2.30368136515,-17.3797447944,1.24671241384));
#81245=CARTESIAN_POINT('Ctrl Pts',(2.26864933085,-17.4046242188,1.20277711487));
#81246=CARTESIAN_POINT('Ctrl Pts',(2.23651128313,-17.4163976498,1.15078915349));
#81247=CARTESIAN_POINT('Ctrl Pts',(2.21010974441,-17.4140237598,1.09534672271));
#81248=CARTESIAN_POINT('Ctrl Pts',(2.19100518783,-17.3987921062,1.04094168425));
#81249=CARTESIAN_POINT('Ctrl Pts',(2.46656348386,-17.3868132718,1.24002603887));
#81250=CARTESIAN_POINT('Ctrl Pts',(2.42844748972,-17.4291544248,1.20768003199));
#81251=CARTESIAN_POINT('Ctrl Pts',(2.39033149557,-17.4606361606,1.16135256604));
#81252=CARTESIAN_POINT('Ctrl Pts',(2.35591441479,-17.4771747692,1.10419328591));
#81253=CARTESIAN_POINT('Ctrl Pts',(2.32881040502,-17.477098625,1.04217993252));
#81254=CARTESIAN_POINT('Ctrl Pts',(2.31078053575,-17.4619464725,0.981200951561));
#81255=CARTESIAN_POINT('Ctrl Pts',(2.59487812775,-17.4343620581,1.20661041268));
#81256=CARTESIAN_POINT('Ctrl Pts',(2.55330984454,-17.4840818306,1.17681423799));
#81257=CARTESIAN_POINT('Ctrl Pts',(2.51174156132,-17.5227993839,1.12922208024));
#81258=CARTESIAN_POINT('Ctrl Pts',(2.47489289955,-17.5449043891,1.06729320786));
#81259=CARTESIAN_POINT('Ctrl Pts',(2.44734293975,-17.5477841071,0.998707070211));
#81260=CARTESIAN_POINT('Ctrl Pts',(2.43099106691,-17.5332197496,0.93111255917));
#81261=CARTESIAN_POINT('Ctrl Pts',(2.72261491105,-17.4869576367,1.17969475941));
#81262=CARTESIAN_POINT('Ctrl Pts',(2.67711454496,-17.5437282683,1.15424808256));
#81263=CARTESIAN_POINT('Ctrl Pts',(2.63161417887,-17.5901493824,1.10663321957));
#81264=CARTESIAN_POINT('Ctrl Pts',(2.59215946779,-17.6186952055,1.0403312197));
#81265=CARTESIAN_POINT('Ctrl Pts',(2.56454650279,-17.6253471943,0.965088224411));
#81266=CARTESIAN_POINT('Ctrl Pts',(2.55066029792,-17.6120575799,0.890767574454));
#81267=CARTESIAN_POINT('Ctrl Pts',(2.97172474664,-17.6000943145,1.1412362125));
#81268=CARTESIAN_POINT('Ctrl Pts',(2.91735433119,-17.6692765139,1.12809880562));
#81269=CARTESIAN_POINT('Ctrl Pts',(2.86298391574,-17.7315429739,1.08325341223));
#81270=CARTESIAN_POINT('Ctrl Pts',(2.8179996123,-17.7746943065,1.00928125711));
#81271=CARTESIAN_POINT('Ctrl Pts',(2.79121040663,-17.7907023387,0.920813266721));
#81272=CARTESIAN_POINT('Ctrl Pts',(2.78403685548,-17.7816436282,0.833120105007));
#81273=CARTESIAN_POINT('Ctrl Pts',(3.21130945297,-17.7305299504,1.13861871946));
#81274=CARTESIAN_POINT('Ctrl Pts',(3.14443125953,-17.8051039402,1.14445298434));
#81275=CARTESIAN_POINT('Ctrl Pts',(3.07755306609,-17.8822389016,1.10879949478));
#81276=CARTESIAN_POINT('Ctrl Pts',(3.02603277475,-17.9446380869,1.03007665658));
#81277=CARTESIAN_POINT('Ctrl Pts',(3.0034518946,-17.976136713,0.929176763913));
#81278=CARTESIAN_POINT('Ctrl Pts',(3.00848992062,-17.9771596623,0.8291967484));
#81279=CARTESIAN_POINT('Ctrl Pts',(3.325392695,-17.7982565946,1.14774886529));
#81280=CARTESIAN_POINT('Ctrl Pts',(3.2513090753,-17.8730342715,1.1640276349));
#81281=CARTESIAN_POINT('Ctrl Pts',(3.1772254556,-17.9567834794,1.13437155799));
#81282=CARTESIAN_POINT('Ctrl Pts',(3.12223578852,-18.0298580146,1.05431482767));
#81283=CARTESIAN_POINT('Ctrl Pts',(3.10275958695,-18.0708463807,0.948032090962));
#81284=CARTESIAN_POINT('Ctrl Pts',(3.1153678987,-18.0786783194,0.842882322279));
#81285=CARTESIAN_POINT('Ctrl Pts',(3.43467455982,-17.8694391349,1.1700344079));
#81286=CARTESIAN_POINT('Ctrl Pts',(3.35146956174,-17.9400304974,1.19792357011));
#81287=CARTESIAN_POINT('Ctrl Pts',(3.26826456366,-18.0285526893,1.17642640861));
#81288=CARTESIAN_POINT('Ctrl Pts',(3.20940399066,-18.1140150626,1.09643232242));
#81289=CARTESIAN_POINT('Ctrl Pts',(3.19494098605,-18.1676222846,0.985546029641));
#81290=CARTESIAN_POINT('Ctrl Pts',(3.21774774552,-18.1853772775,0.876287149069));
#81291=CARTESIAN_POINT('Ctrl Pts',(3.53153633351,-17.9397782658,1.2109699402));
#81292=CARTESIAN_POINT('Ctrl Pts',(3.43735910775,-18.0003263168,1.24620732043));
#81293=CARTESIAN_POINT('Ctrl Pts',(3.34318188199,-18.0897485104,1.23183053971));
#81294=CARTESIAN_POINT('Ctrl Pts',(3.28035125045,-18.1886331584,1.15483676411));
#81295=CARTESIAN_POINT('Ctrl Pts',(3.27308199046,-18.2588703505,1.04489921328));
#81296=CARTESIAN_POINT('Ctrl Pts',(3.3084919335,-18.2908119326,0.937647357484));
#81297=CARTESIAN_POINT('Ctrl Pts',(3.53153633351,-17.9397782658,1.2109699402));
#81298=CARTESIAN_POINT('Ctrl Pts',(3.50556811491538,-17.9209206519348,1.19999530273144));
#81299=CARTESIAN_POINT('Ctrl Pts',(3.47707465175054,-17.9009947410055,1.19005350125579));
#81300=CARTESIAN_POINT('Ctrl Pts',(3.44603904201575,-17.8801221407561,1.18138128795028));
#81301=CARTESIAN_POINT('Ctrl Pts',(3.40908705834256,-17.8552705592913,1.17105587507089));
#81302=CARTESIAN_POINT('Ctrl Pts',(3.3685335775199,-17.8290766670107,1.16252994367687));
#81303=CARTESIAN_POINT('Ctrl Pts',(3.32439190884036,-17.8017986399993,1.15617041085934));
#81304=CARTESIAN_POINT('Ctrl Pts',(3.31431861168232,-17.7955736901913,1.15471914121381));
#81305=CARTESIAN_POINT('Ctrl Pts',(3.30405849594343,-17.7892924725729,1.15338059333593));
#81306=CARTESIAN_POINT('Ctrl Pts',(3.29361170856435,-17.7829583723188,1.15215898525626));
#81307=CARTESIAN_POINT('Ctrl Pts',(3.25114950591464,-17.7572126728199,1.14719361475952));
#81308=CARTESIAN_POINT('Ctrl Pts',(3.20559642908899,-17.7306009301782,1.14416617105331));
#81309=CARTESIAN_POINT('Ctrl Pts',(3.1569521793853,-17.703441631524,1.14334279135102));
#81310=CARTESIAN_POINT('Ctrl Pts',(3.15136773655507,-17.7003236977175,1.14324826595689));
#81311=CARTESIAN_POINT('Ctrl Pts',(3.14574255851777,-17.6971985681436,1.14318273767508));
#81312=CARTESIAN_POINT('Ctrl Pts',(3.14007665104147,-17.6940667421653,1.14314657180127));
#81313=CARTESIAN_POINT('Ctrl Pts',(3.11256676654638,-17.6788606747737,1.14297097433246));
#81314=CARTESIAN_POINT('Ctrl Pts',(3.08409652814019,-17.6634980322924,1.14348805625532));
#81315=CARTESIAN_POINT('Ctrl Pts',(3.0546659359017,-17.6480454008806,1.14473598939578));
#81316=CARTESIAN_POINT('Ctrl Pts',(3.03995063978245,-17.6403190851746,1.14535995596601));
#81317=CARTESIAN_POINT('Ctrl Pts',(3.02499521890932,-17.632570287484,1.14616660890463));
#81318=CARTESIAN_POINT('Ctrl Pts',(3.00979681525875,-17.6248116462183,1.14715957583797));
#81319=CARTESIAN_POINT('Ctrl Pts',(3.00219761343346,-17.6209323255855,1.14765605930464));
#81320=CARTESIAN_POINT('Ctrl Pts',(2.99453711990554,-17.6170512120295,1.14819899664201));
#81321=CARTESIAN_POINT('Ctrl Pts',(2.98681744787082,-17.6131669151875,1.14878923028722));
#81322=CARTESIAN_POINT('Ctrl Pts',(2.9845683002017,-17.6120352146245,1.14896119648233));
#81323=CARTESIAN_POINT('Ctrl Pts',(2.98231412808812,-17.6109032447226,1.149137179012));
#81324=CARTESIAN_POINT('Ctrl Pts',(2.98005493497421,-17.6097710297417,1.14931719275426));
#81325=CARTESIAN_POINT('Ctrl Pts',(2.97846279508803,-17.608973114495,1.1494440553307));
#81326=CARTESIAN_POINT('Ctrl Pts',(2.97686816150228,-17.6081750775378,1.14957292003385));
#81327=CARTESIAN_POINT('Ctrl Pts',(2.97527103558563,-17.607376927504,1.1497037920794));
#81328=CARTESIAN_POINT('Ctrl Pts',(2.97491126692257,-17.6071971361879,1.14973327232286));
#81329=CARTESIAN_POINT('Ctrl Pts',(2.97454370653952,-17.6070135083179,1.14976348226065));
#81330=CARTESIAN_POINT('Ctrl Pts',(2.974167052028,-17.6068254014812,1.14979454198035));
#81331=CARTESIAN_POINT('Ctrl Pts',(2.97384315794509,-17.6066636439833,1.14982125096464));
#81332=CARTESIAN_POINT('Ctrl Pts',(2.97351352309312,-17.6064990661748,1.1498485076559));
#81333=CARTESIAN_POINT('Ctrl Pts',(2.97317996049783,-17.6063325774542,1.14987616875897));
#81334=CARTESIAN_POINT('Ctrl Pts',(2.96968027511006,-17.6045858044311,1.15016638462728));
#81335=CARTESIAN_POINT('Ctrl Pts',(2.96574739989838,-17.6026302164279,1.15050426861635));
#81336=CARTESIAN_POINT('Ctrl Pts',(2.96348100707217,-17.6015054896627,1.15070247652069));
#81337=CARTESIAN_POINT('Ctrl Pts',(2.92803905491366,-17.5839169623146,1.15380206057428));
#81338=CARTESIAN_POINT('Ctrl Pts',(2.88987049590359,-17.5655398311131,1.15801219935198));
#81339=CARTESIAN_POINT('Ctrl Pts',(2.84895815223916,-17.5465854691076,1.16361465647827));
#81340=CARTESIAN_POINT('Ctrl Pts',(2.83971491844516,-17.5423031527272,1.16488040701712));
#81341=CARTESIAN_POINT('Ctrl Pts',(2.83033174950334,-17.5379915451762,1.16621721245778));
#81342=CARTESIAN_POINT('Ctrl Pts',(2.82080866325753,-17.5336533934426,1.16762830374947));
#81343=CARTESIAN_POINT('Ctrl Pts',(2.79497160771564,-17.5218835675274,1.17145673112451));
#81344=CARTESIAN_POINT('Ctrl Pts',(2.76810639391988,-17.5099151377531,1.17583291465314));
#81345=CARTESIAN_POINT('Ctrl Pts',(2.74021302188449,-17.4978111868782,1.18082044452999));
#81346=CARTESIAN_POINT('Ctrl Pts',(2.72626633586679,-17.4917592114407,1.18331420946842));
#81347=CARTESIAN_POINT('Ctrl Pts',(2.71206261028851,-17.4856733693343,1.18596084863352));
#81348=CARTESIAN_POINT('Ctrl Pts',(2.69760184513937,-17.4795629428546,1.18876792472649));
#81349=CARTESIAN_POINT('Ctrl Pts',(2.6903714625648,-17.4765077296148,1.19017146277297));
#81350=CARTESIAN_POINT('Ctrl Pts',(2.68307682009751,-17.4734463704891,1.19161511116579));
#81351=CARTESIAN_POINT('Ctrl Pts',(2.67571791773619,-17.4703800732671,1.19309980222432));
#81352=CARTESIAN_POINT('Ctrl Pts',(2.67203846655553,-17.4688469246562,1.19384214775358));
#81353=CARTESIAN_POINT('Ctrl Pts',(2.66834295040137,-17.4673125415659,1.19459475404243));
#81354=CARTESIAN_POINT('Ctrl Pts',(2.6646313692736,-17.4657770799259,1.19535773587256));
#81355=CARTESIAN_POINT('Ctrl Pts',(2.66277557870971,-17.4650093491059,1.19573922678762));
#81356=CARTESIAN_POINT('Ctrl Pts',(2.66091577190243,-17.4642413486511,1.1961233115932));
#81357=CARTESIAN_POINT('Ctrl Pts',(2.65905194885173,-17.4634730983855,1.19651000450817));
#81358=CARTESIAN_POINT('Ctrl Pts',(2.65718812580103,-17.4627048481199,1.19689669742315));
#81359=CARTESIAN_POINT('Ctrl Pts',(2.65385512538322,-17.4613346385436,1.19759276935488));
#81360=CARTESIAN_POINT('Ctrl Pts',(2.65344843096939,-17.4611676180876,1.19767792176957));
#81361=CARTESIAN_POINT('Ctrl Pts',(2.64868306052613,-17.4592105851962,1.19867568024947));
#81362=CARTESIAN_POINT('Ctrl Pts',(2.64128756638981,-17.4561782064591,1.2002330735104));
#81363=CARTESIAN_POINT('Ctrl Pts',(2.63125348900647,-17.4521133445083,1.20241115568425));
#81364=CARTESIAN_POINT('Ctrl Pts',(2.62114362876218,-17.4480177824884,1.20460568793041));
#81365=CARTESIAN_POINT('Ctrl Pts',(2.60835491676642,-17.442873956329,1.20743048208744));
#81366=CARTESIAN_POINT('Ctrl Pts',(2.59287672241144,-17.4367582258099,1.21098967640617));
#81367=CARTESIAN_POINT('Ctrl Pts',(2.57741059224131,-17.4306472620809,1.21454609657843));
#81368=CARTESIAN_POINT('Ctrl Pts',(2.5592587583199,-17.4235657759116,1.21883599503214));
#81369=CARTESIAN_POINT('Ctrl Pts',(2.53841370144026,-17.4156241624524,1.22400164543882));
#81370=CARTESIAN_POINT('Ctrl Pts',(2.51788460629228,-17.4078029250591,1.22908899681004));
#81371=CARTESIAN_POINT('Ctrl Pts',(2.49474277554049,-17.3991473310975,1.23502591824219));
#81372=CARTESIAN_POINT('Ctrl Pts',(2.46899103022168,-17.3897976559456,1.24198241379793));
#81373=CARTESIAN_POINT('Ctrl Pts',(2.44461188735642,-17.3809463309791,1.24856811884025));
#81374=CARTESIAN_POINT('Ctrl Pts',(2.41789312181659,-17.3714729933677,1.25606770645213));
#81375=CARTESIAN_POINT('Ctrl Pts',(2.38885356688222,-17.3615281457323,1.26465399261196));
#81376=CARTESIAN_POINT('Ctrl Pts',(2.37284312652012,-17.3560452314681,1.26938788825205));
#81377=CARTESIAN_POINT('Ctrl Pts',(2.35612757048598,-17.3504195498407,1.27445259817871));
#81378=CARTESIAN_POINT('Ctrl Pts',(2.33871339945,-17.3446807781,1.27988117638));
#81379=CARTESIAN_POINT('Origin',(3.225,-17.6882812316,1.64311487169));
#81380=CARTESIAN_POINT('',(0.,-17.9397782658,1.2109699402));
#81381=CARTESIAN_POINT('Origin',(-4.4408920985E-16,-18.4073812884,1.48310265486));
#81382=CARTESIAN_POINT('',(2.225,-18.3719297863,1.46247080897));
#81383=CARTESIAN_POINT('Origin',(4.35,-18.3216303794,1.54889979527));
#81384=CARTESIAN_POINT('Origin',(4.35,-18.3216303794,1.54889979527));
#81385=CARTESIAN_POINT('Ctrl Pts',(3.94208068347,-18.560475405,1.92017998057));
#81386=CARTESIAN_POINT('Ctrl Pts',(3.87720138837,-18.5604754047,1.92017997921));
#81387=CARTESIAN_POINT('Ctrl Pts',(3.81231526335,-18.5765098903,1.91310601594));
#81388=CARTESIAN_POINT('Ctrl Pts',(3.7537820265,-18.6086631358,1.8989209116));
#81389=CARTESIAN_POINT('Ctrl Pts',(3.66183898589,-18.6983642164,1.85934732843));
#81390=CARTESIAN_POINT('Ctrl Pts',(3.63176681675,-18.8182205442,1.80647010407));
#81391=CARTESIAN_POINT('Ctrl Pts',(3.63525640136,-18.8806030959,1.77894868584));
#81392=CARTESIAN_POINT('Ctrl Pts',(3.65691134997,-18.9388168398,1.75326642816));
#81393=CARTESIAN_POINT('Ctrl Pts',(3.69310716565,-18.9880798429,1.73153298464));
#81394=CARTESIAN_POINT('Ctrl Pts',(3.94208074492,-18.5766887246,1.9569305147));
#81395=CARTESIAN_POINT('Ctrl Pts',(3.87720145143,-18.573797947,1.95037801966));
#81396=CARTESIAN_POINT('Ctrl Pts',(3.81231532801,-18.5878885088,1.93889778448));
#81397=CARTESIAN_POINT('Ctrl Pts',(3.75378209234,-18.6193330273,1.92310621435));
#81398=CARTESIAN_POINT('Ctrl Pts',(3.66183905239,-18.7102361193,1.88625721169));
#81399=CARTESIAN_POINT('Ctrl Pts',(3.63176688029,-18.8358324651,1.84639081277));
#81400=CARTESIAN_POINT('Ctrl Pts',(3.63525646243,-18.902055441,1.82757443591));
#81401=CARTESIAN_POINT('Ctrl Pts',(3.65691140785,-18.9646727386,1.81187365705));
#81402=CARTESIAN_POINT('Ctrl Pts',(3.69310722012,-19.0184584616,1.80039180405));
#81403=CARTESIAN_POINT('Ctrl Pts',(3.9309703758,-18.5868132355,1.99657589927));
#81404=CARTESIAN_POINT('Ctrl Pts',(3.86765536306,-18.583214534,1.98238806807));
#81405=CARTESIAN_POINT('Ctrl Pts',(3.80433403936,-18.5969151126,1.96571696787));
#81406=CARTESIAN_POINT('Ctrl Pts',(3.747100735,-18.6283553041,1.94794658657));
#81407=CARTESIAN_POINT('Ctrl Pts',(3.65672049689,-18.7201473882,1.91392916105));
#81408=CARTESIAN_POINT('Ctrl Pts',(3.62587466002,-18.8484282953,1.88855630444));
#81409=CARTESIAN_POINT('Ctrl Pts',(3.62831693429,-18.9164444968,1.87945311729));
#81410=CARTESIAN_POINT('Ctrl Pts',(3.64838248883,-18.9812381625,1.8748423295));
#81411=CARTESIAN_POINT('Ctrl Pts',(3.68269856573,-19.037428697,1.87467495374));
#81412=CARTESIAN_POINT('Ctrl Pts',(3.90873107927,-18.5892873009,2.03559195441));
#81413=CARTESIAN_POINT('Ctrl Pts',(3.84843942238,-18.5881253798,2.01531034459));
#81414=CARTESIAN_POINT('Ctrl Pts',(3.78814242491,-18.6037700715,1.99484202289));
#81415=CARTESIAN_POINT('Ctrl Pts',(3.73342452262,-18.6363892469,1.97609984706));
#81416=CARTESIAN_POINT('Ctrl Pts',(3.64608120201,-18.728999463,1.94582805337));
#81417=CARTESIAN_POINT('Ctrl Pts',(3.61376485716,-18.855867862,1.93373053153));
#81418=CARTESIAN_POINT('Ctrl Pts',(3.61419481888,-18.9228203826,1.93320496012));
#81419=CARTESIAN_POINT('Ctrl Pts',(3.63119178412,-18.9865881277,1.93820769667));
#81420=CARTESIAN_POINT('Ctrl Pts',(3.6618638453,-19.0420643013,1.94777851272));
#81421=CARTESIAN_POINT('Ctrl Pts',(3.84485695788,-18.5827804967,2.11566725872));
#81422=CARTESIAN_POINT('Ctrl Pts',(3.79152009507,-18.5888985515,2.08692370546));
#81423=CARTESIAN_POINT('Ctrl Pts',(3.73817980644,-18.6098769483,2.06216975114));
#81424=CARTESIAN_POINT('Ctrl Pts',(3.68928525628,-18.6452122306,2.04386917313));
#81425=CARTESIAN_POINT('Ctrl Pts',(3.60913704956,-18.7381762607,2.02344540596));
#81426=CARTESIAN_POINT('Ctrl Pts',(3.57378597362,-18.8578355373,2.03575440104));
#81427=CARTESIAN_POINT('Ctrl Pts',(3.56976842438,-18.9199130291,2.05024905768));
#81428=CARTESIAN_POINT('Ctrl Pts',(3.57980389627,-18.9786742001,2.07169908381));
#81429=CARTESIAN_POINT('Ctrl Pts',(3.60202389653,-19.0298725019,2.09781456345));
#81430=CARTESIAN_POINT('Ctrl Pts',(3.75754974665,-18.5555835484,2.18057996716));
#81431=CARTESIAN_POINT('Ctrl Pts',(3.71097917267,-18.570346009,2.15154816967));
#81432=CARTESIAN_POINT('Ctrl Pts',(3.66440657994,-18.5969345937,2.12885177485));
#81433=CARTESIAN_POINT('Ctrl Pts',(3.6212405898,-18.6342490738,2.11465497547));
#81434=CARTESIAN_POINT('Ctrl Pts',(3.54845228546,-18.7244284924,2.10544382014));
#81435=CARTESIAN_POINT('Ctrl Pts',(3.5107816715,-18.8312096705,2.13301209303));
#81436=CARTESIAN_POINT('Ctrl Pts',(3.50278189077,-18.8851477119,2.15564806317));
#81437=CARTESIAN_POINT('Ctrl Pts',(3.50627219288,-18.9354336643,2.18531444577));
#81438=CARTESIAN_POINT('Ctrl Pts',(3.52023080346,-18.9789141355,2.21944021466));
#81439=CARTESIAN_POINT('Ctrl Pts',(3.70638924491,-18.5368582595,2.21099047066));
#81440=CARTESIAN_POINT('Ctrl Pts',(3.66291643405,-18.5553781779,2.18355413245));
#81441=CARTESIAN_POINT('Ctrl Pts',(3.61944208646,-18.5840852858,2.16319877519));
#81442=CARTESIAN_POINT('Ctrl Pts',(3.57892432105,-18.6217121176,2.15180573279));
#81443=CARTESIAN_POINT('Ctrl Pts',(3.50965240858,-18.709332499,2.14854765445));
#81444=CARTESIAN_POINT('Ctrl Pts',(3.47118766711,-18.80892295,2.18210077644));
#81445=CARTESIAN_POINT('Ctrl Pts',(3.46151440616,-18.8585337116,2.20756445935));
#81446=CARTESIAN_POINT('Ctrl Pts',(3.46211782876,-18.9043879244,2.23984745237));
#81447=CARTESIAN_POINT('Ctrl Pts',(3.47230150547,-18.9438289149,2.27642005797));
#81448=CARTESIAN_POINT('Ctrl Pts',(3.653040134,-18.5154874832,2.23714441069));
#81449=CARTESIAN_POINT('Ctrl Pts',(3.6123450469,-18.5369866519,2.2120117706));
#81450=CARTESIAN_POINT('Ctrl Pts',(3.57164880036,-18.5671228869,2.19437159188));
#81451=CARTESIAN_POINT('Ctrl Pts',(3.53351916143,-18.6045418784,2.18582044714));
#81452=CARTESIAN_POINT('Ctrl Pts',(3.46747923522,-18.6889362982,2.18800948694));
#81453=CARTESIAN_POINT('Ctrl Pts',(3.42846086971,-18.7812883476,2.22611332253));
#81454=CARTESIAN_POINT('Ctrl Pts',(3.4173813101,-18.8266730185,2.25351528442));
#81455=CARTESIAN_POINT('Ctrl Pts',(3.4154812712,-18.8682463624,2.28742585674));
#81456=CARTESIAN_POINT('Ctrl Pts',(3.42232180975,-18.9037867018,2.32542426548));
#81457=CARTESIAN_POINT('Ctrl Pts',(3.59839803273,-18.4921598488,2.25921115747));
#81458=CARTESIAN_POINT('Ctrl Pts',(3.56014406941,-18.515804635,2.23684440141));
#81459=CARTESIAN_POINT('Ctrl Pts',(3.52188922088,-18.5466712753,2.22211105827));
#81460=CARTESIAN_POINT('Ctrl Pts',(3.48587211338,-18.5833900306,2.21633478685));
#81461=CARTESIAN_POINT('Ctrl Pts',(3.42275307116,-18.6640035029,2.22340619898));
#81462=CARTESIAN_POINT('Ctrl Pts',(3.38341089221,-18.7492623786,2.26482681385));
#81463=CARTESIAN_POINT('Ctrl Pts',(3.37119264755,-18.7906308355,2.29343152682));
#81464=CARTESIAN_POINT('Ctrl Pts',(3.36718144669,-18.8281878268,2.32816820766));
#81465=CARTESIAN_POINT('Ctrl Pts',(3.37113078856,-18.8600780815,2.3667703805));
#81466=CARTESIAN_POINT('Ctrl Pts',(3.59839803273,-18.4921598488,2.25921115747));
#81467=CARTESIAN_POINT('Ctrl Pts',(3.62233696850021,-18.5023797841465,2.2495436223255));
#81468=CARTESIAN_POINT('Ctrl Pts',(3.64495292720081,-18.5117286768719,2.23933546288846));
#81469=CARTESIAN_POINT('Ctrl Pts',(3.66623232550782,-18.5202015158469,2.22875537729148));
#81470=CARTESIAN_POINT('Ctrl Pts',(3.68905088268763,-18.5292872032258,2.21741002416266));
#81471=CARTESIAN_POINT('Ctrl Pts',(3.71033413511391,-18.537364597701,2.20563343890839));
#81472=CARTESIAN_POINT('Ctrl Pts',(3.73009481200645,-18.5444472306444,2.19361958363631));
#81473=CARTESIAN_POINT('Ctrl Pts',(3.74918903963728,-18.5512909944679,2.18201090805619));
#81474=CARTESIAN_POINT('Ctrl Pts',(3.76685603736808,-18.5572088969338,2.1701786682227));
#81475=CARTESIAN_POINT('Ctrl Pts',(3.78307881567319,-18.5622509716294,2.15826715051219));
#81476=CARTESIAN_POINT('Ctrl Pts',(3.79119020482575,-18.5647720089771,2.15231139165694));
#81477=CARTESIAN_POINT('Ctrl Pts',(3.79893297411376,-18.5670759749598,2.1463313197106));
#81478=CARTESIAN_POINT('Ctrl Pts',(3.80632114933958,-18.5691671180339,2.14035234406015));
#81479=CARTESIAN_POINT('Ctrl Pts',(3.80945469991699,-18.5700540356269,2.13781647802705));
#81480=CARTESIAN_POINT('Ctrl Pts',(3.81252449773391,-18.5709027096732,2.13528080883013));
#81481=CARTESIAN_POINT('Ctrl Pts',(3.81553100219335,-18.571713764473,2.13274675851501));
#81482=CARTESIAN_POINT('Ctrl Pts',(3.8160401777717,-18.5718511230907,2.13231759682503));
#81483=CARTESIAN_POINT('Ctrl Pts',(3.81654753806618,-18.5719874027859,2.13188848151232));
#81484=CARTESIAN_POINT('Ctrl Pts',(3.81705308543795,-18.5721226066858,2.13145941941345));
#81485=CARTESIAN_POINT('Ctrl Pts',(3.81733124428043,-18.5721969976577,2.13122334377853));
#81486=CARTESIAN_POINT('Ctrl Pts',(3.81760298733007,-18.5722694927627,2.13099226077464));
#81487=CARTESIAN_POINT('Ctrl Pts',(3.81786543179076,-18.5723393509092,2.13076869253328));
#81488=CARTESIAN_POINT('Ctrl Pts',(3.81964637454033,-18.5728134068644,2.12925156301398));
#81489=CARTESIAN_POINT('Ctrl Pts',(3.82107546829223,-18.5731881952949,2.12802006423603));
#81490=CARTESIAN_POINT('Ctrl Pts',(3.82282441905364,-18.5736398446241,2.12649540116583));
#81491=CARTESIAN_POINT('Ctrl Pts',(3.82355222464133,-18.5738277932575,2.12586093030117));
#81492=CARTESIAN_POINT('Ctrl Pts',(3.82433507104321,-18.574028724121,2.12517540037968));
#81493=CARTESIAN_POINT('Ctrl Pts',(3.82521946282455,-18.5742535657944,2.12439558589974));
#81494=CARTESIAN_POINT('Ctrl Pts',(3.82562558266263,-18.574356814904,2.12403748880182));
#81495=CARTESIAN_POINT('Ctrl Pts',(3.82605309574868,-18.5744650878723,2.12365949439501));
#81496=CARTESIAN_POINT('Ctrl Pts',(3.82650638208159,-18.5745793301371,2.12325732390271));
#81497=CARTESIAN_POINT('Ctrl Pts',(3.82680114447219,-18.5746536194342,2.1229958010481));
#81498=CARTESIAN_POINT('Ctrl Pts',(3.82710680368985,-18.5747304313617,2.12272405375829));
#81499=CARTESIAN_POINT('Ctrl Pts',(3.82742454124706,-18.5748100050847,2.12244088867393));
#81500=CARTESIAN_POINT('Ctrl Pts',(3.82766950334125,-18.5748713530286,2.12222258048061));
#81501=CARTESIAN_POINT('Ctrl Pts',(3.82791424023572,-18.5749324874447,2.122004082586));
#81502=CARTESIAN_POINT('Ctrl Pts',(3.82815850400271,-18.5749933462999,2.12178561640277));
#81503=CARTESIAN_POINT('Ctrl Pts',(3.83453725872146,-18.5765826270799,2.11608054514195));
#81504=CARTESIAN_POINT('Ctrl Pts',(3.84064962774462,-18.5779981016353,2.11034704654695));
#81505=CARTESIAN_POINT('Ctrl Pts',(3.84649530522882,-18.5792406016356,2.10459310610884));
#81506=CARTESIAN_POINT('Ctrl Pts',(3.85801299017752,-18.5816886880363,2.09325616982407));
#81507=CARTESIAN_POINT('Ctrl Pts',(3.86849909477289,-18.5834662492265,2.08183660805855));
#81508=CARTESIAN_POINT('Ctrl Pts',(3.87795597733478,-18.5845827583383,2.07038887555791));
#81509=CARTESIAN_POINT('Ctrl Pts',(3.89182600413462,-18.5862202970516,2.05359894975076));
#81510=CARTESIAN_POINT('Ctrl Pts',(3.9034754532728,-18.5864319067783,2.03675151545631));
#81511=CARTESIAN_POINT('Ctrl Pts',(3.91286084283373,-18.5852514849807,2.02007879637055));
#81512=CARTESIAN_POINT('Ctrl Pts',(3.92152399525822,-18.584161900591,2.00468909881638));
#81513=CARTESIAN_POINT('Ctrl Pts',(3.92825680658283,-18.5818861450572,1.98944950741741));
#81514=CARTESIAN_POINT('Ctrl Pts',(3.9330579411577,-18.5784837796564,1.97454056755214));
#81515=CARTESIAN_POINT('Ctrl Pts',(3.93739051868325,-18.5754134612474,1.96108663561528));
#81516=CARTESIAN_POINT('Ctrl Pts',(3.94015054802317,-18.5714255692593,1.9479005209682));
#81517=CARTESIAN_POINT('Ctrl Pts',(3.94136360670749,-18.5665912520027,1.93512016333239));
#81518=CARTESIAN_POINT('Ctrl Pts',(3.94184262224495,-18.5646822651509,1.93007342490078));
#81519=CARTESIAN_POINT('Ctrl Pts',(3.94208069165379,-18.5626416312864,1.92509013935795));
#81520=CARTESIAN_POINT('Ctrl Pts',(3.94208068347,-18.5604754053606,1.9201799813874));
#81521=CARTESIAN_POINT('Origin',(2.225,-18.2859995693,2.04127093829));
#81522=CARTESIAN_POINT('',(3.97419901637,-18.4921598488,2.25921115747));
#81523=CARTESIAN_POINT('Ctrl Pts',(-3.59839802628,-18.4921598689,2.25921118379));
#81524=CARTESIAN_POINT('Ctrl Pts',(-3.56014406419,-18.5158046533,2.23684443014));
#81525=CARTESIAN_POINT('Ctrl Pts',(-3.52188921689,-18.5466712915,2.22211108998));
#81526=CARTESIAN_POINT('Ctrl Pts',(-3.48587211043,-18.5833900444,2.21633482189));
#81527=CARTESIAN_POINT('Ctrl Pts',(-3.4227530696,-18.6640035122,2.22340624095));
#81528=CARTESIAN_POINT('Ctrl Pts',(-3.38341089028,-18.7492623846,2.26482686261));
#81529=CARTESIAN_POINT('Ctrl Pts',(-3.37119264491,-18.7906308404,2.29343157878));
#81530=CARTESIAN_POINT('Ctrl Pts',(-3.36718144281,-18.8281878313,2.32816826251));
#81531=CARTESIAN_POINT('Ctrl Pts',(-3.37113078303,-18.8600780864,2.36677043789));
#81532=CARTESIAN_POINT('Ctrl Pts',(-3.64436692045,-18.5117847779,2.24064705327));
#81533=CARTESIAN_POINT('Ctrl Pts',(-3.60405930901,-18.5336245127,2.21595343871));
#81534=CARTESIAN_POINT('Ctrl Pts',(-3.56375058165,-18.5638766801,2.19877465942));
#81535=CARTESIAN_POINT('Ctrl Pts',(-3.52595626142,-18.6011845215,2.19066396874));
#81536=CARTESIAN_POINT('Ctrl Pts',(-3.46037996228,-18.6849787943,2.19362798662));
#81537=CARTESIAN_POINT('Ctrl Pts',(-3.42131019803,-18.7762049571,2.23225829761));
#81538=CARTESIAN_POINT('Ctrl Pts',(-3.41004989653,-18.8209521428,2.25985117454));
#81539=CARTESIAN_POINT('Ctrl Pts',(-3.40781475601,-18.8618879807,2.29389287788));
#81540=CARTESIAN_POINT('Ctrl Pts',(-3.41419637926,-18.896848952,2.3319871249));
#81541=CARTESIAN_POINT('Ctrl Pts',(-3.68942267786,-18.5300289855,2.21919802164));
#81542=CARTESIAN_POINT('Ctrl Pts',(-3.64682650884,-18.549477242,2.19249708165));
#81543=CARTESIAN_POINT('Ctrl Pts',(-3.60422892213,-18.5786239197,2.17300240599));
#81544=CARTESIAN_POINT('Ctrl Pts',(-3.56446501193,-18.6161750191,2.16250612538));
#81545=CARTESIAN_POINT('Ctrl Pts',(-3.49621412217,-18.7027600572,2.16096091912));
#81546=CARTESIAN_POINT('Ctrl Pts',(-3.4575770292,-18.8000544061,2.19593478233));
#81547=CARTESIAN_POINT('Ctrl Pts',(-3.44746147233,-18.8483268457,2.22200085189));
#81548=CARTESIAN_POINT('Ctrl Pts',(-3.44727650114,-18.8928262827,2.25478702366));
#81549=CARTESIAN_POINT('Ctrl Pts',(-3.45640650501,-18.9310329775,2.29179836087));
#81550=CARTESIAN_POINT('Ctrl Pts',(-3.73299942942,-18.5464475453,2.19473372054));
#81551=CARTESIAN_POINT('Ctrl Pts',(-3.68788926215,-18.5629624494,2.16652139764));
#81552=CARTESIAN_POINT('Ctrl Pts',(-3.64277730184,-18.5905259818,2.14497410893));
#81553=CARTESIAN_POINT('Ctrl Pts',(-3.60086046205,-18.6279613042,2.13211990982));
#81554=CARTESIAN_POINT('Ctrl Pts',(-3.52973391166,-18.716878496,2.12570951285));
#81555=CARTESIAN_POINT('Ctrl Pts',(-3.49169746784,-18.8202109654,2.15601350401));
#81556=CARTESIAN_POINT('Ctrl Pts',(-3.48291402379,-18.8720796182,2.17992329081));
#81557=CARTESIAN_POINT('Ctrl Pts',(-3.48504860923,-18.9202474297,2.21075381154));
#81558=CARTESIAN_POINT('Ctrl Pts',(-3.49723105271,-18.9617959389,2.2459600962));
#81559=CARTESIAN_POINT('Ctrl Pts',(-3.82298172564,-18.5768059901,2.13424066669));
#81560=CARTESIAN_POINT('Ctrl Pts',(-3.77156381879,-18.5854424673,2.10496507054));
#81561=CARTESIAN_POINT('Ctrl Pts',(-3.72014291975,-18.60813878,2.08044622543));
#81562=CARTESIAN_POINT('Ctrl Pts',(-3.67286687834,-18.6441962696,2.06309541364));
#81563=CARTESIAN_POINT('Ctrl Pts',(-3.59477049484,-18.736716632,2.04570253954));
#81564=CARTESIAN_POINT('Ctrl Pts',(-3.55869501022,-18.8530757831,2.06267614809));
#81565=CARTESIAN_POINT('Ctrl Pts',(-3.5535101442,-18.9130111236,2.07975240645));
#81566=CARTESIAN_POINT('Ctrl Pts',(-3.56165956977,-18.9695241648,2.10386975363));
#81567=CARTESIAN_POINT('Ctrl Pts',(-3.58153023859,-19.0186783852,2.13261506243));
#81568=CARTESIAN_POINT('Ctrl Pts',(-3.89478846084,-18.5899476448,2.05800806562));
#81569=CARTESIAN_POINT('Ctrl Pts',(-3.83630626947,-18.590413213,2.03451887228));
#81570=CARTESIAN_POINT('Ctrl Pts',(-3.77781929644,-18.6073285136,2.01213169523));
#81571=CARTESIAN_POINT('Ctrl Pts',(-3.72460903492,-18.6406872183,1.99301884559));
#81572=CARTESIAN_POINT('Ctrl Pts',(-3.63909548341,-18.7337132711,1.96507082573));
#81573=CARTESIAN_POINT('Ctrl Pts',(-3.60591816557,-18.8594295314,1.9603907779));
#81574=CARTESIAN_POINT('Ctrl Pts',(-3.6051532526,-18.9255461021,1.96459768824));
#81575=CARTESIAN_POINT('Ctrl Pts',(-3.62031734938,-18.9884767792,1.97487408281));
#81576=CARTESIAN_POINT('Ctrl Pts',(-3.64880183242,-19.0433013389,1.98977942023));
#81577=CARTESIAN_POINT('Ctrl Pts',(-3.92614909738,-18.5904810042,2.0121443256));
#81578=CARTESIAN_POINT('Ctrl Pts',(-3.86354641755,-18.5867461784,1.99488079923));
#81579=CARTESIAN_POINT('Ctrl Pts',(-3.80093767134,-18.6004023618,1.97610614456));
#81580=CARTESIAN_POINT('Ctrl Pts',(-3.74429549879,-18.6318988452,1.95751630482));
#81581=CARTESIAN_POINT('Ctrl Pts',(-3.65462232559,-18.7240449536,1.92457929667));
#81582=CARTESIAN_POINT('Ctrl Pts',(-3.62341697818,-18.8532013091,1.90495660993));
#81583=CARTESIAN_POINT('Ctrl Pts',(-3.62537876376,-18.9217952194,1.89971595229));
#81584=CARTESIAN_POINT('Ctrl Pts',(-3.64471917587,-18.9873022527,1.89951609703));
#81585=CARTESIAN_POINT('Ctrl Pts',(-3.67818178874,-19.0443009521,1.90384525985));
#81586=CARTESIAN_POINT('Ctrl Pts',(-3.94208066889,-18.5798348566,1.96406190215));
#81587=CARTESIAN_POINT('Ctrl Pts',(-3.87720137211,-18.5763831337,1.95623791132));
#81588=CARTESIAN_POINT('Ctrl Pts',(-3.81231524539,-18.5900964858,1.94390265508));
#81589=CARTESIAN_POINT('Ctrl Pts',(-3.7537820072,-18.6214034822,1.92779936516));
#81590=CARTESIAN_POINT('Ctrl Pts',(-3.66183896524,-18.712539831,1.89147909198));
#81591=CARTESIAN_POINT('Ctrl Pts',(-3.63176679768,-18.8392500191,1.8541374553));
#81592=CARTESIAN_POINT('Ctrl Pts',(-3.6352563839,-18.9062182215,1.8370102935));
#81593=CARTESIAN_POINT('Ctrl Pts',(-3.65691133475,-18.9696900169,1.8232464184));
#81594=CARTESIAN_POINT('Ctrl Pts',(-3.69310715296,-19.0243533592,1.81375388105));
#81595=CARTESIAN_POINT('Ctrl Pts',(-3.94208066889,-18.5604753986,1.92017998437));
#81596=CARTESIAN_POINT('Ctrl Pts',(-3.87720137211,-18.5604753986,1.92017998437));
#81597=CARTESIAN_POINT('Ctrl Pts',(-3.81231524539,-18.5765098851,1.91310602353));
#81598=CARTESIAN_POINT('Ctrl Pts',(-3.7537820072,-18.6086631321,1.89892092257));
#81599=CARTESIAN_POINT('Ctrl Pts',(-3.66183896524,-18.6983642163,1.85934734744));
#81600=CARTESIAN_POINT('Ctrl Pts',(-3.63176679768,-18.8182205477,1.80647013222));
#81601=CARTESIAN_POINT('Ctrl Pts',(-3.6352563839,-18.8806031007,1.77894871848));
#81602=CARTESIAN_POINT('Ctrl Pts',(-3.65691133475,-18.9388168454,1.75326646482));
#81603=CARTESIAN_POINT('Ctrl Pts',(-3.69310715296,-18.9880798485,1.73153302458));
#81604=CARTESIAN_POINT('Ctrl Pts',(-3.94208066889,-18.5604753986,1.92017998437));
#81605=CARTESIAN_POINT('Ctrl Pts',(-3.94208066889,-18.5657281416406,1.93208633206972));
#81606=CARTESIAN_POINT('Ctrl Pts',(-3.94065119988507,-18.5702315992113,
1.94441093072267));
#81607=CARTESIAN_POINT('Ctrl Pts',(-3.93779591447238,-18.5739224805057,
1.95702353188134));
#81608=CARTESIAN_POINT('Ctrl Pts',(-3.93380262854624,-18.579084396811,1.97466300234372));
#81609=CARTESIAN_POINT('Ctrl Pts',(-3.92702066882058,-18.5826580874444,
1.99286811843331));
#81610=CARTESIAN_POINT('Ctrl Pts',(-3.91744476193116,-18.584517276425,2.01138446283056));
#81611=CARTESIAN_POINT('Ctrl Pts',(-3.91616044782598,-18.5847666295839,
2.01386786232058));
#81612=CARTESIAN_POINT('Ctrl Pts',(-3.91482587460073,-18.5849851799538,
2.0163569188334));
#81613=CARTESIAN_POINT('Ctrl Pts',(-3.91344104111079,-18.5851726554105,
2.01885104891104));
#81614=CARTESIAN_POINT('Ctrl Pts',(-3.90562472234754,-18.5862308100119,
2.03292849278095));
#81615=CARTESIAN_POINT('Ctrl Pts',(-3.89620941410297,-18.5862950059314,
2.04715128243047));
#81616=CARTESIAN_POINT('Ctrl Pts',(-3.88517509792813,-18.5853373319509,
2.06136781888637));
#81617=CARTESIAN_POINT('Ctrl Pts',(-3.88273253357344,-18.5851253405333,
2.06451480186602));
#81618=CARTESIAN_POINT('Ctrl Pts',(-3.88021078432442,-18.5848634083244,
2.0676614064857));
#81619=CARTESIAN_POINT('Ctrl Pts',(-3.87760986289313,-18.5845514594247,
2.07080589867206));
#81620=CARTESIAN_POINT('Ctrl Pts',(-3.8704345540156,-18.5836908683731,2.07948078689767));
#81621=CARTESIAN_POINT('Ctrl Pts',(-3.86265400859441,-18.5824497275828,
2.0881389299267));
#81622=CARTESIAN_POINT('Ctrl Pts',(-3.85428553574451,-18.5808265237171,
2.09675428436504));
#81623=CARTESIAN_POINT('Ctrl Pts',(-3.85010129931957,-18.5800149217843,
2.10106196158421));
#81624=CARTESIAN_POINT('Ctrl Pts',(-3.84577002421308,-18.5791077857091,
2.10535901184153));
#81625=CARTESIAN_POINT('Ctrl Pts',(-3.84129246804519,-18.5781049463998,
2.10964170600792));
#81626=CARTESIAN_POINT('Ctrl Pts',(-3.83919880205726,-18.5776360275355,
2.11164425623325));
#81627=CARTESIAN_POINT('Ctrl Pts',(-3.83677005848046,-18.5770763899686,
2.11392889126115));
#81628=CARTESIAN_POINT('Ctrl Pts',(-3.83442653236003,-18.5765193810966,
2.11609139417422));
#81629=CARTESIAN_POINT('Ctrl Pts',(-3.83175814641062,-18.5758851595983,
2.11855366346087));
#81630=CARTESIAN_POINT('Ctrl Pts',(-3.82920065543799,-18.5752546318829,
2.12085758181794));
#81631=CARTESIAN_POINT('Ctrl Pts',(-3.82742157038535,-18.5748090672012,
2.12244296878305));
#81632=CARTESIAN_POINT('Ctrl Pts',(-3.82259073759956,-18.5735992045984,
2.12674784409964));
#81633=CARTESIAN_POINT('Ctrl Pts',(-3.81757758328911,-18.5722826572169,
2.13106343755174));
#81634=CARTESIAN_POINT('Ctrl Pts',(-3.81237820924604,-18.5708553930854,
2.13538342234656));
#81635=CARTESIAN_POINT('Ctrl Pts',(-3.79392163837841,-18.5657889367444,
2.15071836552475));
#81636=CARTESIAN_POINT('Ctrl Pts',(-3.77311289509145,-18.5593227106784,
2.16610956974355));
#81637=CARTESIAN_POINT('Ctrl Pts',(-3.74993785221099,-18.5513665587327,
2.1812003601061));
#81638=CARTESIAN_POINT('Ctrl Pts',(-3.72815451567081,-18.5438881891654,
2.19538491919496));
#81639=CARTESIAN_POINT('Ctrl Pts',(-3.70428289127466,-18.5350948765864,
2.20930315692247));
#81640=CARTESIAN_POINT('Ctrl Pts',(-3.67832404689165,-18.5249399314279,
2.22267762482839));
#81641=CARTESIAN_POINT('Ctrl Pts',(-3.65783608400393,-18.5169251624935,
2.23323339526471));
#81642=CARTESIAN_POINT('Ctrl Pts',(-3.6360461079442,-18.5080622310107,2.24345293909897));
#81643=CARTESIAN_POINT('Ctrl Pts',(-3.61296616496511,-18.4983387101615,
2.25319561885508));
#81644=CARTESIAN_POINT('Ctrl Pts',(-3.60816568166547,-18.4963162788455,
2.25522203510339));
#81645=CARTESIAN_POINT('Ctrl Pts',(-3.60330951103741,-18.4942566687393,
2.25722772150755));
#81646=CARTESIAN_POINT('Ctrl Pts',(-3.59839802627999,-18.4921598714318,
2.25921118139502));
#81647=CARTESIAN_POINT('Origin',(2.225,-18.2859995693,2.04127093829));
#81648=CARTESIAN_POINT('',(-4.35,-18.4921598488,2.25921115747));
#81649=CARTESIAN_POINT('',(-3.97419901637,-18.4921598488,2.25921115747));
#81650=CARTESIAN_POINT('Origin',(-4.35,-18.2859995693,2.04127093829));
#81651=CARTESIAN_POINT('Origin',(0.,-14.2790683411,6.24457983432));
#81652=CARTESIAN_POINT('',(-4.35,-14.5682305188,5.97104723161));
#81653=CARTESIAN_POINT('',(2.225,-14.5682305188,5.97104723161));
#81654=CARTESIAN_POINT('',(-4.35,-18.9225141731,1.85211801911));
#81655=CARTESIAN_POINT('Origin',(2.225,-13.881029587,5.24457983432));
#81656=CARTESIAN_POINT('',(-4.35,-13.881029587,6.24457983432));
#81657=CARTESIAN_POINT('',(0.,-13.881029587,6.24457983432));
#81658=CARTESIAN_POINT('Origin',(-4.35,-13.881029587,5.24457983432));
#81659=CARTESIAN_POINT('Origin',(0.,-7.56172990606,6.24457983432));
#81660=CARTESIAN_POINT('',(-4.35,-7.67105043563,6.24457983432));
#81661=CARTESIAN_POINT('',(2.225,-7.67105043563,6.24457983432));
#81662=CARTESIAN_POINT('',(-4.35,-1.95899712601,6.24457983432));
#81663=CARTESIAN_POINT('Origin',(2.225,-7.67105043563,5.74457983432));
#81664=CARTESIAN_POINT('',(-4.35,-7.46238442811,6.19895687742));
#81665=CARTESIAN_POINT('',(0.,-7.46238442811,6.19895687742));
#81666=CARTESIAN_POINT('Origin',(-4.35,-7.67105043563,5.74457983432));
#81667=CARTESIAN_POINT('Origin',(0.,-2.35008265971,3.85120710557));
#81668=CARTESIAN_POINT('',(-4.35,-2.44942813767,3.89683006246));
#81669=CARTESIAN_POINT('',(2.225,-2.44942813767,3.89683006246));
#81670=CARTESIAN_POINT('',(-4.35,4.63581368472,0.643036443538));
#81671=CARTESIAN_POINT('Origin',(2.225,-2.24076213014,4.35120710557));
#81672=CARTESIAN_POINT('',(-4.35,-2.24076213014,3.85120710557));
#81673=CARTESIAN_POINT('',(0.,-2.24076213014,3.85120710557));
#81674=CARTESIAN_POINT('Origin',(-4.35,-2.24076213014,4.35120710557));
#81675=CARTESIAN_POINT('Origin',(0.,2.74061906787,3.85120710557));
#81676=CARTESIAN_POINT('',(-4.35,2.48275227055,3.85120710557));
#81677=CARTESIAN_POINT('',(2.225,2.48275227055,3.85120710557));
#81678=CARTESIAN_POINT('',(-4.35,-1.95899712601,3.85120710557));
#81679=CARTESIAN_POINT('Origin',(2.225,2.48275227055,4.35120710557));
#81680=CARTESIAN_POINT('',(-4.35,2.89013084681,4.06130592308));
#81681=CARTESIAN_POINT('',(0.,2.89013084681,4.06130592308));
#81682=CARTESIAN_POINT('Origin',(-4.35,2.48275227055,4.35120710557));
#81683=CARTESIAN_POINT('Origin',(0.,4.27111742671,6.00191320834));
#81684=CARTESIAN_POINT('',(-4.35,4.24121507093,5.95989344484));
#81685=CARTESIAN_POINT('',(2.225,4.24121507093,5.95989344484));
#81686=CARTESIAN_POINT('',(-4.35,0.250890909306,0.352560070814));
#81687=CARTESIAN_POINT('Origin',(4.35,4.32269078618,5.90191320834));
#81688=CARTESIAN_POINT('Origin',(4.35,4.32269078618,5.90191320834));
#81689=CARTESIAN_POINT('Origin',(0.,4.8773238354,6.00191320834));
#81690=CARTESIAN_POINT('',(-4.35,4.7773238354,6.00191320834));
#81691=CARTESIAN_POINT('',(2.225,4.7773238354,6.00191320834));
#81692=CARTESIAN_POINT('',(-4.35,4.32269078618,6.00191320834));
#81693=CARTESIAN_POINT('',(-4.35,-1.95899712601,6.00191320834));
#81694=CARTESIAN_POINT('',(2.225,4.32269078618,6.00191320834));
#81695=CARTESIAN_POINT('Origin',(4.35,4.7773238354,5.90191320834));
#81696=CARTESIAN_POINT('Origin',(4.35,4.7773238354,5.90191320834));
#81697=CARTESIAN_POINT('Origin',(0.,4.8773238354,4.12878088412));
#81698=CARTESIAN_POINT('',(-4.35,4.8773238354,4.22878088412));
#81699=CARTESIAN_POINT('',(2.225,4.8773238354,4.22878088412));
#81700=CARTESIAN_POINT('',(-4.35,4.8773238354,5.90191320834));
#81701=CARTESIAN_POINT('',(-4.35,4.8773238354,0.294579834316));
#81702=CARTESIAN_POINT('',(2.225,4.8773238354,5.90191320834));
#81703=CARTESIAN_POINT('Origin',(2.225,4.9773238354,4.22878088412));
#81704=CARTESIAN_POINT('',(-4.35,4.9773238354,4.12878088412));
#81705=CARTESIAN_POINT('',(0.,4.9773238354,4.12878088412));
#81706=CARTESIAN_POINT('Origin',(-4.35,4.9773238354,4.22878088412));
#81707=CARTESIAN_POINT('Origin',(0.,15.277455061,4.12878088412));
#81708=CARTESIAN_POINT('',(-4.35,15.177455061,4.12878088412));
#81709=CARTESIAN_POINT('',(2.225,15.177455061,4.12878088412));
#81710=CARTESIAN_POINT('',(-4.35,-1.95899712601,4.12878088412));
#81711=CARTESIAN_POINT('Origin',(4.35,15.177455061,4.02878088412));
#81712=CARTESIAN_POINT('Origin',(4.35,15.177455061,4.02878088412));
#81713=CARTESIAN_POINT('Origin',(0.,15.277455061,-4.77121911588));
#81714=CARTESIAN_POINT('',(-4.35,15.277455061,-4.67121911588));
#81715=CARTESIAN_POINT('',(2.225,15.277455061,-4.67121911588));
#81716=CARTESIAN_POINT('',(-4.35,15.277455061,4.02878088412));
#81717=CARTESIAN_POINT('',(-4.35,15.277455061,0.294579834316));
#81718=CARTESIAN_POINT('',(2.225,15.277455061,4.02878088412));
#81719=CARTESIAN_POINT('Origin',(4.35,15.177455061,-4.67121911588));
#81720=CARTESIAN_POINT('Origin',(4.35,15.177455061,-4.67121911588));
#81721=CARTESIAN_POINT('Origin',(0.,15.277455061,-4.77121911588));
#81722=CARTESIAN_POINT('',(-4.35,4.9773238354,-4.77121911588));
#81723=CARTESIAN_POINT('',(2.225,4.9773238354,-4.77121911588));
#81724=CARTESIAN_POINT('',(-4.35,15.177455061,-4.77121911588));
#81725=CARTESIAN_POINT('',(-4.35,-1.95899712601,-4.77121911588));
#81726=CARTESIAN_POINT('',(2.225,15.177455061,-4.77121911588));
#81727=CARTESIAN_POINT('Origin',(2.225,4.9773238354,-4.87121911588));
#81728=CARTESIAN_POINT('',(-4.35,4.8773238354,-4.87121911588));
#81729=CARTESIAN_POINT('',(0.,4.8773238354,-4.87121911588));
#81730=CARTESIAN_POINT('Origin',(-4.35,4.9773238354,-4.87121911588));
#81731=CARTESIAN_POINT('Origin',(0.,4.8773238354,4.12878088412));
#81732=CARTESIAN_POINT('',(-4.35,4.8773238354,0.294579834316));
#81733=CARTESIAN_POINT('Origin',(0.,-9.17423561284,0.47366156039));
#81734=CARTESIAN_POINT('',(4.35,-11.8242356128,0.47366156039));
#81735=CARTESIAN_POINT('Origin',(4.35,-9.17423561284,0.473661560389999));
#81736=CARTESIAN_POINT('',(0.,-11.82423561284,0.47366156039));
#81737=CARTESIAN_POINT('Origin',(-4.35,-21.2594877202,0.729452270839));
#81738=CARTESIAN_POINT('',(-4.45,-18.4689834555,1.96054363567));
#81739=CARTESIAN_POINT('Origin',(-4.35,-18.4689834555,1.96054363567));
#81740=CARTESIAN_POINT('',(-4.45,-18.3216303794,1.54889979527));
#81741=CARTESIAN_POINT('Origin',(-4.45,-21.2594877202,0.729452270839));
#81742=CARTESIAN_POINT('Origin',(-4.35,-18.3216303794,1.54889979527));
#81743=CARTESIAN_POINT('Ctrl Pts',(-3.94234877308934,-18.4179622929748,
1.5220634491669));
#81744=CARTESIAN_POINT('Ctrl Pts',(-3.87741592322529,-18.4179021372523,
1.52206354967647));
#81745=CARTESIAN_POINT('Ctrl Pts',(-3.81246043986878,-18.4347523597789,
1.51735270773294));
#81746=CARTESIAN_POINT('Ctrl Pts',(-3.75385806626735,-18.4686084523042,
1.50790595663289));
#81747=CARTESIAN_POINT('Ctrl Pts',(-3.66185147225803,-18.5630744293574,
1.48156577864178));
#81748=CARTESIAN_POINT('Ctrl Pts',(-3.63176687268071,-18.6893211886786,
1.44638791408526));
#81749=CARTESIAN_POINT('Ctrl Pts',(-3.63525645057377,-18.7550039506979,
1.42809073665793));
#81750=CARTESIAN_POINT('Ctrl Pts',(-3.65691138925993,-18.8162985856091,
1.41102067506232));
#81751=CARTESIAN_POINT('Ctrl Pts',(-3.69310719334021,-18.8681699604421,
1.39657949980758));
#81752=CARTESIAN_POINT('Ctrl Pts',(-3.94236571798829,-18.4133876700544,
1.50564227215289));
#81753=CARTESIAN_POINT('Ctrl Pts',(-3.87742949734126,-18.4156210030371,
1.51388530750485));
#81754=CARTESIAN_POINT('Ctrl Pts',(-3.8124706399661,-18.4339647887765,1.51454343666174));
#81755=CARTESIAN_POINT('Ctrl Pts',(-3.75386547213153,-18.4682850893703,
1.50676707768882));
#81756=CARTESIAN_POINT('Ctrl Pts',(-3.66185555985532,-18.5615234559633,
1.47602152543541));
#81757=CARTESIAN_POINT('Ctrl Pts',(-3.63177274765737,-18.682852077315,1.4231810522504));
#81758=CARTESIAN_POINT('Ctrl Pts',(-3.63526465905675,-18.7453003527305,
1.39326767740239));
#81759=CARTESIAN_POINT('Ctrl Pts',(-3.65692311167227,-18.8029268266872,
1.36302496574797));
#81760=CARTESIAN_POINT('Ctrl Pts',(-3.69312305426809,-18.8510626926684,
1.33517080589476));
#81761=CARTESIAN_POINT('Ctrl Pts',(-3.93117743481258,-18.4053199263241,
1.49021851431677));
#81762=CARTESIAN_POINT('Ctrl Pts',(-3.86848432428731,-18.4133496508806,
1.50572009052338));
#81763=CARTESIAN_POINT('Ctrl Pts',(-3.80577072397423,-18.4356439814143,
1.51105797007258));
#81764=CARTESIAN_POINT('Ctrl Pts',(-3.74902487427037,-18.4714835809575,
1.50465788542018));
#81765=CARTESIAN_POINT('Ctrl Pts',(-3.65922237266646,-18.5627831102452,
1.46971354377953));
#81766=CARTESIAN_POINT('Ctrl Pts',(-3.62794841541813,-18.6740098368393,
1.40067791306863));
#81767=CARTESIAN_POINT('Ctrl Pts',(-3.62988637637911,-18.7297933802063,
1.36011859423275));
#81768=CARTESIAN_POINT('Ctrl Pts',(-3.64920524301539,-18.7800386429644,
1.31775397033819));
#81769=CARTESIAN_POINT('Ctrl Pts',(-3.68265005904169,-18.8209194717089,
1.277483839591));
#81770=CARTESIAN_POINT('Ctrl Pts',(-3.90937039764836,-18.3946473544159,
1.47823990790765));
#81771=CARTESIAN_POINT('Ctrl Pts',(-3.85079941235044,-18.4100260311796,
1.4954773509941));
#81772=CARTESIAN_POINT('Ctrl Pts',(-3.79221048551906,-18.4371226818621,
1.50112267759752));
#81773=CARTESIAN_POINT('Ctrl Pts',(-3.73888775605576,-18.4745486886345,
1.49356057393109));
#81774=CARTESIAN_POINT('Ctrl Pts',(-3.65317282634548,-18.5626874259432,
1.45356159969605));
#81775=CARTESIAN_POINT('Ctrl Pts',(-3.6197569336771,-18.6607011526531,1.37482011528626));
#81776=CARTESIAN_POINT('Ctrl Pts',(-3.61885954013509,-18.7079919198437,
1.32845104766779));
#81777=CARTESIAN_POINT('Ctrl Pts',(-3.63388281316495,-18.7490375736454,
1.27962425360384));
#81778=CARTESIAN_POINT('Ctrl Pts',(-3.66223622907347,-18.7810400637854,
1.23262277310423));
#81779=CARTESIAN_POINT('Ctrl Pts',(-3.88313625536304,-18.3833905207368,
1.46911853484485));
#81780=CARTESIAN_POINT('Ctrl Pts',(-3.82827635921413,-18.4040707835055,
1.48560034168476));
#81781=CARTESIAN_POINT('Ctrl Pts',(-3.77340110703683,-18.4341185642061,
1.48981511758575));
#81782=CARTESIAN_POINT('Ctrl Pts',(-3.72318353452304,-18.4717817689888,
1.48031522313803));
#81783=CARTESIAN_POINT('Ctrl Pts',(-3.64128193973745,-18.5553892025893,
1.4356866604964));
#81784=CARTESIAN_POINT('Ctrl Pts',(-3.60614533962705,-18.6412407365273,
1.35102616050676));
#81785=CARTESIAN_POINT('Ctrl Pts',(-3.60279817951113,-18.6811249203593,
1.30143857220328));
#81786=CARTESIAN_POINT('Ctrl Pts',(-3.61399030710223,-18.7143667021278,
1.24912958467003));
#81787=CARTESIAN_POINT('Ctrl Pts',(-3.63767337026233,-18.738937433864,1.19843010357245));
#81788=CARTESIAN_POINT('Ctrl Pts',(-3.85356722871327,-18.3718068169226,
1.46239916841677));
#81789=CARTESIAN_POINT('Ctrl Pts',(-3.80215086093377,-18.3963222194477,
1.47671313353459));
#81790=CARTESIAN_POINT('Ctrl Pts',(-3.75072128784765,-18.4280665581311,
1.47861300783342));
#81791=CARTESIAN_POINT('Ctrl Pts',(-3.70340064135175,-18.4651002965507,
1.46690668481873));
#81792=CARTESIAN_POINT('Ctrl Pts',(-3.62512643672596,-18.5433562230935,
1.41831938308649));
#81793=CARTESIAN_POINT('Ctrl Pts',(-3.58854128012704,-18.6178411571792,
1.3304346488623));
#81794=CARTESIAN_POINT('Ctrl Pts',(-3.58299778663471,-18.6510735894616,
1.27938625857796));
#81795=CARTESIAN_POINT('Ctrl Pts',(-3.59067473503819,-18.6774630701226,
1.22558481182393));
#81796=CARTESIAN_POINT('Ctrl Pts',(-3.60998517910906,-18.6955883056329,
1.17321662092078));
#81797=CARTESIAN_POINT('Ctrl Pts',(-3.85341043799,-18.3719297862815,1.46247080900171));
#81798=CARTESIAN_POINT('Ctrl Pts',(-3.87059142535003,-18.3786553513643,
1.46638491177223));
#81799=CARTESIAN_POINT('Ctrl Pts',(-3.88527563788033,-18.3848432456902,
1.47104121504505));
#81800=CARTESIAN_POINT('Ctrl Pts',(-3.89746307558087,-18.3903663596056,
1.47626808714481));
#81801=CARTESIAN_POINT('Ctrl Pts',(-3.90983341714612,-18.3959723620578,
1.48157340191077));
#81802=CARTESIAN_POINT('Ctrl Pts',(-3.91963148047731,-18.4008934150417,
1.48746561968176));
#81803=CARTESIAN_POINT('Ctrl Pts',(-3.92685726557444,-18.4050492008162,
1.49375181041533));
#81804=CARTESIAN_POINT('Ctrl Pts',(-3.93425454899559,-18.4093036208963,
1.50018719893999));
#81805=CARTESIAN_POINT('Ctrl Pts',(-3.93895600318521,-18.4127561162088,
1.50703457317492));
#81806=CARTESIAN_POINT('Ctrl Pts',(-3.94096162814328,-18.4153751057879,
1.51408706377056));
#81807=CARTESIAN_POINT('Ctrl Pts',(-3.94170771372341,-18.4163493608956,
1.51671056599425));
#81808=CARTESIAN_POINT('Ctrl Pts',(-3.94208074657565,-18.4172087969225,
1.51936252321673));
#81809=CARTESIAN_POINT('Ctrl Pts',(-3.9420807267,-18.4179535709002,1.52203266331995));
#81810=CARTESIAN_POINT('Origin',(-2.225,-18.3216303794,1.54889979527));
#81811=CARTESIAN_POINT('',(-4.35,-18.3719297863,1.46247080897));
#81812=CARTESIAN_POINT('Origin',(-4.35,-18.3216303794,1.54889979527));
#81813=CARTESIAN_POINT('',(0.,-18.3719297863,1.46247080897));
#81814=CARTESIAN_POINT('Origin',(-2.3,-21.2594877202,0.729452270839));
#81815=CARTESIAN_POINT('',(-2.,-17.1183636721,1.08100826706));
#81816=CARTESIAN_POINT('Origin',(-2.3,-17.1183636721,1.08100826706));
#81817=CARTESIAN_POINT('',(-2.,-17.3209666442,-0.597405571358));
#81818=CARTESIAN_POINT('Origin',(-2.,-21.2594877202,0.729452270839));
#81819=CARTESIAN_POINT('Origin',(-2.3,-17.3209666442,-0.597405571358));
#81820=CARTESIAN_POINT('Origin',(-2.,0.,0.));
#81821=CARTESIAN_POINT('',(-2.,-13.3863832983,4.61127046457));
#81822=CARTESIAN_POINT('',(-2.,-16.3982789105,1.76217155265));
#81823=CARTESIAN_POINT('',(-2.,-12.9053426461,4.80274328646));
#81824=CARTESIAN_POINT('Origin',(-2.,-12.9053426461,4.10274328646));
#81825=CARTESIAN_POINT('',(-2.,-9.41827086707,4.80274328646));
#81826=CARTESIAN_POINT('',(-2.,-12.0504559477,4.80274328646));
#81827=CARTESIAN_POINT('',(-2.,-8.76025711822,4.30133994369));
#81828=CARTESIAN_POINT('Origin',(-2.,-8.67423561284,5.09670168568));
#81829=CARTESIAN_POINT('',(-2.,-8.76025711822,-3.35401682291));
#81830=CARTESIAN_POINT('Origin',(-2.,-9.17423561284,0.47366156039));
#81831=CARTESIAN_POINT('',(-2.,-9.41827086707,-3.85542016568));
#81832=CARTESIAN_POINT('Origin',(-2.,-8.67423561284,-4.1493785649));
#81833=CARTESIAN_POINT('',(-2.,-10.0779006799,-3.85542016568));
#81834=CARTESIAN_POINT('',(-2.,-8.20939783898,-3.85542016568));
#81835=CARTESIAN_POINT('',(-2.,-10.371774934,-3.79074521854));
#81836=CARTESIAN_POINT('Origin',(-2.,-10.0779006799,-3.15542016568));
#81837=CARTESIAN_POINT('',(-2.,-17.1551720262,-0.653035235664));
#81838=CARTESIAN_POINT('',(-2.,-13.7337583338,-2.23563518556));
#81839=CARTESIAN_POINT('Origin',(-2.,-17.4910283166,-1.37912101035));
#81840=CARTESIAN_POINT('',(-2.,-12.12423561284,0.47366156039));
#81841=CARTESIAN_POINT('Origin',(-2.,-9.17423561284,0.47366156039));
#81842=CARTESIAN_POINT('Ctrl Pts',(-3.88718266259547,-19.025433934838,-1.22483561091038));
#81843=CARTESIAN_POINT('Ctrl Pts',(-3.77580408384224,-19.0736898839023,
-1.23616597952645));
#81844=CARTESIAN_POINT('Ctrl Pts',(-3.66440778333474,-19.1360641780841,
-1.18720219522702));
#81845=CARTESIAN_POINT('Ctrl Pts',(-3.59323386373744,-19.1955274355822,
-1.07211980399972));
#81846=CARTESIAN_POINT('Ctrl Pts',(-3.59207872644302,-19.2271844940609,
-0.939102859271506));
#81847=CARTESIAN_POINT('Ctrl Pts',(-3.64159979814485,-19.2306078238278,
-0.827755898096201));
#81848=CARTESIAN_POINT('Ctrl Pts',(-3.90640659993754,-19.0359515024118,
-1.22729295147926));
#81849=CARTESIAN_POINT('Ctrl Pts',(-3.78964355915635,-19.0775118594821,
-1.24255434458416));
#81850=CARTESIAN_POINT('Ctrl Pts',(-3.67286110812766,-19.1403096158138,
-1.19644007340445));
#81851=CARTESIAN_POINT('Ctrl Pts',(-3.60013346101267,-19.2091455215151,
-1.0813755662174));
#81852=CARTESIAN_POINT('Ctrl Pts',(-3.60331125265511,-19.2540269422902,
-0.947808006978175));
#81853=CARTESIAN_POINT('Ctrl Pts',(-3.65960588543438,-19.2700026746203,
-0.836975235851294));
#81854=CARTESIAN_POINT('Ctrl Pts',(-3.92284970227234,-19.0467428229707,
-1.23131164661682));
#81855=CARTESIAN_POINT('Ctrl Pts',(-3.80072845787408,-19.0792180125451,
-1.24870207523215));
#81856=CARTESIAN_POINT('Ctrl Pts',(-3.67858607893163,-19.1408694654263,
-1.20498533022795));
#81857=CARTESIAN_POINT('Ctrl Pts',(-3.60441223261194,-19.2195874016009,
-1.09137878321749));
#81858=CARTESIAN_POINT('Ctrl Pts',(-3.61202763612795,-19.2797027732923,
-0.959801768378248));
#81859=CARTESIAN_POINT('Ctrl Pts',(-3.67500679368465,-19.3104167222716,
-0.852040651816825));
#81860=CARTESIAN_POINT('Ctrl Pts',(-3.93558612334475,-19.0576343352439,
-1.23716860991036));
#81861=CARTESIAN_POINT('Ctrl Pts',(-3.80845043726328,-19.0782994500631,
-1.25360431235422));
#81862=CARTESIAN_POINT('Ctrl Pts',(-3.68129195135629,-19.1367502302322,
-1.21109032580039));
#81863=CARTESIAN_POINT('Ctrl Pts',(-3.60588177835506,-19.2256755686209,
-1.10083932805995));
#81864=CARTESIAN_POINT('Ctrl Pts',(-3.61778081899953,-19.303262871619,-0.974970009523419));
#81865=CARTESIAN_POINT('Ctrl Pts',(-3.68693535426574,-19.3511979302931,
-0.873985633650477));
#81866=CARTESIAN_POINT('Ctrl Pts',(-3.94218039631734,-19.0678943136438,
-1.24528320682825));
#81867=CARTESIAN_POINT('Ctrl Pts',(-3.8124009667551,-19.0766778004732,-1.25501049679676));
#81868=CARTESIAN_POINT('Ctrl Pts',(-3.68259785626293,-19.1312303113916,
-1.21075865244405));
#81869=CARTESIAN_POINT('Ctrl Pts',(-3.60654295125758,-19.2294718799634,
-1.10665750700906));
#81870=CARTESIAN_POINT('Ctrl Pts',(-3.62070686959814,-19.3242869156647,
-0.992634050237943));
#81871=CARTESIAN_POINT('Ctrl Pts',(-3.69311133654807,-19.3896139653707,
-0.904376164438057));
#81872=CARTESIAN_POINT('Ctrl Pts',(-3.94217592748915,-19.076683734755,-1.25495360386885));
#81873=CARTESIAN_POINT('Ctrl Pts',(-3.81239828953171,-19.0766457743704,
-1.25497310675431));
#81874=CARTESIAN_POINT('Ctrl Pts',(-3.68259697124399,-19.1285379948036,
-1.20779327228567));
#81875=CARTESIAN_POINT('Ctrl Pts',(-3.60654249737104,-19.2341457609791,
-1.1117975978063));
#81876=CARTESIAN_POINT('Ctrl Pts',(-3.62070488664521,-19.3428206630258,
-1.01302463080287));
#81877=CARTESIAN_POINT('Ctrl Pts',(-3.69310715118846,-19.4225269040689,
-0.940588007021057));
#81878=CARTESIAN_POINT('Ctrl Pts',(-3.94208066889,-19.0766762824804,-1.25494542807784));
#81879=CARTESIAN_POINT('Ctrl Pts',(-3.94208066889,-19.0715553844833,-1.24931250745258));
#81880=CARTESIAN_POINT('Ctrl Pts',(-3.9393205736673,-19.0657379583168,-1.2442116228788));
#81881=CARTESIAN_POINT('Ctrl Pts',(-3.9338003832219,-19.0593444548702,-1.23981507244739));
#81882=CARTESIAN_POINT('Ctrl Pts',(-3.92838645285692,-19.0530740222121,
-1.23550315275601));
#81883=CARTESIAN_POINT('Ctrl Pts',(-3.9203176646309,-19.0462498198137,-1.23186946682268));
#81884=CARTESIAN_POINT('Ctrl Pts',(-3.90959401854385,-19.0390290035994,
-1.22905229461513));
#81885=CARTESIAN_POINT('Ctrl Pts',(-3.90308103832551,-19.0346434585356,
-1.22734129196635));
#81886=CARTESIAN_POINT('Ctrl Pts',(-3.89558875789756,-19.0301124511698,
-1.22593095609068));
#81887=CARTESIAN_POINT('Ctrl Pts',(-3.88711717726,-19.0254782582987,-1.22484599945563));
#81888=CARTESIAN_POINT('Origin',(-2.225,-19.0026826744,-1.32221314666));
#81889=CARTESIAN_POINT('',(-4.35,-19.0254782583,-1.22484599945));
#81890=CARTESIAN_POINT('',(0.,-19.0254782583,-1.22484599945));
#81891=CARTESIAN_POINT('Origin',(-4.35,-19.0026826744,-1.32221314666));
#81892=CARTESIAN_POINT('Origin',(-2.3,-9.41827086707,-3.85542016568));
#81893=CARTESIAN_POINT('',(-2.3,-9.13925764673,-3.96565456539));
#81894=CARTESIAN_POINT('Origin',(-2.3,-9.41827086707,-3.85542016568));
#81895=CARTESIAN_POINT('',(-2.3,-9.41827086707,-4.15542016568));
#81896=CARTESIAN_POINT('Origin',(-2.3,-9.41827086707,-3.85542016568));
#81897=CARTESIAN_POINT('Origin',(-2.3,-9.41827086707,-3.85542016568));
#81898=CARTESIAN_POINT('Ctrl Pts',(3.85357127529058,-18.3718036312809,1.46239723758686));
#81899=CARTESIAN_POINT('Ctrl Pts',(3.80215397592704,-18.3963191316518,1.47671247492689));
#81900=CARTESIAN_POINT('Ctrl Pts',(3.75072320422429,-18.4280638952455,1.47861315152616));
#81901=CARTESIAN_POINT('Ctrl Pts',(3.70340133340925,-18.4650983039147,1.46690700156938));
#81902=CARTESIAN_POINT('Ctrl Pts',(3.62512602082281,-18.5433548310396,1.41831937899194));
#81903=CARTESIAN_POINT('Ctrl Pts',(3.58854039733859,-18.6178399766783,1.33043350136151));
#81904=CARTESIAN_POINT('Ctrl Pts',(3.5829967928236,-18.6510720638893,1.27938501876718));
#81905=CARTESIAN_POINT('Ctrl Pts',(3.59067356313336,-18.6774611898981,1.22558347765477));
#81906=CARTESIAN_POINT('Ctrl Pts',(3.60998378544702,-18.6955860923029,1.17321518442684));
#81907=CARTESIAN_POINT('Ctrl Pts',(3.88315087732857,-18.3833917237588,1.46911854700638));
#81908=CARTESIAN_POINT('Ctrl Pts',(3.82828881190557,-18.4040705718358,1.4856024608897));
#81909=CARTESIAN_POINT('Ctrl Pts',(3.7734110869559,-18.4341180636217,1.48981892272446));
#81910=CARTESIAN_POINT('Ctrl Pts',(3.72319120146361,-18.4717821126652,1.48032002015744));
#81911=CARTESIAN_POINT('Ctrl Pts',(3.64128717554319,-18.5553919914991,1.4356925004318));
#81912=CARTESIAN_POINT('Ctrl Pts',(3.60615060806008,-18.6412476903878,1.35103186316354));
#81913=CARTESIAN_POINT('Ctrl Pts',(3.6028040762687,-18.6811337590432,1.30144459840769));
#81914=CARTESIAN_POINT('Ctrl Pts',(3.6139972125595,-18.7143774757967,1.24913593326059));
#81915=CARTESIAN_POINT('Ctrl Pts',(3.63768153388863,-18.738950023906,1.1984368256642));
#81916=CARTESIAN_POINT('Ctrl Pts',(3.90939559357203,-18.3946540094753,1.4782446449377));
#81917=CARTESIAN_POINT('Ctrl Pts',(3.85082074009429,-18.4100283850775,1.49548402094887));
#81918=CARTESIAN_POINT('Ctrl Pts',(3.7922276215467,-18.4371229831985,1.50113134358345));
#81919=CARTESIAN_POINT('Ctrl Pts',(3.73890110215105,-18.4745494045097,1.49357102698152));
#81920=CARTESIAN_POINT('Ctrl Pts',(3.65318201219449,-18.5626922931479,1.45357539566712));
#81921=CARTESIAN_POINT('Ctrl Pts',(3.61976694585612,-18.6607156097194,1.37483737433787));
#81922=CARTESIAN_POINT('Ctrl Pts',(3.61887128440298,-18.7080115525041,1.32847064540805));
#81923=CARTESIAN_POINT('Ctrl Pts',(3.63389722882754,-18.7490626081558,1.27964638891813));
#81924=CARTESIAN_POINT('Ctrl Pts',(3.66225393957856,-18.7810702739468,1.23264761022329));
#81925=CARTESIAN_POINT('Ctrl Pts',(3.93117576959292,-18.4053110180947,1.49019805486829));
#81926=CARTESIAN_POINT('Ctrl Pts',(3.86848316971063,-18.4133452763836,1.50571006544666));
#81927=CARTESIAN_POINT('Ctrl Pts',(3.80576973439363,-18.43564302456,1.5110547043985));
#81928=CARTESIAN_POINT('Ctrl Pts',(3.74902367655503,-18.4714843750673,1.50465682308547));
#81929=CARTESIAN_POINT('Ctrl Pts',(3.65922142539151,-18.5627826491134,1.46970715178544));
#81930=CARTESIAN_POINT('Ctrl Pts',(3.62794609617334,-18.6740004978667,1.40065049328273));
#81931=CARTESIAN_POINT('Ctrl Pts',(3.62988278031609,-18.729777409853,1.36007776743956));
#81932=CARTESIAN_POINT('Ctrl Pts',(3.64919964740062,-18.7800152939447,1.31769811801765));
#81933=CARTESIAN_POINT('Ctrl Pts',(3.68264216713878,-18.8208888431934,1.27741247157079));
#81934=CARTESIAN_POINT('Ctrl Pts',(3.9423729901106,-18.4133858070116,1.50563516198861));
#81935=CARTESIAN_POINT('Ctrl Pts',(3.87743527118537,-18.4156185427818,1.51388218351694));
#81936=CARTESIAN_POINT('Ctrl Pts',(3.81247450205661,-18.4339621657064,1.51454292609738));
#81937=CARTESIAN_POINT('Ctrl Pts',(3.75386744558497,-18.4682828070917,1.50676736425539));
#81938=CARTESIAN_POINT('Ctrl Pts',(3.66185577629033,-18.5615214174088,1.47602002943265));
#81939=CARTESIAN_POINT('Ctrl Pts',(3.63177269714063,-18.6828496357294,1.4231722323832));
#81940=CARTESIAN_POINT('Ctrl Pts',(3.63526468072322,-18.7452967881311,1.39325441889084));
#81941=CARTESIAN_POINT('Ctrl Pts',(3.65692324111908,-18.8029219813393,1.36300667854291));
#81942=CARTESIAN_POINT('Ctrl Pts',(3.69312330991489,-18.8510565319363,1.33514740419474));
#81943=CARTESIAN_POINT('Ctrl Pts',(3.94235571266733,-18.4179625115314,1.5220642680868));
#81944=CARTESIAN_POINT('Ctrl Pts',(3.87742145776479,-18.4179007841395,1.52206437062455));
#81945=CARTESIAN_POINT('Ctrl Pts',(3.81246415607458,-18.4347501956728,1.51735346837426));
#81946=CARTESIAN_POINT('Ctrl Pts',(3.753859970967,-18.4686064148437,1.50790658895422));
#81947=CARTESIAN_POINT('Ctrl Pts',(3.66185171063921,-18.5630731192789,1.48156642851933));
#81948=CARTESIAN_POINT('Ctrl Pts',(3.63176679199362,-18.6893214659412,1.4463890385369));
#81949=CARTESIAN_POINT('Ctrl Pts',(3.63525637590299,-18.7550043776421,1.42809242464829));
#81950=CARTESIAN_POINT('Ctrl Pts',(3.65691132327402,-18.8162991820994,1.41102300383918));
#81951=CARTESIAN_POINT('Ctrl Pts',(3.69310713738719,-18.8681707290433,1.39658248257056));
#81952=CARTESIAN_POINT('Ctrl Pts',(3.94208066889,-18.4179535709002,1.52203266331995));
#81953=CARTESIAN_POINT('Ctrl Pts',(3.94208066889,-18.4159570093382,1.51487465397101));
#81954=CARTESIAN_POINT('Ctrl Pts',(3.93939976457242,-18.4131329107994,1.50784646200859));
#81955=CARTESIAN_POINT('Ctrl Pts',(3.93403795593725,-18.4094935804964,1.50114984350989));
#81956=CARTESIAN_POINT('Ctrl Pts',(3.92876493073444,-18.4059145119927,1.49456411087376));
#81957=CARTESIAN_POINT('Ctrl Pts',(3.9208990495868,-18.4015467557532,1.48829988745783));
#81958=CARTESIAN_POINT('Ctrl Pts',(3.91044031249432,-18.3964516676079,1.48255392252034));
#81959=CARTESIAN_POINT('Ctrl Pts',(3.90021604344847,-18.3914708031355,1.47693677286552));
#81960=CARTESIAN_POINT('Ctrl Pts',(3.88751387064069,-18.3857948927057,1.47181575064448));
#81961=CARTESIAN_POINT('Ctrl Pts',(3.87233379407099,-18.3795304027369,1.46736705768817));
#81962=CARTESIAN_POINT('Ctrl Pts',(3.86640409230692,-18.3770833427996,1.46562929158734));
#81963=CARTESIAN_POINT('Ctrl Pts',(3.86009629442993,-18.3745470069084,1.46399396287509));
#81964=CARTESIAN_POINT('Ctrl Pts',(3.85341040044,-18.3719297862815,1.46247080900171));
#81965=CARTESIAN_POINT('Origin',(2.225,-18.3216303794,1.54889979527));
#81966=CARTESIAN_POINT('Ctrl Pts',(3.94217663519884,-19.0766837901707,-1.2549536550141));
#81967=CARTESIAN_POINT('Ctrl Pts',(3.81239886354541,-19.076645554116,-1.25497330040668));
#81968=CARTESIAN_POINT('Ctrl Pts',(3.68259724249823,-19.1285376451827,-1.20779355502293));
#81969=CARTESIAN_POINT('Ctrl Pts',(3.60654250007182,-19.2341455692012,-1.1117978356177));
#81970=CARTESIAN_POINT('Ctrl Pts',(3.62070484051499,-19.3428207129455,-1.01302482729591));
#81971=CARTESIAN_POINT('Ctrl Pts',(3.69310717754101,-19.4225271378534,-0.94058821884175));
#81972=CARTESIAN_POINT('Ctrl Pts',(3.94218096368045,-19.0678969965114,-1.24528619924438));
#81973=CARTESIAN_POINT('Ctrl Pts',(3.8124013649262,-19.0766775490856,-1.25501070217547));
#81974=CARTESIAN_POINT('Ctrl Pts',(3.68259791616145,-19.1312291346839,-1.21075808335523));
#81975=CARTESIAN_POINT('Ctrl Pts',(3.60654273595517,-19.2294730875314,-1.10665936685993));
#81976=CARTESIAN_POINT('Ctrl Pts',(3.62070664165137,-19.324292537579,-0.992640516836252));
#81977=CARTESIAN_POINT('Ctrl Pts',(3.6931112295076,-19.3896240982595,-0.904387480917484));
#81978=CARTESIAN_POINT('Ctrl Pts',(3.93559125826023,-19.0576325988436,-1.23716461215919));
#81979=CARTESIAN_POINT('Ctrl Pts',(3.80845383863766,-19.0782981623898,-1.25360525685934));
#81980=CARTESIAN_POINT('Ctrl Pts',(3.68129345587565,-19.1367489342405,-1.21109305480358));
#81981=CARTESIAN_POINT('Ctrl Pts',(3.60588262725552,-19.2256736017137,-1.10083844359046));
#81982=CARTESIAN_POINT('Ctrl Pts',(3.61778298506652,-19.303259371832,-0.974962537597518));
#81983=CARTESIAN_POINT('Ctrl Pts',(3.68693955445337,-19.3511924443395,-0.873971611157963));
#81984=CARTESIAN_POINT('Ctrl Pts',(3.92284245621784,-19.0467376773103,-1.23131009492543));
#81985=CARTESIAN_POINT('Ctrl Pts',(3.80072347300955,-19.0792164390004,-1.24869960618928));
#81986=CARTESIAN_POINT('Ctrl Pts',(3.67858320514373,-19.1408681690318,-1.20498191179878));
#81987=CARTESIAN_POINT('Ctrl Pts',(3.60440977323658,-19.2195819167867,-1.09137485002728));
#81988=CARTESIAN_POINT('Ctrl Pts',(3.61202315176679,-19.2796909254035,-0.959797114573344));
#81989=CARTESIAN_POINT('Ctrl Pts',(3.67499936923216,-19.3103986831458,-0.852034828687459));
#81990=CARTESIAN_POINT('Ctrl Pts',(3.90640478505367,-19.0359499558752,-1.22729253742374));
#81991=CARTESIAN_POINT('Ctrl Pts',(3.78964230727276,-19.0775111308421,-1.24255371131931));
#81992=CARTESIAN_POINT('Ctrl Pts',(3.67286028089071,-19.1403088898408,-1.19643924561693));
#81993=CARTESIAN_POINT('Ctrl Pts',(3.60013259824114,-19.2091437100303,-1.08137464614068));
#81994=CARTESIAN_POINT('Ctrl Pts',(3.60330978482216,-19.2540235088518,-0.947806978160459));
#81995=CARTESIAN_POINT('Ctrl Pts',(3.65960361600605,-19.269997643815,-0.836974012631725));
#81996=CARTESIAN_POINT('Ctrl Pts',(3.8871831332344,-19.0254336179556,-1.22483553825469));
#81997=CARTESIAN_POINT('Ctrl Pts',(3.7758044692101,-19.0736895981168,-1.23616614954179));
#81998=CARTESIAN_POINT('Ctrl Pts',(3.66440795692671,-19.1360639649269,-1.18720250561116));
#81999=CARTESIAN_POINT('Ctrl Pts',(3.59323382499553,-19.195527288658,-1.07212003077549));
#82000=CARTESIAN_POINT('Ctrl Pts',(3.5920786079709,-19.2271843326888,-0.939102925829812));
#82001=CARTESIAN_POINT('Ctrl Pts',(3.64159969192542,-19.2306075924216,-0.827755843337992));
#82002=CARTESIAN_POINT('Ctrl Pts',(3.88711718104,-19.0254782582987,-1.22484599945563));
#82003=CARTESIAN_POINT('Ctrl Pts',(3.90102713913336,-19.0330874010163,-1.22662745096361));
#82004=CARTESIAN_POINT('Ctrl Pts',(3.91229688764402,-19.0404164069268,-1.22928808656999));
#82005=CARTESIAN_POINT('Ctrl Pts',(3.92092642657198,-19.0472854309651,-1.23271122429632));
#82006=CARTESIAN_POINT('Ctrl Pts',(3.92972882390163,-19.0542920485095,-1.23620293093707));
#82007=CARTESIAN_POINT('Ctrl Pts',(3.93578418014501,-19.0608195794311,-1.24048724663272));
#82008=CARTESIAN_POINT('Ctrl Pts',(3.93909249530211,-19.0667202939656,-1.24540700575729));
#82009=CARTESIAN_POINT('Ctrl Pts',(3.94108457006763,-19.0702733606974,-1.24836939825591));
#82010=CARTESIAN_POINT('Ctrl Pts',(3.94208063718359,-19.0736000363802,-1.25156159772694));
#82011=CARTESIAN_POINT('Ctrl Pts',(3.94208069665,-19.0766762824038,-1.25494542799359));
#82012=CARTESIAN_POINT('Origin',(2.225,-19.0026826744,-1.32221314666));
#82013=CARTESIAN_POINT('Origin',(-4.35,-1.95899712601,-5.55542016568));
#82014=CARTESIAN_POINT('',(-4.45,4.7773238354,-5.55542016568));
#82015=CARTESIAN_POINT('Origin',(-4.35,4.7773238354,-5.55542016568));
#82016=CARTESIAN_POINT('',(-4.45,-10.4080160928,-5.55542016568));
#82017=CARTESIAN_POINT('Origin',(-4.35,-10.4080160928,-5.55542016568));
#82018=CARTESIAN_POINT('',(-4.45,-2.8153461287,-5.55542016568));
#82019=CARTESIAN_POINT('Origin',(-4.35,-10.4080160928,-4.65542016568));
#82020=CARTESIAN_POINT('',(-4.45,-10.7858544195,-5.47226666221));
#82021=CARTESIAN_POINT('Origin',(-4.35,-10.7858544195,-5.47226666221));
#82022=CARTESIAN_POINT('Origin',(-4.45,-10.4080160928,-4.65542016568));
#82023=CARTESIAN_POINT('Origin',(-4.35,-15.667308925,-3.214314146));
#82024=CARTESIAN_POINT('',(-4.45,-18.9794133856,-1.68227598146));
#82025=CARTESIAN_POINT('Origin',(-4.35,-18.9794133856,-1.68227598146));
#82026=CARTESIAN_POINT('',(-4.45,-14.8826339026,-3.57727132183));
#82027=CARTESIAN_POINT('Origin',(-4.35,-18.895449313,-1.50075453779));
#82028=CARTESIAN_POINT('',(-4.45,-19.0409285996,-1.36351104187));
#82029=CARTESIAN_POINT('Origin',(-4.35,-19.0409285996,-1.36351104187));
#82030=CARTESIAN_POINT('Origin',(-4.45,-18.895449313,-1.50075453779));
#82031=CARTESIAN_POINT('Origin',(-4.35,-18.2859995693,2.04127093829));
#82032=CARTESIAN_POINT('',(-4.45,-18.4234397556,2.18656441774));
#82033=CARTESIAN_POINT('Origin',(-4.35,-18.4234397556,2.18656441774));
#82034=CARTESIAN_POINT('Origin',(-4.45,-18.2859995693,2.04127093829));
#82035=CARTESIAN_POINT('Origin',(-4.35,-18.85379408,1.77947127938));
#82036=CARTESIAN_POINT('',(-4.45,-14.4995104256,5.89840049188));
#82037=CARTESIAN_POINT('Origin',(-4.35,-14.4995104256,5.89840049188));
#82038=CARTESIAN_POINT('',(-4.45,-16.4614750906,4.04248245481));
#82039=CARTESIAN_POINT('Origin',(-4.35,-13.881029587,5.24457983432));
#82040=CARTESIAN_POINT('',(-4.45,-13.881029587,6.14457983432));
#82041=CARTESIAN_POINT('Origin',(-4.35,-13.881029587,6.14457983432));
#82042=CARTESIAN_POINT('Origin',(-4.45,-13.881029587,5.24457983432));
#82043=CARTESIAN_POINT('Origin',(-4.35,-1.95899712601,6.14457983432));
#82044=CARTESIAN_POINT('',(-4.45,-7.67105043563,6.14457983432));
#82045=CARTESIAN_POINT('Origin',(-4.35,-7.67105043563,6.14457983432));
#82046=CARTESIAN_POINT('',(-4.45,-10.7760400113,6.14457983432));
#82047=CARTESIAN_POINT('Origin',(-4.35,-7.67105043563,5.74457983432));
#82048=CARTESIAN_POINT('',(-4.45,-7.50411762961,6.1080814688));
#82049=CARTESIAN_POINT('Origin',(-4.35,-7.50411762961,6.1080814688));
#82050=CARTESIAN_POINT('Origin',(-4.45,-7.67105043563,5.74457983432));
#82051=CARTESIAN_POINT('Origin',(-4.35,4.59408048322,0.552161034916));
#82052=CARTESIAN_POINT('',(-4.45,-2.49116133917,3.80595465384));
#82053=CARTESIAN_POINT('Origin',(-4.35,-2.49116133917,3.80595465384));
#82054=CARTESIAN_POINT('',(-4.45,-4.99763948439,4.95701806132));
#82055=CARTESIAN_POINT('Origin',(-4.35,-2.24076213014,4.35120710557));
#82056=CARTESIAN_POINT('',(-4.45,-2.24076213014,3.75120710557));
#82057=CARTESIAN_POINT('Origin',(-4.35,-2.24076213014,3.75120710557));
#82058=CARTESIAN_POINT('Origin',(-4.45,-2.24076213014,4.35120710557));
#82059=CARTESIAN_POINT('Origin',(-4.35,-1.95899712601,3.75120710557));
#82060=CARTESIAN_POINT('',(-4.45,2.48275227055,3.75120710557));
#82061=CARTESIAN_POINT('Origin',(-4.35,2.48275227055,3.75120710557));
#82062=CARTESIAN_POINT('',(-4.45,0.120995070207,3.75120710557));
#82063=CARTESIAN_POINT('Origin',(-4.35,2.48275227055,4.35120710557));
#82064=CARTESIAN_POINT('',(-4.45,2.97160656206,4.00332568658));
#82065=CARTESIAN_POINT('Origin',(-4.35,2.97160656206,4.00332568658));
#82066=CARTESIAN_POINT('Origin',(-4.45,2.48275227055,4.35120710557));
#82067=CARTESIAN_POINT('Origin',(-4.35,0.332366624557,0.294579834316));
#82068=CARTESIAN_POINT('',(-4.45,4.32269078618,5.90191320834));
#82069=CARTESIAN_POINT('Origin',(-4.35,4.32269078618,5.90191320834));
#82070=CARTESIAN_POINT('',(-4.45,3.64714867412,4.95261944746));
#82071=CARTESIAN_POINT('Origin',(2.225,4.32269078618,5.90191320834));
#82072=CARTESIAN_POINT('Origin',(-4.35,4.32269078618,5.90191320834));
#82073=CARTESIAN_POINT('Origin',(-4.35,-1.95899712601,5.90191320834));
#82074=CARTESIAN_POINT('',(-4.45,4.7773238354,5.90191320834));
#82075=CARTESIAN_POINT('Origin',(-4.35,4.7773238354,5.90191320834));
#82076=CARTESIAN_POINT('',(-4.45,4.55000731079,5.90191320834));
#82077=CARTESIAN_POINT('Origin',(-4.35,4.32269078618,5.90191320834));
#82078=CARTESIAN_POINT('Origin',(2.225,4.7773238354,5.90191320834));
#82079=CARTESIAN_POINT('Origin',(-4.35,4.7773238354,5.90191320834));
#82080=CARTESIAN_POINT('Origin',(-4.35,4.7773238354,0.294579834316));
#82081=CARTESIAN_POINT('',(-4.45,4.7773238354,4.22878088412));
#82082=CARTESIAN_POINT('Origin',(-4.35,4.7773238354,4.22878088412));
#82083=CARTESIAN_POINT('',(-4.45,4.7773238354,5.06534704623));
#82084=CARTESIAN_POINT('Origin',(-4.35,4.7773238354,5.90191320834));
#82085=CARTESIAN_POINT('Origin',(-4.35,4.9773238354,4.22878088412));
#82086=CARTESIAN_POINT('',(-4.45,4.9773238354,4.02878088412));
#82087=CARTESIAN_POINT('Origin',(-4.35,4.9773238354,4.02878088412));
#82088=CARTESIAN_POINT('Origin',(-4.45,4.9773238354,4.22878088412));
#82089=CARTESIAN_POINT('Origin',(-4.35,-1.95899712601,4.02878088412));
#82090=CARTESIAN_POINT('',(-4.45,15.177455061,4.02878088412));
#82091=CARTESIAN_POINT('Origin',(-4.35,15.177455061,4.02878088412));
#82092=CARTESIAN_POINT('',(-4.45,10.0773894482,4.02878088412));
#82093=CARTESIAN_POINT('Origin',(2.225,15.177455061,4.02878088412));
#82094=CARTESIAN_POINT('Origin',(-4.35,15.177455061,4.02878088412));
#82095=CARTESIAN_POINT('Origin',(-4.35,15.177455061,0.294579834316));
#82096=CARTESIAN_POINT('',(-4.45,15.177455061,-4.67121911588));
#82097=CARTESIAN_POINT('Origin',(-4.35,15.177455061,-4.67121911588));
#82098=CARTESIAN_POINT('',(-4.45,15.177455061,-0.32121911588));
#82099=CARTESIAN_POINT('Origin',(-4.35,15.177455061,4.02878088412));
#82100=CARTESIAN_POINT('Origin',(2.225,15.177455061,-4.67121911588));
#82101=CARTESIAN_POINT('Origin',(-4.35,15.177455061,-4.67121911588));
#82102=CARTESIAN_POINT('Origin',(-4.35,-1.95899712601,-4.67121911588));
#82103=CARTESIAN_POINT('',(-4.45,4.9773238354,-4.67121911588));
#82104=CARTESIAN_POINT('Origin',(-4.35,4.9773238354,-4.67121911588));
#82105=CARTESIAN_POINT('',(-4.45,10.0773894482,-4.67121911588));
#82106=CARTESIAN_POINT('Origin',(-4.35,15.177455061,-4.67121911588));
#82107=CARTESIAN_POINT('Origin',(-4.35,4.9773238354,-4.87121911588));
#82108=CARTESIAN_POINT('',(-4.45,4.7773238354,-4.87121911588));
#82109=CARTESIAN_POINT('Origin',(-4.35,4.7773238354,-4.87121911588));
#82110=CARTESIAN_POINT('Origin',(-4.45,4.9773238354,-4.87121911588));
#82111=CARTESIAN_POINT('Origin',(-4.35,4.7773238354,0.294579834316));
#82112=CARTESIAN_POINT('',(-4.45,4.7773238354,-5.21331964078));
#82113=CARTESIAN_POINT('Origin',(4.35,0.,0.));
#82114=CARTESIAN_POINT('',(4.35,-10.5742356128,0.47366156039));
#82115=CARTESIAN_POINT('Origin',(4.35,-9.17423561284,0.47366156039));
#82116=CARTESIAN_POINT('Origin',(-4.35,-18.3216303794,1.54889979527));
#82117=CARTESIAN_POINT('Origin',(-4.35,-18.3216303794,1.54889979527));
#82118=CARTESIAN_POINT('Origin',(-7.44184532531,-9.17423561283998,0.473661560388455));
#82119=CARTESIAN_POINT('',(-5.0771333862,-11.8030366882,0.47366156039));
#82120=CARTESIAN_POINT('Origin',(-5.0771333862,-9.17423561284,0.47366156039));
#82121=CARTESIAN_POINT('',(-5.31156614753,-11.6198777414,0.47366156039));
#82122=CARTESIAN_POINT('',(-7.44184532530999,-9.95552123934695,0.473661560388455));
#82123=CARTESIAN_POINT('',(-5.31156614753,-6.74197323652571,0.218191104751761));
#82124=CARTESIAN_POINT('Origin',(-5.31156614753,-9.17423561284,0.473661560391));
#82125=CARTESIAN_POINT('Origin',(-5.31156614753,-9.17423561284,0.473661560391));
#82126=CARTESIAN_POINT('Origin',(4.4408920985E-16,-18.4073812884,1.48310265486));
#82127=CARTESIAN_POINT('',(-4.35,-17.9397782658,1.2109699402));
#82128=CARTESIAN_POINT('',(-4.35,-14.0218073513,-1.06918653748));
#82129=CARTESIAN_POINT('',(-3.225,-17.9397782658,1.2109699402));
#82130=CARTESIAN_POINT('Origin',(-2.3,-9.17423561284,0.47366156039));
#82131=CARTESIAN_POINT('',(-2.3,-11.82423561284,0.47366156039));
#82132=CARTESIAN_POINT('Origin',(-2.3,-9.17423561284,0.47366156039));
#82133=CARTESIAN_POINT('Origin',(-2.3,-12.12423561284,0.47366156039));
#82134=CARTESIAN_POINT('Origin',(-2.3,-12.0504559477,4.80274328646));
#82135=CARTESIAN_POINT('',(-2.3,-12.9053426461,5.10274328646));
#82136=CARTESIAN_POINT('Origin',(-2.3,-12.9053426461,4.80274328646));
#82137=CARTESIAN_POINT('',(-2.3,-9.41827086707,5.10274328646));
#82138=CARTESIAN_POINT('',(-2.3,-11.1618067566,5.10274328646));
#82139=CARTESIAN_POINT('Origin',(-2.3,-9.41827086707,4.80274328646));
#82140=CARTESIAN_POINT('Origin',(-2.3,-12.9053426461,4.10274328646));
#82141=CARTESIAN_POINT('',(-2.3,-13.5925435779,4.82921068375));
#82142=CARTESIAN_POINT('Origin',(-2.3,-13.3863832983,4.61127046457));
#82143=CARTESIAN_POINT('Origin',(-2.3,-12.9053426461,4.10274328646));
#82144=CARTESIAN_POINT('Origin',(-2.3,-10.0779006799,-3.15542016568));
#82145=CARTESIAN_POINT('',(-2.3,-10.0779006799,-4.15542016568));
#82146=CARTESIAN_POINT('Origin',(-2.3,-10.0779006799,-3.85542016568));
#82147=CARTESIAN_POINT('',(-2.3,-10.4977210429,-4.06302738404));
#82148=CARTESIAN_POINT('Origin',(-2.3,-10.0779006799,-3.15542016568));
#82149=CARTESIAN_POINT('Origin',(-2.3,-10.371774934,-3.79074521854));
#82150=CARTESIAN_POINT('Origin',(-2.3,-8.20939783898,-3.85542016568));
#82151=CARTESIAN_POINT('',(-2.3,-9.7480857735,-4.15542016568));
#82152=CARTESIAN_POINT('Origin',(-2.3,-8.67423561284,-4.1493785649));
#82153=CARTESIAN_POINT('',(-2.3,-8.7279990537,-3.65227747616));
#82154=CARTESIAN_POINT('Origin',(-2.3,-8.76025711822,-3.35401682291));
#82155=CARTESIAN_POINT('Origin',(-2.3,-8.67423561284,-4.1493785649));
#82156=CARTESIAN_POINT('Origin',(-2.3,-17.1183636721,1.08100826706));
#82157=CARTESIAN_POINT('',(-2.3,-17.3245239517,1.29894848625));
#82158=CARTESIAN_POINT('Origin',(-2.3,-17.1183636721,1.08100826706));
#82159=CARTESIAN_POINT('Origin',(-2.3,-17.1183636721,1.08100826706));
#82160=CARTESIAN_POINT('Origin',(-2.3,-16.3982789105,1.76217155265));
#82161=CARTESIAN_POINT('',(-2.3,-15.4585337648,3.064079585));
#82162=CARTESIAN_POINT('Origin',(-2.3,-17.3209666442,-0.597405571358));
#82163=CARTESIAN_POINT('',(-2.30000000000001,-17.3847397931138,-0.890548863178005));
#82164=CARTESIAN_POINT('Origin',(-2.3,-17.3209666442,-0.597405571358));
#82165=CARTESIAN_POINT('Ctrl Pts',(-2.15473685769753,-17.5697153662214,
-0.513604063130804));
#82166=CARTESIAN_POINT('Ctrl Pts',(-2.15395405942168,-17.574609993053,-0.529489742692386));
#82167=CARTESIAN_POINT('Ctrl Pts',(-2.15388324244328,-17.5783881601095,
-0.545799682384687));
#82168=CARTESIAN_POINT('Ctrl Pts',(-2.15451525157936,-17.5809692196611,
-0.562293625661652));
#82169=CARTESIAN_POINT('Ctrl Pts',(-2.1551503423395,-17.5835628642447,-0.578867992036593));
#82170=CARTESIAN_POINT('Ctrl Pts',(-2.1564949444798,-17.5849474880118,-0.595627317314118));
#82171=CARTESIAN_POINT('Ctrl Pts',(-2.15851501242277,-17.5850869864651,
-0.612320097566757));
#82172=CARTESIAN_POINT('Ctrl Pts',(-2.16056754790439,-17.5852287270071,
-0.629281172502292));
#82173=CARTESIAN_POINT('Ctrl Pts',(-2.16331716225515,-17.5840849489386,
-0.646172685370115));
#82174=CARTESIAN_POINT('Ctrl Pts',(-2.1667060874432,-17.5816670068449,-0.662735914936609));
#82175=CARTESIAN_POINT('Ctrl Pts',(-2.17014082128786,-17.5792163810321,
-0.679523032388902));
#82176=CARTESIAN_POINT('Ctrl Pts',(-2.17423187430862,-17.5754571498334,
-0.695972148081803));
#82177=CARTESIAN_POINT('Ctrl Pts',(-2.1789017592561,-17.5704498287427,-0.711831777793248));
#82178=CARTESIAN_POINT('Ctrl Pts',(-2.18365732878883,-17.5653506316774,
-0.727982405207925));
#82179=CARTESIAN_POINT('Ctrl Pts',(-2.18901271728734,-17.5589575689096,
-0.743521087226289));
#82180=CARTESIAN_POINT('Ctrl Pts',(-2.19487469522746,-17.5513795105412,
-0.758211607690351));
#82181=CARTESIAN_POINT('Ctrl Pts',(-2.20088007215961,-17.5436160734589,
-0.773261495905079));
#82182=CARTESIAN_POINT('Ctrl Pts',(-2.20741666432177,-17.5346095538899,
-0.787420812647958));
#82183=CARTESIAN_POINT('Ctrl Pts',(-2.21437945983172,-17.5245157190218,
-0.800474272147822));
#82184=CARTESIAN_POINT('Ctrl Pts',(-2.22171459988143,-17.5138821032147,
-0.814225782360628));
#82185=CARTESIAN_POINT('Ctrl Pts',(-2.22952228939455,-17.5020423686272,
-0.826749707962301));
#82186=CARTESIAN_POINT('Ctrl Pts',(-2.23768186400214,-17.4892117556151,
-0.837842740719717));
#82187=CARTESIAN_POINT('Ctrl Pts',(-2.24617531542753,-17.4758561343214,
-0.84938968273771));
#82188=CARTESIAN_POINT('Ctrl Pts',(-2.25504971643787,-17.4614274905277,
-0.859386461572597));
#82189=CARTESIAN_POINT('Ctrl Pts',(-2.26417755548704,-17.4461935944183,
-0.867655388024234));
#82190=CARTESIAN_POINT('Ctrl Pts',(-2.27393424211809,-17.4299101838862,
-0.876493988675408));
#82191=CARTESIAN_POINT('Ctrl Pts',(-2.28398040584175,-17.4127068136573,
-0.883358866726679));
#82192=CARTESIAN_POINT('Ctrl Pts',(-2.29417357219113,-17.3949324822234,
-0.888085993031839));
#82193=CARTESIAN_POINT('Ctrl Pts',(-2.29611068012178,-17.3915546507232,
-0.888984335464508));
#82194=CARTESIAN_POINT('Ctrl Pts',(-2.29805313306564,-17.3881562612702,
-0.88980560552101));
#82195=CARTESIAN_POINT('Ctrl Pts',(-2.3,-17.3847398009031,-0.890548854556042));
#82196=CARTESIAN_POINT('Origin',(-2.3,-17.4910283166,-1.37912101035));
#82197=CARTESIAN_POINT('',(-2.3,-17.2811181351,-0.925317401172));
#82198=CARTESIAN_POINT('Origin',(-2.3,-17.1551720262,-0.653035235664));
#82199=CARTESIAN_POINT('Origin',(-2.3,-17.4910283166,-1.37912101035));
#82200=CARTESIAN_POINT('Origin',(-2.3,-13.7337583338,-2.23563518556));
#82201=CARTESIAN_POINT('',(-2.3,-13.889419589,-2.49417239261));
#82202=CARTESIAN_POINT('Origin',(-2.3,-8.67423561284,5.09670168568));
#82203=CARTESIAN_POINT('',(-2.3,-9.13925764673,4.91297768617));
#82204=CARTESIAN_POINT('Origin',(-2.3,-9.41827086707,4.80274328646));
#82205=CARTESIAN_POINT('',(-2.3,-8.7279990537,4.59960059693));
#82206=CARTESIAN_POINT('Origin',(-2.3,-8.67423561284,5.09670168568));
#82207=CARTESIAN_POINT('Origin',(-2.3,-8.76025711822,4.30133994369));
#82208=CARTESIAN_POINT('Origin',(-2.3,-9.17423561284,0.47366156039));
#82209=CARTESIAN_POINT('Origin',(-2.3,-9.17423561284,0.47366156039));
#82210=CARTESIAN_POINT('Origin',(4.4408920985E-16,-17.4373752488,-0.853039529372));
#82211=CARTESIAN_POINT('',(-4.35,-17.6050062358,-0.892285274267));
#82212=CARTESIAN_POINT('',(-3.225,-17.6050062358,-0.892285274267));
#82213=CARTESIAN_POINT('',(-4.35,-1.98179270986,2.76541944482));
#82214=CARTESIAN_POINT('Origin',(-5.25,-9.17423561284,0.473661560391));
#82215=CARTESIAN_POINT('',(-5.35,-6.82034320266343,0.226422622515883));
#82216=CARTESIAN_POINT('Origin',(-5.25,-6.82034320266825,0.226422622516389));
#82217=CARTESIAN_POINT('',(-5.35,-6.8073945597,0.473677431302));
#82218=CARTESIAN_POINT('Origin',(-5.35,-9.17423561282425,0.473661560374535));
#82219=CARTESIAN_POINT('',(-5.35,-11.541076666,0.47366441431));
#82220=CARTESIAN_POINT('Origin',(-5.35,-9.17423561282426,0.47366156039));
#82221=CARTESIAN_POINT('Origin',(-5.35,-9.17423561282425,0.473661560374535));
#82222=CARTESIAN_POINT('Origin',(-4.35,4.32269078618,5.90191320834));
#82223=CARTESIAN_POINT('Origin',(-4.35,4.7773238354,5.90191320834));
#82224=CARTESIAN_POINT('Origin',(-4.35,15.177455061,4.02878088412));
#82225=CARTESIAN_POINT('Origin',(-4.35,15.177455061,-4.67121911588));
#82226=CARTESIAN_POINT('Origin',(0.,-9.17423561284,0.47366156039));
#82227=CARTESIAN_POINT('',(-5.35,-10.5742356128,0.47366156039));
#82228=CARTESIAN_POINT('Origin',(-5.35,-9.17423561284,0.47366156039));
#82229=CARTESIAN_POINT('',(0.,-10.57423561284,0.473661560390001));
#82230=CARTESIAN_POINT('Origin',(-4.35,-13.9715079445,-0.982757551184));
#82231=CARTESIAN_POINT('',(-4.45,-17.889478859,1.2973989265));
#82232=CARTESIAN_POINT('',(-4.45,-18.1055546192,1.42314936088));
#82233=CARTESIAN_POINT('Origin',(-4.35,-17.889478859,1.2973989265));
#82234=CARTESIAN_POINT('Origin',(-4.35,-17.6882812316,1.64311487169));
#82235=CARTESIAN_POINT('',(-4.35,-17.3446807657,1.27988117305));
#82236=CARTESIAN_POINT('Origin',(-4.35,-17.6882812316,1.64311487169));
#82237=CARTESIAN_POINT('',(-4.45,-17.4134008589,1.35252791278));
#82238=CARTESIAN_POINT('Origin',(-4.45,-17.6882812316,1.64311487169));
#82239=CARTESIAN_POINT('Origin',(-4.35,-17.4134008589,1.35252791278));
#82240=CARTESIAN_POINT('Origin',(-4.35,-17.907928075,0.88473050722));
#82241=CARTESIAN_POINT('',(-4.35,-13.5925435779,4.82921068375));
#82242=CARTESIAN_POINT('',(-4.35,-15.4686121718,3.0545459284));
#82243=CARTESIAN_POINT('',(-4.45,-13.661263671,4.90185742348));
#82244=CARTESIAN_POINT('',(-4.45,-15.537332265,3.12719266813));
#82245=CARTESIAN_POINT('Origin',(-4.35,-13.661263671,4.90185742348));
#82246=CARTESIAN_POINT('Origin',(-4.35,-12.9053426461,4.10274328646));
#82247=CARTESIAN_POINT('',(-4.35,-12.9053426461,5.10274328646));
#82248=CARTESIAN_POINT('Origin',(-4.35,-12.9053426461,4.10274328646));
#82249=CARTESIAN_POINT('',(-4.45,-12.9053426461,5.20274328646));
#82250=CARTESIAN_POINT('Origin',(-4.45,-12.9053426461,4.10274328646));
#82251=CARTESIAN_POINT('Origin',(-4.35,-12.9053426461,5.20274328646));
#82252=CARTESIAN_POINT('Origin',(-4.35,-1.95899712601,5.20274328646));
#82253=CARTESIAN_POINT('',(-4.35,-8.31430322211,5.10274328646));
#82254=CARTESIAN_POINT('',(-4.35,-10.6098229341,5.10274328646));
#82255=CARTESIAN_POINT('',(-4.45,-8.31430322211,5.20274328646));
#82256=CARTESIAN_POINT('',(-4.45,-10.6098229341,5.20274328646));
#82257=CARTESIAN_POINT('Origin',(-4.35,-8.31430322211,5.20274328646));
#82258=CARTESIAN_POINT('Origin',(-2.3,-9.41827086707,4.80274328646));
#82259=CARTESIAN_POINT('Origin',(-2.3,-9.41827086707,4.80274328646));
#82260=CARTESIAN_POINT('Origin',(3.225,-12.9053426461,4.10274328646));
#82261=CARTESIAN_POINT('',(-3.325,-12.9053426461,5.10274328646));
#82262=CARTESIAN_POINT('',(-3.325,-13.5925435779,4.82921068375));
#82263=CARTESIAN_POINT('Origin',(2.6645352591E-15,-19.4793690683,-1.15238185378));
#82264=CARTESIAN_POINT('',(-2.33871339239,-17.3446807657,1.27988117305));
#82265=CARTESIAN_POINT('Origin',(-2.33872773956445,-17.1384751807674,1.06192182456203));
#82266=CARTESIAN_POINT('Origin',(9.50350909079E-14,-19.6855293478,-0.934441634591));
#82267=CARTESIAN_POINT('Origin',(0.,-13.3033814002,5.10274328646));
#82268=CARTESIAN_POINT('',(-3.225,-17.3446807657,1.27988117305));
#82269=CARTESIAN_POINT('Origin',(-5.01556723867,-9.17423561284,0.47366156039));
#82270=CARTESIAN_POINT('',(-5.01556723867,-11.8242356128,0.47366156039));
#82271=CARTESIAN_POINT('Origin',(-5.01556723867,-11.72423561284,0.47366156039));
#82272=CARTESIAN_POINT('Origin',(-5.01556723867,-9.17423561284,0.47366156039));
#82273=CARTESIAN_POINT('Origin',(-5.35,0.,0.));
#82274=CARTESIAN_POINT('Origin',(-4.3,-2.12788809108,3.34387696505));
#82275=CARTESIAN_POINT('',(-4.,-2.69184369587,2.1725725316));
#82276=CARTESIAN_POINT('',(-4.3,-2.56170009476,2.4428735547));
#82277=CARTESIAN_POINT('Origin',(-4.3,-2.69184369587,2.1725725316));
#82278=CARTESIAN_POINT('',(-4.3,-2.12788809108,2.34387696505));
#82279=CARTESIAN_POINT('Origin',(-4.3,-2.12788809108,3.34387696505));
#82280=CARTESIAN_POINT('',(-4.,-2.12788809108,2.04387696505));
#82281=CARTESIAN_POINT('Origin',(-4.3,-2.12788809108,2.04387696505));
#82282=CARTESIAN_POINT('Origin',(-4.,-2.12788809108,3.34387696505));
#82283=CARTESIAN_POINT('Origin',(3.225,-9.41827086707,-3.85542016568));
#82284=CARTESIAN_POINT('',(-3.7,-9.13925764671,-3.96565456533));
#82285=CARTESIAN_POINT('',(3.,-9.13925764673,-3.96565456539));
#82286=CARTESIAN_POINT('',(-3.69999999774,-9.41827086749,-4.15542016568));
#82287=CARTESIAN_POINT('Origin',(-3.69999999887,-9.41827086707,-3.85542016568));
#82288=CARTESIAN_POINT('',(-3.,-9.41827086707,-4.15542016568));
#82289=CARTESIAN_POINT('Ctrl Pts',(-4.,2.8773238354,2.04387696505));
#82290=CARTESIAN_POINT('Ctrl Pts',(-4.,3.0773238354,2.04387696505));
#82291=CARTESIAN_POINT('Ctrl Pts',(-4.,3.0773238354,1.84387696505));
#82292=CARTESIAN_POINT('Ctrl Pts',(-4.,2.8773238354,2.34387696505));
#82293=CARTESIAN_POINT('Ctrl Pts',(-4.,3.3773238354,2.34387696505));
#82294=CARTESIAN_POINT('Ctrl Pts',(-4.,3.3773238354,1.84387696505));
#82295=CARTESIAN_POINT('Ctrl Pts',(-4.3,2.8773238354,2.34387696505));
#82296=CARTESIAN_POINT('Ctrl Pts',(-4.3,3.3773238354,2.34387696505));
#82297=CARTESIAN_POINT('Ctrl Pts',(-4.3,3.3773238354,1.84387696505));
#82298=CARTESIAN_POINT('',(-4.,2.8773238354,2.04387696505));
#82299=CARTESIAN_POINT('',(-4.3,2.8773238354,2.34387696505));
#82300=CARTESIAN_POINT('Origin',(-4.3,2.8773238354,2.04387696505));
#82301=CARTESIAN_POINT('',(-4.3,3.3773238354,1.84387696505));
#82302=CARTESIAN_POINT('Origin',(-4.3,2.8773238354,1.84387696505));
#82303=CARTESIAN_POINT('',(-4.,3.0773238354,1.84387696505));
#82304=CARTESIAN_POINT('Origin',(-4.3,3.0773238354,1.84387696505));
#82305=CARTESIAN_POINT('Origin',(-4.,2.8773238354,1.84387696505));
#82306=CARTESIAN_POINT('Origin',(-4.3,-2.74845588872,2.04387696505));
#82307=CARTESIAN_POINT('',(-4.3,0.374717872161,2.34387696505));
#82308=CARTESIAN_POINT('',(-4.,0.374717872161,2.04387696505));
#82309=CARTESIAN_POINT('Ctrl Pts',(-3.53153643377,-17.9397782186,1.21096972349));
#82310=CARTESIAN_POINT('Ctrl Pts',(-3.43735921762,-18.0003262942,1.24620711182));
#82311=CARTESIAN_POINT('Ctrl Pts',(-3.34318200148,-18.0897485133,1.23183031842));
#82312=CARTESIAN_POINT('Ctrl Pts',(-3.28035136998,-18.1886331834,1.15483650889));
#82313=CARTESIAN_POINT('Ctrl Pts',(-3.27308209541,-18.2588703936,1.04489890981));
#82314=CARTESIAN_POINT('Ctrl Pts',(-3.30849201868,-18.2908119879,0.937647001707));
#82315=CARTESIAN_POINT('Ctrl Pts',(-3.44407910476,-17.8762683682,1.17400854083));
#82316=CARTESIAN_POINT('Ctrl Pts',(-3.35980883034,-17.945884643,1.20261112942));
#82317=CARTESIAN_POINT('Ctrl Pts',(-3.27553855592,-18.0344942384,1.18180525286));
#82318=CARTESIAN_POINT('Ctrl Pts',(-3.21629253048,-18.1212598109,1.10210242162));
#82319=CARTESIAN_POINT('Ctrl Pts',(-3.20252794116,-18.1764816782,0.991308189139));
#82320=CARTESIAN_POINT('Ctrl Pts',(-3.22655830802,-18.1956140888,0.882244113432));
#82321=CARTESIAN_POINT('Ctrl Pts',(-3.3464798887,-17.8120594694,1.15225334483));
#82322=CARTESIAN_POINT('Ctrl Pts',(-3.27061651551,-17.8859816006,1.17073218793));
#82323=CARTESIAN_POINT('Ctrl Pts',(-3.19475314232,-17.9706270502,1.14263777494));
#82324=CARTESIAN_POINT('Ctrl Pts',(-3.13901290586,-18.0461110452,1.06262258853));
#82325=CARTESIAN_POINT('Ctrl Pts',(-3.12052271368,-18.0895777918,0.955511460449));
#82326=CARTESIAN_POINT('Ctrl Pts',(-3.1351232828,-18.0993679319,0.849634347569));
#82327=CARTESIAN_POINT('Ctrl Pts',(-3.24445759626,-17.7503923647,1.14165798595));
#82328=CARTESIAN_POINT('Ctrl Pts',(-3.17540943486,-17.8248792216,1.15059278692));
#82329=CARTESIAN_POINT('Ctrl Pts',(-3.10636127346,-17.9038800164,1.11677030553));
#82330=CARTESIAN_POINT('Ctrl Pts',(-3.05381470327,-17.9694500338,1.03769631264));
#82331=CARTESIAN_POINT('Ctrl Pts',(-3.03220663125,-18.0038208707,0.935228982262));
#82332=CARTESIAN_POINT('Ctrl Pts',(-3.03954447223,-18.006932574,0.833752309795));
#82333=CARTESIAN_POINT('Ctrl Pts',(-3.00710650148,-17.6178055192,1.13794464306));
#82334=CARTESIAN_POINT('Ctrl Pts',(-2.95127328323,-17.6885112346,1.12719077166));
#82335=CARTESIAN_POINT('Ctrl Pts',(-2.89544006498,-17.7531454598,1.08321253997));
#82336=CARTESIAN_POINT('Ctrl Pts',(-2.84959649515,-17.7987006574,1.00827828536));
#82337=CARTESIAN_POINT('Ctrl Pts',(-2.82308648415,-17.8163636325,0.917856141561));
#82338=CARTESIAN_POINT('Ctrl Pts',(-2.81718400147,-17.8081915572,0.828186375887));
#82339=CARTESIAN_POINT('Ctrl Pts',(-2.75866817858,-17.5019383088,1.17227759984));
#82340=CARTESIAN_POINT('Ctrl Pts',(-2.71204809217,-17.5606955711,1.14808808045));
#82341=CARTESIAN_POINT('Ctrl Pts',(-2.66542800575,-17.6093034777,1.10048544899));
#82342=CARTESIAN_POINT('Ctrl Pts',(-2.62523407894,-17.6396878429,1.03296291179));
#82343=CARTESIAN_POINT('Ctrl Pts',(-2.59761061232,-17.6474253317,0.955854949617));
#82344=CARTESIAN_POINT('Ctrl Pts',(-2.5844364843,-17.6345130992,0.879649456437));
#82345=CARTESIAN_POINT('Ctrl Pts',(-2.61902164686,-17.4433557891,1.20037711022));
#82346=CARTESIAN_POINT('Ctrl Pts',(-2.5768009727,-17.4944653366,1.17107895197));
#82347=CARTESIAN_POINT('Ctrl Pts',(-2.53458029853,-17.5345510327,1.12326065353));
#82348=CARTESIAN_POINT('Ctrl Pts',(-2.49727274202,-17.5577104896,1.06043707681));
#82349=CARTESIAN_POINT('Ctrl Pts',(-2.46964074457,-17.5611511175,0.990611628682));
#82350=CARTESIAN_POINT('Ctrl Pts',(-2.45360974016,-17.5467007921,0.921769238571));
#82351=CARTESIAN_POINT('Ctrl Pts',(-2.47860839712,-17.3907825954,1.23627120452));
#82352=CARTESIAN_POINT('Ctrl Pts',(-2.44020185655,-17.4338093447,1.20400270366));
#82353=CARTESIAN_POINT('Ctrl Pts',(-2.40179531599,-17.4659130997,1.15744985931));
#82354=CARTESIAN_POINT('Ctrl Pts',(-2.36716352241,-17.4829006471,1.09980337157));
#82355=CARTESIAN_POINT('Ctrl Pts',(-2.3399933307,-17.4830409793,1.03717095186));
#82356=CARTESIAN_POINT('Ctrl Pts',(-2.32206470888,-17.4678963173,0.975572621049));
#82357=CARTESIAN_POINT('Ctrl Pts',(-2.33871339239,-17.3446807657,1.27988117305));
#82358=CARTESIAN_POINT('Ctrl Pts',(-2.30368135741,-17.3797447841,1.24671240841));
#82359=CARTESIAN_POINT('Ctrl Pts',(-2.26864932242,-17.4046242104,1.20277710693));
#82360=CARTESIAN_POINT('Ctrl Pts',(-2.23651127409,-17.416397643,1.15078914283));
#82361=CARTESIAN_POINT('Ctrl Pts',(-2.21010973495,-17.414023754,1.09534670941));
#82362=CARTESIAN_POINT('Ctrl Pts',(-2.19100517814,-17.398792101,1.04094166862));
#82363=CARTESIAN_POINT('Ctrl Pts',(-2.33871339239,-17.3446807657,1.27988117305));
#82364=CARTESIAN_POINT('Ctrl Pts',(-2.37085722385345,-17.3552736346009,
1.26986086187324));
#82365=CARTESIAN_POINT('Ctrl Pts',(-2.40060138748257,-17.3654931419459,
1.26106505972869));
#82366=CARTESIAN_POINT('Ctrl Pts',(-2.42792441532416,-17.3751539348591,
1.25330473292905));
#82367=CARTESIAN_POINT('Ctrl Pts',(-2.45683268599488,-17.3853752331006,
1.24509416311528));
#82368=CARTESIAN_POINT('Ctrl Pts',(-2.48303144889736,-17.3949709404682,
1.23804288922432));
#82369=CARTESIAN_POINT('Ctrl Pts',(-2.50652519652193,-17.4037561126913,
1.23196427011995));
#82370=CARTESIAN_POINT('Ctrl Pts',(-2.52430430947977,-17.4104043738289,
1.22736421833548));
#82371=CARTESIAN_POINT('Ctrl Pts',(-2.54053497856681,-17.4165891620293,
1.22332190980238));
#82372=CARTESIAN_POINT('Ctrl Pts',(-2.55522602630707,-17.4222434165849,
1.2197694487075));
#82373=CARTESIAN_POINT('Ctrl Pts',(-2.57438046892142,-17.4296155316531,
1.21513768837394));
#82374=CARTESIAN_POINT('Ctrl Pts',(-2.59090554108931,-17.4360979659964,
1.21132852184931));
#82375=CARTESIAN_POINT('Ctrl Pts',(-2.6048009567519,-17.441601809986,1.20820745071824));
#82376=CARTESIAN_POINT('Ctrl Pts',(-2.60993120718498,-17.443633854129,1.20705513711276));
#82377=CARTESIAN_POINT('Ctrl Pts',(-2.61470302832676,-17.4455328588739,
1.20599698877206));
#82378=CARTESIAN_POINT('Ctrl Pts',(-2.61911644276473,-17.4472955559474,
1.2050275628334));
#82379=CARTESIAN_POINT('Ctrl Pts',(-2.62730007342115,-17.4505640597353,
1.20322999228066));
#82380=CARTESIAN_POINT('Ctrl Pts',(-2.63425131799992,-17.4533635882907,
1.20173688910744));
#82381=CARTESIAN_POINT('Ctrl Pts',(-2.63997017640731,-17.4556785810865,
1.20052048671079));
#82382=CARTESIAN_POINT('Ctrl Pts',(-2.642829605611,-17.4568360774844,1.19991228551246));
#82383=CARTESIAN_POINT('Ctrl Pts',(-2.64538093825375,-17.4578725207325,
1.19937341434368));
#82384=CARTESIAN_POINT('Ctrl Pts',(-2.64762417435145,-17.4587865567906,
1.1989012763582));
#82385=CARTESIAN_POINT('Ctrl Pts',(-2.6487457924003,-17.4592435748197,1.19866520736547));
#82386=CARTESIAN_POINT('Ctrl Pts',(-2.64979038631128,-17.4596699961906,
1.19844583132589));
#82387=CARTESIAN_POINT('Ctrl Pts',(-2.65075795608283,-17.4600656805176,
1.198242882505));
#82388=CARTESIAN_POINT('Ctrl Pts',(-2.65124174096861,-17.460263522681,1.19814140809456));
#82389=CARTESIAN_POINT('Ctrl Pts',(-2.65170626964839,-17.4604536819025,
1.19804404256586));
#82390=CARTESIAN_POINT('Ctrl Pts',(-2.65214192053663,-17.460632254491,1.19795273829656));
#82391=CARTESIAN_POINT('Ctrl Pts',(-2.65257757142488,-17.4608108270794,
1.19786143402726));
#82392=CARTESIAN_POINT('Ctrl Pts',(-2.65300365773986,-17.4609851971307,
1.19777165882951));
#82393=CARTESIAN_POINT('Ctrl Pts',(-2.65483063319514,-17.461736156073,1.19739003540087));
#82394=CARTESIAN_POINT('Ctrl Pts',(-2.68950642668481,-17.4759892743222,
1.19014686463782));
#82395=CARTESIAN_POINT('Ctrl Pts',(-2.72323913489447,-17.490340247288,1.18371785132662));
#82396=CARTESIAN_POINT('Ctrl Pts',(-2.75572764050077,-17.5045738471626,
1.17809425967101));
#82397=CARTESIAN_POINT('Ctrl Pts',(-2.77801459302075,-17.5143380255597,
1.17423650389304));
#82398=CARTESIAN_POINT('Ctrl Pts',(-2.79971637818909,-17.5240463924571,
1.17075696072237));
#82399=CARTESIAN_POINT('Ctrl Pts',(-2.8207410235801,-17.5336236381446,1.16764089921239));
#82400=CARTESIAN_POINT('Ctrl Pts',(-2.84657754344982,-17.5453928116027,
1.16381167005678));
#82401=CARTESIAN_POINT('Ctrl Pts',(-2.87138972981263,-17.556965111084,1.16052926742677));
#82402=CARTESIAN_POINT('Ctrl Pts',(-2.89517608835571,-17.5682913708109,
1.15772838507829));
#82403=CARTESIAN_POINT('Ctrl Pts',(-2.90706926762725,-17.5739545006744,
1.15632794390404));
#82404=CARTESIAN_POINT('Ctrl Pts',(-2.91870376450622,-17.5795588671794,
1.15504729109772));
#82405=CARTESIAN_POINT('Ctrl Pts',(-2.93008295529788,-17.585095124209,1.15387927549878));
#82406=CARTESIAN_POINT('Ctrl Pts',(-2.93577255069372,-17.5878632527238,
1.15329526769931));
#82407=CARTESIAN_POINT('Ctrl Pts',(-2.94139832389838,-17.5906143505413,
1.15273941070078));
#82408=CARTESIAN_POINT('Ctrl Pts',(-2.94696039348753,-17.5933476575522,
1.15221069698343));
#82409=CARTESIAN_POINT('Ctrl Pts',(-2.94974142828211,-17.5947143110577,
1.15194634012475));
#82410=CARTESIAN_POINT('Ctrl Pts',(-2.95250653708668,-17.5960765170342,
1.15168876905108));
#82411=CARTESIAN_POINT('Ctrl Pts',(-2.95525573651771,-17.5974341826461,
1.15143785739361));
#82412=CARTESIAN_POINT('Ctrl Pts',(-2.95780061870979,-17.598690948161,1.15120559319273));
#82413=CARTESIAN_POINT('Ctrl Pts',(-2.95930210470662,-17.5994332235654,
1.15106977482125));
#82414=CARTESIAN_POINT('Ctrl Pts',(-2.9626199252829,-17.6010788586254,1.15077824350422));
#82415=CARTESIAN_POINT('Ctrl Pts',(-2.96288629829677,-17.6012109793234,
1.15075483775524));
#82416=CARTESIAN_POINT('Ctrl Pts',(-2.96316437249295,-17.6013489348644,
1.15073045290619));
#82417=CARTESIAN_POINT('Ctrl Pts',(-2.96345562364545,-17.601493466588,1.15070497409997));
#82418=CARTESIAN_POINT('Ctrl Pts',(-2.98660845975514,-17.6129829294787,
1.1486795516434));
#82419=CARTESIAN_POINT('Ctrl Pts',(-3.00924236604217,-17.6244510594205,
1.14707287507716));
#82420=CARTESIAN_POINT('Ctrl Pts',(-3.03135622106119,-17.6358748807149,
1.14586888188318));
#82421=CARTESIAN_POINT('Ctrl Pts',(-3.07548657744149,-17.658672231268,1.14346619593431));
#82422=CARTESIAN_POINT('Ctrl Pts',(-3.11754201398305,-17.6812897018117,
1.14266734811753));
#82423=CARTESIAN_POINT('Ctrl Pts',(-3.15750338943099,-17.703545586087,1.14334632593646));
#82424=CARTESIAN_POINT('Ctrl Pts',(-3.20904005267743,-17.7322481520094,
1.1442219777581));
#82425=CARTESIAN_POINT('Ctrl Pts',(-3.25709852006457,-17.7603520183409,
1.14755784233417));
#82426=CARTESIAN_POINT('Ctrl Pts',(-3.30167585169498,-17.7875179004328,
1.15305956494331));
#82427=CARTESIAN_POINT('Ctrl Pts',(-3.34214685945926,-17.8121813467373,
1.15805448613505));
#82428=CARTESIAN_POINT('Ctrl Pts',(-3.37974752021567,-17.836071417311,1.16483514835252));
#82429=CARTESIAN_POINT('Ctrl Pts',(-3.41447735425161,-17.8589510516284,
1.17314411559556));
#82430=CARTESIAN_POINT('Ctrl Pts',(-3.44443398255037,-17.8786861502802,
1.18031111337011));
#82431=CARTESIAN_POINT('Ctrl Pts',(-3.47225349205163,-17.8976688837122,
1.18861468802206));
#82432=CARTESIAN_POINT('Ctrl Pts',(-3.49795473249979,-17.9157683536315,
1.19786218814635));
#82433=CARTESIAN_POINT('Ctrl Pts',(-3.5095802536272,-17.9239553425189,1.20204513831513));
#82434=CARTESIAN_POINT('Ctrl Pts',(-3.5207727482244,-17.9319619744418,1.20642085871186));
#82435=CARTESIAN_POINT('Ctrl Pts',(-3.53153633920471,-17.9397782793976,
1.21096975887257));
#82436=CARTESIAN_POINT('Origin',(-3.225,-17.6882812316,1.64311487169));
#82437=CARTESIAN_POINT('Origin',(0.,-9.17423561284,0.47366156039));
#82438=CARTESIAN_POINT('',(0.,-11.82423561284,0.47366156039));
#82439=CARTESIAN_POINT('Origin',(-4.3,3.0773238354,0.47366156039));
#82440=CARTESIAN_POINT('',(-4.3,3.3773238354,-3.65542016568));
#82441=CARTESIAN_POINT('',(-4.3,3.3773238354,-0.905771600316));
#82442=CARTESIAN_POINT('',(-4.,3.0773238354,-3.65542016568));
#82443=CARTESIAN_POINT('Origin',(-4.3,3.0773238354,-3.65542016568));
#82444=CARTESIAN_POINT('',(-4.,3.0773238354,-0.905771600316));
#82445=CARTESIAN_POINT('Origin',(-4.35,-10.0779006799,-3.15542016568));
#82446=CARTESIAN_POINT('',(-4.35,-10.4977210429,-4.06302738404));
#82447=CARTESIAN_POINT('',(-4.35,-10.0779006799,-4.15542016568));
#82448=CARTESIAN_POINT('Origin',(-4.35,-10.0779006799,-3.15542016568));
#82449=CARTESIAN_POINT('',(-4.45,-10.0779006799,-4.25542016568));
#82450=CARTESIAN_POINT('Origin',(-4.35,-10.0779006799,-4.25542016568));
#82451=CARTESIAN_POINT('',(-4.45,-10.5397030792,-4.15378810588));
#82452=CARTESIAN_POINT('Origin',(-4.45,-10.0779006799,-3.15542016568));
#82453=CARTESIAN_POINT('Origin',(-4.35,-10.5397030792,-4.15378810588));
#82454=CARTESIAN_POINT('Origin',(-4.35,-14.1190276664,-2.49814531564));
#82455=CARTESIAN_POINT('',(-4.35,-17.2811181351,-0.925317401172));
#82456=CARTESIAN_POINT('',(-4.35,-13.889419589,-2.49417239261));
#82457=CARTESIAN_POINT('',(-4.45,-17.3231001714,-1.01607812301));
#82458=CARTESIAN_POINT('',(-4.45,-13.9314016253,-2.58493311444));
#82459=CARTESIAN_POINT('Origin',(-4.35,-17.3231001714,-1.01607812301));
#82460=CARTESIAN_POINT('Origin',(-4.45,0.,0.));
#82461=CARTESIAN_POINT('',(-4.45,-19.0026826744,-1.32221314666));
#82462=CARTESIAN_POINT('Origin',(-4.45,-21.2594877202,0.729452270839));
#82463=CARTESIAN_POINT('',(-4.45,-17.582210652,-0.989652421484));
#82464=CARTESIAN_POINT('',(-4.45,-1.95899712601,2.6680522976));
#82465=CARTESIAN_POINT('Origin',(-4.45,-17.4910283166,-1.37912101035));
#82466=CARTESIAN_POINT('',(-4.45,2.8773238354,-4.25542016568));
#82467=CARTESIAN_POINT('',(-4.45,-1.95899712601,-4.25542016568));
#82468=CARTESIAN_POINT('',(-4.45,3.4773238354,-3.65542016568));
#82469=CARTESIAN_POINT('Origin',(-4.45,2.8773238354,-3.65542016568));
#82470=CARTESIAN_POINT('',(-4.45,3.4773238354,1.84387696505));
#82471=CARTESIAN_POINT('',(-4.45,3.4773238354,0.294579834316));
#82472=CARTESIAN_POINT('',(-4.45,2.8773238354,2.44387696505));
#82473=CARTESIAN_POINT('Origin',(-4.45,2.8773238354,1.84387696505));
#82474=CARTESIAN_POINT('',(-4.45,-2.12788809108,2.44387696505));
#82475=CARTESIAN_POINT('',(-4.45,-1.95899712601,2.44387696505));
#82476=CARTESIAN_POINT('',(-4.45,-2.51831889439,2.53297389574));
#82477=CARTESIAN_POINT('Origin',(-4.45,-2.12788809108,3.34387696505));
#82478=CARTESIAN_POINT('',(-4.45,-7.83711001806,5.09384703785));
#82479=CARTESIAN_POINT('',(-4.45,2.13070110951,0.294579834316));
#82480=CARTESIAN_POINT('Origin',(-4.45,-8.31430322211,4.10274328646));
#82481=CARTESIAN_POINT('Origin',(-4.35,-21.2594877202,0.729452270839));
#82482=CARTESIAN_POINT('Origin',(-4.35,-19.0026826744,-1.32221314666));
#82483=CARTESIAN_POINT('Origin',(-4.35,-19.0026826744,-1.32221314666));
#82484=CARTESIAN_POINT('Origin',(-4.35,-19.0026826744,-1.32221314666));
#82485=CARTESIAN_POINT('Origin',(-4.35,-1.95899712601,2.6680522976));
#82486=CARTESIAN_POINT('Origin',(-4.35,-17.582210652,-0.989652421484));
#82487=CARTESIAN_POINT('Origin',(-4.35,-17.4910283166,-1.37912101035));
#82488=CARTESIAN_POINT('Origin',(-4.35,-17.4910283166,-1.37912101035));
#82489=CARTESIAN_POINT('Ctrl Pts',(-2.30026150234977,-17.3820580265551,
-0.891121645497691));
#82490=CARTESIAN_POINT('Ctrl Pts',(-2.2511020282712,-17.4685660559916,-0.873172032485047));
#82491=CARTESIAN_POINT('Ctrl Pts',(-2.2017503487722,-17.5463291774412,-0.813547788890955));
#82492=CARTESIAN_POINT('Ctrl Pts',(-2.16413757728291,-17.5942001577229,
-0.71591120019767));
#82493=CARTESIAN_POINT('Ctrl Pts',(-2.14871234024909,-17.5988806949977,
-0.607385187645706));
#82494=CARTESIAN_POINT('Ctrl Pts',(-2.15387724303736,-17.5683659671124,
-0.511132105859265));
#82495=CARTESIAN_POINT('Ctrl Pts',(-2.40878057050813,-17.418797425994,-0.882916394445839));
#82496=CARTESIAN_POINT('Ctrl Pts',(-2.35504797194602,-17.5086551346987,
-0.87112727920342));
#82497=CARTESIAN_POINT('Ctrl Pts',(-2.30108940419278,-17.5922280790055,
-0.813709700010545));
#82498=CARTESIAN_POINT('Ctrl Pts',(-2.26093305392475,-17.6458395466711,
-0.713034714408869));
#82499=CARTESIAN_POINT('Ctrl Pts',(-2.24664268994449,-17.6534402243889,
-0.599427746817492));
#82500=CARTESIAN_POINT('Ctrl Pts',(-2.25552652731881,-17.6235908872705,
-0.498965911082793));
#82501=CARTESIAN_POINT('Ctrl Pts',(-2.51566402719547,-17.4589771799051,
-0.877572242965746));
#82502=CARTESIAN_POINT('Ctrl Pts',(-2.45670878457325,-17.5514899225794,
-0.872981025895007));
#82503=CARTESIAN_POINT('Ctrl Pts',(-2.39748577966448,-17.6410198701621,
-0.818594729897352));
#82504=CARTESIAN_POINT('Ctrl Pts',(-2.35461942392657,-17.7011884981179,
-0.714934954500043));
#82505=CARTESIAN_POINT('Ctrl Pts',(-2.34208969093556,-17.7124931079571,
-0.595961003183311));
#82506=CARTESIAN_POINT('Ctrl Pts',(-2.35565283813046,-17.683962733608,-0.491125495637028));
#82507=CARTESIAN_POINT('Ctrl Pts',(-2.62041115594089,-17.5028395885339,
-0.87613658390424));
#82508=CARTESIAN_POINT('Ctrl Pts',(-2.5553750193492,-17.5968327517438,-0.879749872744001));
#82509=CARTESIAN_POINT('Ctrl Pts',(-2.49001831660964,-17.69222510147,-0.82932513722258));
#82510=CARTESIAN_POINT('Ctrl Pts',(-2.44424641281096,-17.7599256351865,
-0.722853057106192));
#82511=CARTESIAN_POINT('Ctrl Pts',(-2.43432528251228,-17.7760500789645,
-0.598373539580247));
#82512=CARTESIAN_POINT('Ctrl Pts',(-2.4537889856892,-17.7498341449337,-0.489185387248891));
#82513=CARTESIAN_POINT('Ctrl Pts',(-2.7224545911624,-17.5507108773925,-0.879827372138517));
#82514=CARTESIAN_POINT('Ctrl Pts',(-2.65009743783106,-17.6443621840397,
-0.892953323240521));
#82515=CARTESIAN_POINT('Ctrl Pts',(-2.57735067987483,-17.7452621208078,
-0.84787026250574));
#82516=CARTESIAN_POINT('Ctrl Pts',(-2.5284103961115,-17.821745215291,-0.738849741797549));
#82517=CARTESIAN_POINT('Ctrl Pts',(-2.52234106163441,-17.8441995989119,
-0.608578431302329));
#82518=CARTESIAN_POINT('Ctrl Pts',(-2.54940634153372,-17.8216799279534,
-0.494979618252563));
#82519=CARTESIAN_POINT('Ctrl Pts',(-2.81901489023132,-17.6025946693237,
-0.891701921170512));
#82520=CARTESIAN_POINT('Ctrl Pts',(-2.73744075495876,-17.6921936758885,
-0.914074996544492));
#82521=CARTESIAN_POINT('Ctrl Pts',(-2.65538058640039,-17.7967415471119,
-0.875010275347337));
#82522=CARTESIAN_POINT('Ctrl Pts',(-2.60302630158974,-17.8835187867793,
-0.764336819213081));
#82523=CARTESIAN_POINT('Ctrl Pts',(-2.60282559743216,-17.9153183318905,
-0.629507557784543));
#82524=CARTESIAN_POINT('Ctrl Pts',(-2.63990390140954,-17.8994711764097,
-0.513073271338585));
#82525=CARTESIAN_POINT('Ctrl Pts',(-2.81682310404,-17.6050062358,-0.892285274267));
#82526=CARTESIAN_POINT('Ctrl Pts',(-2.77238544150798,-17.5811167968899,
-0.886692281931633));
#82527=CARTESIAN_POINT('Ctrl Pts',(-2.7243400982194,-17.5570466401642,-0.882915995356844));
#82528=CARTESIAN_POINT('Ctrl Pts',(-2.67274747304574,-17.5330452228065,
-0.880894863642099));
#82529=CARTESIAN_POINT('Ctrl Pts',(-2.62668804079532,-17.5116179034371,
-0.87909049375452));
#82530=CARTESIAN_POINT('Ctrl Pts',(-2.57780359900481,-17.4902459976349,
-0.878683248104142));
#82531=CARTESIAN_POINT('Ctrl Pts',(-2.52610297724738,-17.4691042792122,
-0.879609375083118));
#82532=CARTESIAN_POINT('Ctrl Pts',(-2.47295527054473,-17.4473708104119,
-0.880561424079336));
#82533=CARTESIAN_POINT('Ctrl Pts',(-2.41683107761332,-17.4258804100421,
-0.882923772785761));
#82534=CARTESIAN_POINT('Ctrl Pts',(-2.35768503181644,-17.4048159349658,
-0.886610023581458));
#82535=CARTESIAN_POINT('Ctrl Pts',(-2.33876680496398,-17.3980783329393,
-0.887789093591101));
#82536=CARTESIAN_POINT('Ctrl Pts',(-2.319539086922,-17.3913842780576,-0.889103366281777));
#82537=CARTESIAN_POINT('Ctrl Pts',(-2.30000000000002,-17.3847398066618,
-0.890548881027004));
#82538=CARTESIAN_POINT('Origin',(-3.225,-17.4910283166,-1.37912101035));
#82539=CARTESIAN_POINT('',(-3.325,-17.2811181351,-0.925317401172));
#82540=CARTESIAN_POINT('Origin',(0.,-10.2979776218,-4.15542016568));
#82541=CARTESIAN_POINT('',(3.225,-10.4977210429,-4.06302738404));
#82542=CARTESIAN_POINT('Origin',(3.225,-10.0779006799,-3.15542016568));
#82543=CARTESIAN_POINT('',(-3.325,-10.0779006799,-4.15542016568));
#82544=CARTESIAN_POINT('Origin',(0.,3.3773238354,-4.15542016568));
#82545=CARTESIAN_POINT('',(-4.35,2.8773238354,-4.15542016568));
#82546=CARTESIAN_POINT('',(-4.35,-1.95899712601,-4.15542016568));
#82547=CARTESIAN_POINT('',(-4.29232316258844,-8.70602835244453,-4.15542016568));
#82548=CARTESIAN_POINT('Ctrl Pts',(-4.29232316225885,-8.70602837142191,
-4.15542016568));
#82549=CARTESIAN_POINT('Ctrl Pts',(-4.29205120071452,-8.72168753702626,
-4.15542016568));
#82550=CARTESIAN_POINT('Ctrl Pts',(-4.29158720532918,-8.73740648674787,
-4.15542016568278));
#82551=CARTESIAN_POINT('Ctrl Pts',(-4.29086254081513,-8.75324772180714,
-4.15542016514087));
#82552=CARTESIAN_POINT('Ctrl Pts',(-4.29008645301039,-8.77021307488149,
-4.15542016456051));
#82553=CARTESIAN_POINT('Ctrl Pts',(-4.28901119399487,-8.7873184421748,-4.15542016334628));
#82554=CARTESIAN_POINT('Ctrl Pts',(-4.28754966268177,-8.80457940448153,
-4.15542016341833));
#82555=CARTESIAN_POINT('Ctrl Pts',(-4.28677487233489,-8.81372982558667,
-4.15542016345652));
#82556=CARTESIAN_POINT('Ctrl Pts',(-4.28589150051295,-8.8229229964194,-4.15542016392521));
#82557=CARTESIAN_POINT('Ctrl Pts',(-4.28488660862881,-8.83215545542406,
-4.15542016457497));
#82558=CARTESIAN_POINT('Ctrl Pts',(-4.28275134959082,-8.85177317932411,
-4.15542016595563));
#82559=CARTESIAN_POINT('Ctrl Pts',(-4.28003832504559,-8.87155237324264,
-4.15542016566606));
#82560=CARTESIAN_POINT('Ctrl Pts',(-4.27662963897357,-8.89139030340002,
-4.15542016567672));
#82561=CARTESIAN_POINT('Ctrl Pts',(-4.27453046995187,-8.90360708357898,
-4.15542016568329));
#82562=CARTESIAN_POINT('Ctrl Pts',(-4.27216774709283,-8.91584486940965,
-4.15542016568));
#82563=CARTESIAN_POINT('Ctrl Pts',(-4.26951780859382,-8.92807096217797,
-4.15542016568));
#82564=CARTESIAN_POINT('Ctrl Pts',(-4.26468368982784,-8.95037426638974,
-4.15542016568));
#82565=CARTESIAN_POINT('Ctrl Pts',(-4.25889294909336,-8.97263030125832,
-4.15542016568));
#82566=CARTESIAN_POINT('Ctrl Pts',(-4.25202546552033,-8.99462871319934,
-4.15542016568));
#82567=CARTESIAN_POINT('Ctrl Pts',(-4.24866331428397,-9.00539859522655,
-4.15542016568));
#82568=CARTESIAN_POINT('Ctrl Pts',(-4.24504378092221,-9.01610634900063,
-4.15542016568));
#82569=CARTESIAN_POINT('Ctrl Pts',(-4.24115737109246,-9.02672676812152,
-4.15542016568));
#82570=CARTESIAN_POINT('Ctrl Pts',(-4.23426685680616,-9.04555652434511,
-4.15542016568));
#82571=CARTESIAN_POINT('Ctrl Pts',(-4.22653159494977,-9.06411864425602,
-4.15542016568));
#82572=CARTESIAN_POINT('Ctrl Pts',(-4.21793147778923,-9.08227287068491,
-4.15542016568));
#82573=CARTESIAN_POINT('Ctrl Pts',(-4.2100789353958,-9.0988490207526,-4.15542016568));
#82574=CARTESIAN_POINT('Ctrl Pts',(-4.2015054941613,-9.11508438284678,-4.15542016568));
#82575=CARTESIAN_POINT('Ctrl Pts',(-4.1922309596074,-9.13089839049763,-4.15542016568));
#82576=CARTESIAN_POINT('Ctrl Pts',(-4.18815592541805,-9.13784673075918,
-4.15542016568));
#82577=CARTESIAN_POINT('Ctrl Pts',(-4.1839460127474,-9.14471414658231,-4.15542016568));
#82578=CARTESIAN_POINT('Ctrl Pts',(-4.17960523291625,-9.1514961102524,-4.15542016568));
#82579=CARTESIAN_POINT('Ctrl Pts',(-4.16634611145727,-9.17221194554702,
-4.15542016568));
#82580=CARTESIAN_POINT('Ctrl Pts',(-4.15184518108592,-9.19211860151861,
-4.15542016617984));
#82581=CARTESIAN_POINT('Ctrl Pts',(-4.13618163257724,-9.21102766582222,
-4.15542016179659));
#82582=CARTESIAN_POINT('Ctrl Pts',(-4.11973553103685,-9.23088142957176,
-4.15542015719435));
#82583=CARTESIAN_POINT('Ctrl Pts',(-4.10200809428551,-9.24963529413492,
-4.15542014577611));
#82584=CARTESIAN_POINT('Ctrl Pts',(-4.08313350202983,-9.26711150454399,
-4.15542013374396));
#82585=CARTESIAN_POINT('Ctrl Pts',(-4.07176321009623,-9.27763939365293,
-4.15542012649563));
#82586=CARTESIAN_POINT('Ctrl Pts',(-4.05997740445791,-9.28770440729055,
-4.15542011955517));
#82587=CARTESIAN_POINT('Ctrl Pts',(-4.04781138042469,-9.29727441845877,
-4.15542011643421));
#82588=CARTESIAN_POINT('Ctrl Pts',(-4.02659799740219,-9.31396124333162,
-4.15542011099231));
#82589=CARTESIAN_POINT('Ctrl Pts',(-4.00423092936188,-9.32913206089668,
-4.15542011535558));
#82590=CARTESIAN_POINT('Ctrl Pts',(-3.98091614962384,-9.34262747027809,
-4.15542012343284));
#82591=CARTESIAN_POINT('Ctrl Pts',(-3.95650110095926,-9.3567597537694,-4.15542013189127));
#82592=CARTESIAN_POINT('Ctrl Pts',(-3.93104736555546,-9.36905451674416,
-4.15542014341187));
#82593=CARTESIAN_POINT('Ctrl Pts',(-3.90483049009711,-9.37937035892166,
-4.15542015118524));
#82594=CARTESIAN_POINT('Ctrl Pts',(-3.89672696602562,-9.38255894161665,
-4.15542015358796));
#82595=CARTESIAN_POINT('Ctrl Pts',(-3.88855076480426,-9.38555876112294,
-4.15542015568561));
#82596=CARTESIAN_POINT('Ctrl Pts',(-3.88031058139973,-9.38836645220462,
-4.1554201574361));
#82597=CARTESIAN_POINT('Ctrl Pts',(-3.85132370712238,-9.39824319698063,
-4.15542016359385));
#82598=CARTESIAN_POINT('Ctrl Pts',(-3.82154088715569,-9.40573335220575,
-4.15542016471136));
#82599=CARTESIAN_POINT('Ctrl Pts',(-3.79135695696281,-9.41074020445555,
-4.15542016528016));
#82600=CARTESIAN_POINT('Ctrl Pts',(-3.76117302676992,-9.41574705670534,
-4.15542016584896));
#82601=CARTESIAN_POINT('Ctrl Pts',(-3.73058948857333,-9.41827087355667,
-4.15542016568));
#82602=CARTESIAN_POINT('Ctrl Pts',(-3.69999999774,-9.41827086749,-4.15542016568));
#82603=CARTESIAN_POINT('',(-4.3,-8.14391944342,-4.15542016568));
#82604=CARTESIAN_POINT('Ctrl Pts',(-4.3,-8.14391944342,-4.15542016568));
#82605=CARTESIAN_POINT('Ctrl Pts',(-4.3,-8.20648904053108,-4.15542016568));
#82606=CARTESIAN_POINT('Ctrl Pts',(-4.29947971883186,-8.26880371250586,
-4.15542016568));
#82607=CARTESIAN_POINT('Ctrl Pts',(-4.29869536600186,-8.33090046659907,
-4.15542016568));
#82608=CARTESIAN_POINT('Ctrl Pts',(-4.29790074267177,-8.39381033016885,
-4.15542016568));
#82609=CARTESIAN_POINT('Ctrl Pts',(-4.29683500095811,-8.45649622088276,
-4.15542016568));
#82610=CARTESIAN_POINT('Ctrl Pts',(-4.29571075913684,-8.51899937638185,
-4.15542016568));
#82611=CARTESIAN_POINT('Ctrl Pts',(-4.29458651731557,-8.58150253188095,
-4.15542016568));
#82612=CARTESIAN_POINT('Ctrl Pts',(-4.2934034804918,-8.64382608258768,-4.15542016568));
#82613=CARTESIAN_POINT('Ctrl Pts',(-4.29232316291,-8.70602833393,-4.15542016568));
#82614=CARTESIAN_POINT('',(-4.3,2.8773238354,-4.15542016568));
#82615=CARTESIAN_POINT('',(-4.3,-3.42065492897,-4.15542016568));
#82616=CARTESIAN_POINT('',(3.225,2.8773238354,-4.15542016568));
#82617=CARTESIAN_POINT('Origin',(-4.35,-1.95899712601,-4.25542016568));
#82618=CARTESIAN_POINT('Origin',(-4.35,2.8773238354,-4.25542016568));
#82619=CARTESIAN_POINT('Origin',(-4.35,2.8773238354,-3.65542016568));
#82620=CARTESIAN_POINT('',(-4.35,3.3773238354,-3.65542016568));
#82621=CARTESIAN_POINT('Origin',(-4.35,2.8773238354,-3.65542016568));
#82622=CARTESIAN_POINT('Origin',(-4.35,3.4773238354,-3.65542016568));
#82623=CARTESIAN_POINT('Origin',(-4.35,3.4773238354,0.294579834316));
#82624=CARTESIAN_POINT('',(-4.35,3.3773238354,1.84387696505));
#82625=CARTESIAN_POINT('',(-4.35,3.3773238354,-0.905771600316));
#82626=CARTESIAN_POINT('Origin',(-4.35,3.4773238354,1.84387696505));
#82627=CARTESIAN_POINT('Origin',(-4.35,2.8773238354,1.84387696505));
#82628=CARTESIAN_POINT('',(-4.35,2.8773238354,2.34387696505));
#82629=CARTESIAN_POINT('Origin',(-4.35,2.8773238354,1.84387696505));
#82630=CARTESIAN_POINT('Origin',(-4.35,2.8773238354,2.44387696505));
#82631=CARTESIAN_POINT('Origin',(-4.35,-1.95899712601,2.44387696505));
#82632=CARTESIAN_POINT('',(-4.35,-2.12788809108,2.34387696505));
#82633=CARTESIAN_POINT('',(-4.35,0.374717872161,2.34387696505));
#82634=CARTESIAN_POINT('Origin',(-4.35,-2.12788809108,2.44387696505));
#82635=CARTESIAN_POINT('Origin',(-4.35,-2.12788809108,3.34387696505));
#82636=CARTESIAN_POINT('',(-4.35,-2.56170009476,2.4428735547));
#82637=CARTESIAN_POINT('Origin',(-4.35,-2.12788809108,3.34387696505));
#82638=CARTESIAN_POINT('Origin',(-4.35,-2.51831889439,2.53297389574));
#82639=CARTESIAN_POINT('Origin',(-4.35,2.13070110951,0.294579834316));
#82640=CARTESIAN_POINT('',(-4.35,-7.88049121843,5.00374669681));
#82641=CARTESIAN_POINT('',(-4.35,-5.22109565659,3.72331012576));
#82642=CARTESIAN_POINT('Origin',(-4.35,-7.83711001806,5.09384703785));
#82643=CARTESIAN_POINT('Origin',(-4.35,-8.31430322211,4.10274328646));
#82644=CARTESIAN_POINT('Origin',(-4.35,-8.31430322211,4.10274328646));
#82645=CARTESIAN_POINT('Origin',(3.225,-8.31430322211,4.10274328646));
#82646=CARTESIAN_POINT('',(-4.2990272509,-7.88049121843,5.00374669681));
#82647=CARTESIAN_POINT('',(-4.32451362545,-7.88049121843,5.00374669681));
#82648=CARTESIAN_POINT('',(-4.29889875895,-8.31430322211008,5.10274332057));
#82649=CARTESIAN_POINT('Ctrl Pts',(-4.29889876134,-8.31430322211031,5.1027434229));
#82650=CARTESIAN_POINT('Ctrl Pts',(-4.2992163598671,-8.2759204184726,5.10274351089319));
#82651=CARTESIAN_POINT('Ctrl Pts',(-4.29939095950142,-8.23760601837549,
5.10053256059037));
#82652=CARTESIAN_POINT('Ctrl Pts',(-4.29949929792767,-8.199577020703,5.09614052938043));
#82653=CARTESIAN_POINT('Ctrl Pts',(-4.29956041494064,-8.17812370239259,
5.09366285052106));
#82654=CARTESIAN_POINT('Ctrl Pts',(-4.29959953479425,-8.15676118602362,
5.09049130118834));
#82655=CARTESIAN_POINT('Ctrl Pts',(-4.29962336909445,-8.13552816410012,
5.08663315284131));
#82656=CARTESIAN_POINT('Ctrl Pts',(-4.29966559839581,-8.09790777356408,
5.07979733606101));
#82657=CARTESIAN_POINT('Ctrl Pts',(-4.29966269432202,-8.06069331187253,
5.07080520434682));
#82658=CARTESIAN_POINT('Ctrl Pts',(-4.29961270179433,-8.02409853669487,
5.05970769169322));
#82659=CARTESIAN_POINT('Ctrl Pts',(-4.2995627202886,-7.98751182964539,5.04861262573191));
#82660=CARTESIAN_POINT('Ctrl Pts',(-4.2994656683763,-7.95154459699327,5.0354131084642));
#82661=CARTESIAN_POINT('Ctrl Pts',(-4.2992694321813,-7.91640705990306,5.02017373353442));
#82662=CARTESIAN_POINT('Ctrl Pts',(-4.29920200874686,-7.9043343970172,5.01493774230241));
#82663=CARTESIAN_POINT('Ctrl Pts',(-4.29912244160228,-7.89235964547437,
5.00946106597536));
#82664=CARTESIAN_POINT('Ctrl Pts',(-4.29902725090631,-7.88049121921695,
5.00374669718888));
#82665=CARTESIAN_POINT('',(-4.32444937589,-8.31430322211,5.10274328646));
#82666=CARTESIAN_POINT('Origin',(0.,-2.35608968258,2.34387696505));
#82667=CARTESIAN_POINT('',(4.225,-2.56170009476,2.4428735547));
#82668=CARTESIAN_POINT('',(-4.3,-6.28560647753,4.2358471116));
#82669=CARTESIAN_POINT('',(-4.3,-2.61831228762,2.47013099738));
#82670=CARTESIAN_POINT('Ctrl Pts',(-4.2990272509,-7.88049121843,5.00374669681));
#82671=CARTESIAN_POINT('Ctrl Pts',(-4.29860194904898,-7.84336279989873,
4.98587023435574));
#82672=CARTESIAN_POINT('Ctrl Pts',(-4.29807036319667,-7.8063193049477,4.96803466061349));
#82673=CARTESIAN_POINT('Ctrl Pts',(-4.29749123915026,-7.76934684031188,
4.95023328629991));
#82674=CARTESIAN_POINT('Ctrl Pts',(-4.29661357039136,-7.71331467008551,
4.92325511090297));
#82675=CARTESIAN_POINT('Ctrl Pts',(-4.29562842420427,-7.65745144851057,
4.89635828031341));
#82676=CARTESIAN_POINT('Ctrl Pts',(-4.29470009048654,-7.60171026056881,
4.86952020595908));
#82677=CARTESIAN_POINT('Ctrl Pts',(-4.29377028407366,-7.54588064561534,
4.84263955607304));
#82678=CARTESIAN_POINT('Ctrl Pts',(-4.29289746676361,-7.49017341724383,
4.8158178323467));
#82679=CARTESIAN_POINT('Ctrl Pts',(-4.29219442747521,-7.43454058879187,
4.78903193034465));
#82680=CARTESIAN_POINT('Ctrl Pts',(-4.29149095408814,-7.3788734092915,4.76222948911851));
#82681=CARTESIAN_POINT('Ctrl Pts',(-4.29095746147181,-7.32328068911448,
4.73546289822188));
#82682=CARTESIAN_POINT('Ctrl Pts',(-4.29065473399492,-7.26771400724003,
4.7087088442481));
#82683=CARTESIAN_POINT('Ctrl Pts',(-4.29035187162506,-7.21212256529347,
4.68194286888037));
#82684=CARTESIAN_POINT('Ctrl Pts',(-4.29027997715909,-7.15655715410882,
4.65518942682211));
#82685=CARTESIAN_POINT('Ctrl Pts',(-4.29044774917812,-7.10096941674446,
4.6284252355263));
#82686=CARTESIAN_POINT('Ctrl Pts',(-4.29052775589753,-7.07446086941765,
4.61566199195374));
#82687=CARTESIAN_POINT('Ctrl Pts',(-4.29066150240974,-7.04794724961644,
4.6028963061693));
#82688=CARTESIAN_POINT('Ctrl Pts',(-4.29084575810665,-7.02142335390664,
4.59012567283795));
#82689=CARTESIAN_POINT('Ctrl Pts',(-4.29123152417027,-6.96589172578971,
4.56338849709526));
#82690=CARTESIAN_POINT('Ctrl Pts',(-4.29184075891047,-6.91031984610482,
4.53663194126546));
#82691=CARTESIAN_POINT('Ctrl Pts',(-4.29260245682323,-6.85466578564437,
4.50983581716746));
#82692=CARTESIAN_POINT('Ctrl Pts',(-4.29336407793749,-6.79901733652759,
4.48304239479976));
#82693=CARTESIAN_POINT('Ctrl Pts',(-4.29427813122767,-6.74328668363906,
4.45620939309286));
#82694=CARTESIAN_POINT('Ctrl Pts',(-4.29522152510374,-6.68743327543012,
4.42931728747705));
#82695=CARTESIAN_POINT('Ctrl Pts',(-4.29540155763234,-6.67677449274567,
4.42418533369164));
#82696=CARTESIAN_POINT('Ctrl Pts',(-4.29558250634003,-6.66611124458006,
4.41905122987873));
#82697=CARTESIAN_POINT('Ctrl Pts',(-4.29576330024143,-6.65544325666937,
4.41391484398757));
#82698=CARTESIAN_POINT('Ctrl Pts',(-4.29671133096125,-6.59950342584761,
4.38698112788367));
#82699=CARTESIAN_POINT('Ctrl Pts',(-4.29766075533132,-6.54342366948845,
4.35998004088301));
#82700=CARTESIAN_POINT('Ctrl Pts',(-4.29842842934662,-6.48716607127935,
4.33289332720474));
#82701=CARTESIAN_POINT('Ctrl Pts',(-4.29919717698267,-6.43082979472131,
4.30576873174731));
#82702=CARTESIAN_POINT('Ctrl Pts',(-4.29978365749905,-6.37431514200558,
4.27855825235265));
#82703=CARTESIAN_POINT('Ctrl Pts',(-4.29995176543971,-6.31758659819914,
4.25124478941713));
#82704=CARTESIAN_POINT('Ctrl Pts',(-4.29998333258852,-6.30693416633443,
4.24611589339078));
#82705=CARTESIAN_POINT('Ctrl Pts',(-4.3,-6.29627420060992,4.24098336998769));
#82706=CARTESIAN_POINT('Ctrl Pts',(-4.3,-6.28560647753,4.2358471116));
#82707=CARTESIAN_POINT('Origin',(4.225,-2.12788809108,3.34387696505));
#82708=CARTESIAN_POINT('',(-4.325,-2.12788809108,2.34387696505));
#82709=CARTESIAN_POINT('Origin',(0.,3.3773238354,2.34387696505));
#82710=CARTESIAN_POINT('',(4.225,2.8773238354,2.34387696505));
#82711=CARTESIAN_POINT('Origin',(4.225,2.8773238354,1.84387696505));
#82712=CARTESIAN_POINT('',(-4.325,3.3773238354,1.84387696505));
#82713=CARTESIAN_POINT('Origin',(0.,3.3773238354,-4.15542016568));
#82714=CARTESIAN_POINT('',(3.225,3.3773238354,-3.65542016568));
#82715=CARTESIAN_POINT('Origin',(3.225,2.8773238354,-3.65542016568));
#82716=CARTESIAN_POINT('Origin',(-4.3,2.8773238354,-3.65542016568));
#82717=CARTESIAN_POINT('Ctrl Pts',(-4.,3.0773238354,-3.65542016568));
#82718=CARTESIAN_POINT('Ctrl Pts',(-4.,3.0773238354,-3.85542016568));
#82719=CARTESIAN_POINT('Ctrl Pts',(-4.,2.8773238354,-3.85542016568));
#82720=CARTESIAN_POINT('Ctrl Pts',(-4.,3.3773238354,-3.65542016568));
#82721=CARTESIAN_POINT('Ctrl Pts',(-4.,3.3773238354,-4.15542016568));
#82722=CARTESIAN_POINT('Ctrl Pts',(-4.,2.8773238354,-4.15542016568));
#82723=CARTESIAN_POINT('Ctrl Pts',(-4.3,3.3773238354,-3.65542016568));
#82724=CARTESIAN_POINT('Ctrl Pts',(-4.3,3.3773238354,-4.15542016568));
#82725=CARTESIAN_POINT('Ctrl Pts',(-4.3,2.8773238354,-4.15542016568));
#82726=CARTESIAN_POINT('',(-4.,2.8773238354,-3.85542016568));
#82727=CARTESIAN_POINT('Origin',(-4.3,2.8773238354,-3.85542016568));
#82728=CARTESIAN_POINT('Origin',(-4.,2.8773238354,-3.65542016568));
#82729=CARTESIAN_POINT('Origin',(-4.3,-3.42065492897,-3.85542016568));
#82730=CARTESIAN_POINT('',(-4.,-8.14391944342,-3.85542016568));
#82731=CARTESIAN_POINT('Origin',(-4.29787870966756,-8.14391943179286,-3.85754145569448));
#82732=CARTESIAN_POINT('',(-4.,-2.63329780401,-3.85542016568));
#82733=CARTESIAN_POINT('Ctrl Pts',(-4.29232316291,-8.70602833393,-4.15542016568));
#82734=CARTESIAN_POINT('Ctrl Pts',(-4.20764023978,-8.70455758206,-4.15542016896));
#82735=CARTESIAN_POINT('Ctrl Pts',(-4.12295731665,-8.70308683019,-4.12553116451));
#82736=CARTESIAN_POINT('Ctrl Pts',(-4.05251768323,-8.70186345223,-4.06549009434));
#82737=CARTESIAN_POINT('Ctrl Pts',(-4.00958634297,-8.70111783143,-3.98660373227));
#82738=CARTESIAN_POINT('Ctrl Pts',(-3.99616158804,-8.70088467363,-3.90297907486));
#82739=CARTESIAN_POINT('Ctrl Pts',(-4.2942593567,-8.59454665965,-4.15542016568));
#82740=CARTESIAN_POINT('Ctrl Pts',(-4.20834579354,-8.59289747109,-4.15542016627));
#82741=CARTESIAN_POINT('Ctrl Pts',(-4.12243223039,-8.59124828254,-4.12466052278));
#82742=CARTESIAN_POINT('Ctrl Pts',(-4.05139392587,-8.58988386074,-4.06285702325));
#82743=CARTESIAN_POINT('Ctrl Pts',(-4.00903053768,-8.58906847866,-3.98200796497));
#82744=CARTESIAN_POINT('Ctrl Pts',(-3.99712968313,-8.58883688841,-3.89688931333));
#82745=CARTESIAN_POINT('Ctrl Pts',(-4.29645983294,-8.48273103918,-4.15542016568));
#82746=CARTESIAN_POINT('Ctrl Pts',(-4.20896023779,-8.48105918371,-4.15542015758));
#82747=CARTESIAN_POINT('Ctrl Pts',(-4.12146064264,-8.47938732823,-4.12352488429));
#82748=CARTESIAN_POINT('Ctrl Pts',(-4.04967388507,-8.47801593608,-4.05942126033));
#82749=CARTESIAN_POINT('Ctrl Pts',(-4.00810176319,-8.47722229641,-3.97603783242));
#82750=CARTESIAN_POINT('Ctrl Pts',(-3.99822990786,-8.47703468918,-3.88903180855));
#82751=CARTESIAN_POINT('Ctrl Pts',(-4.29855844641,-8.37042692805,-4.15542016568));
#82752=CARTESIAN_POINT('Ctrl Pts',(-4.20912872342,-8.36895891499,-4.15542016568));
#82753=CARTESIAN_POINT('Ctrl Pts',(-4.11969900043,-8.36749090194,-4.12211547602));
#82754=CARTESIAN_POINT('Ctrl Pts',(-4.04704750378,-8.36630239191,-4.05515458588));
#82755=CARTESIAN_POINT('Ctrl Pts',(-4.00655550671,-8.36564940222,-3.96867720994));
#82756=CARTESIAN_POINT('Ctrl Pts',(-3.99927927276,-8.3655474023,-3.87944960348));
#82757=CARTESIAN_POINT('Ctrl Pts',(-4.3,-8.25752787941,-4.15542016568));
#82758=CARTESIAN_POINT('Ctrl Pts',(-4.20831114128,-8.25657123296,-4.15542016568));
#82759=CARTESIAN_POINT('Ctrl Pts',(-4.11662228256,-8.2556145865,-4.12041892129));
#82760=CARTESIAN_POINT('Ctrl Pts',(-4.04304033238,-8.25485845437,-4.05001401514));
#82761=CARTESIAN_POINT('Ctrl Pts',(-4.00401954353,-8.25448277917,-3.95990362884));
#82762=CARTESIAN_POINT('Ctrl Pts',(-4.,-8.25448277917,-3.86821477012));
#82763=CARTESIAN_POINT('Ctrl Pts',(-4.3,-8.14391944342,-4.15542016568));
#82764=CARTESIAN_POINT('Ctrl Pts',(-4.20575222039,-8.14391944342,-4.15542016568));
#82765=CARTESIAN_POINT('Ctrl Pts',(-4.11150444078,-8.14391944342,-4.11840914918));
#82766=CARTESIAN_POINT('Ctrl Pts',(-4.0370110165,-8.14391944342,-4.0439157249));
#82767=CARTESIAN_POINT('Ctrl Pts',(-4.,-8.14391944342,-3.94966794529));
#82768=CARTESIAN_POINT('Ctrl Pts',(-4.,-8.14391944342,-3.85542016568));
#82769=CARTESIAN_POINT('',(-3.99616160426685,-8.70088467346877,-3.90297923414786));
#82770=CARTESIAN_POINT('Origin',(-4.290691026855,-8.70599993058013,-3.85733562503364));
#82771=CARTESIAN_POINT('Ctrl Pts',(-4.,-8.14391944342,-3.85542016568));
#82772=CARTESIAN_POINT('Ctrl Pts',(-4.,-8.21619147164719,-3.86378362547669));
#82773=CARTESIAN_POINT('Ctrl Pts',(-3.99963494167047,-8.28873626415572,
-3.87134899206184));
#82774=CARTESIAN_POINT('Ctrl Pts',(-3.99911352626311,-8.36160108492365,
-3.87807113866823));
#82775=CARTESIAN_POINT('Ctrl Pts',(-3.99857374958904,-8.43703178769067,
-3.88503000080881));
#82776=CARTESIAN_POINT('Ctrl Pts',(-3.99786619096606,-8.51280461194599,
-3.89108515684303));
#82777=CARTESIAN_POINT('Ctrl Pts',(-3.99716685654696,-8.58897211220517,
-3.89618805925311));
#82778=CARTESIAN_POINT('Ctrl Pts',(-3.99682523423041,-8.62617965865753,
-3.89868080849417));
#82779=CARTESIAN_POINT('Ctrl Pts',(-3.9964847718308,-8.66348146771974,-3.9009463498971));
#82780=CARTESIAN_POINT('Ctrl Pts',(-3.99616161341551,-8.70088467121112,
-3.90297923261801));
#82781=CARTESIAN_POINT('Ctrl Pts',(-3.69999999774,-9.41827086749,-4.15542016568));
#82782=CARTESIAN_POINT('Ctrl Pts',(-3.69999999833,-9.34659890209,-4.15542016568));
#82783=CARTESIAN_POINT('Ctrl Pts',(-3.69999999892,-9.2749269367,-4.13401653812));
#82784=CARTESIAN_POINT('Ctrl Pts',(-3.69999999944,-9.21183540432,-4.09110601764));
#82785=CARTESIAN_POINT('Ctrl Pts',(-3.69999999982,-9.16559336719,-4.03231265157));
#82786=CARTESIAN_POINT('Ctrl Pts',(-3.70000000003,-9.13925764692,-3.96565456539));
#82787=CARTESIAN_POINT('Ctrl Pts',(-3.81412909821,-9.41827089013,-4.15542016568));
#82788=CARTESIAN_POINT('Ctrl Pts',(-3.79947056194,-9.34659892134,-4.15542016565));
#82789=CARTESIAN_POINT('Ctrl Pts',(-3.78481202566,-9.27492695255,-4.13401653803));
#82790=CARTESIAN_POINT('Ctrl Pts',(-3.77190837788,-9.21183541723,-4.09110601746));
#82791=CARTESIAN_POINT('Ctrl Pts',(-3.76245084042,-9.16559337792,-4.03231265129));
#82792=CARTESIAN_POINT('Ctrl Pts',(-3.75706459059,-9.13925765647,-3.96565456502));
#82793=CARTESIAN_POINT('Ctrl Pts',(-3.92823594404,-9.38909765086,-4.15542016568));
#82794=CARTESIAN_POINT('Ctrl Pts',(-3.89892199959,-9.32091627439,-4.15542016461));
#82795=CARTESIAN_POINT('Ctrl Pts',(-3.86960805513,-9.25273489792,-4.13385699888));
#82796=CARTESIAN_POINT('Ctrl Pts',(-3.84380320278,-9.19278171906,-4.0906252646));
#82797=CARTESIAN_POINT('Ctrl Pts',(-3.82488943837,-9.14898176867,-4.03143501908));
#82798=CARTESIAN_POINT('Ctrl Pts',(-3.81411802643,-9.12422889542,-3.96440816956));
#82799=CARTESIAN_POINT('Ctrl Pts',(-4.03302804821,-9.33107957038,-4.15542016568));
#82800=CARTESIAN_POINT('Ctrl Pts',(-3.99017706972,-9.2696193654,-4.1554201695));
#82801=CARTESIAN_POINT('Ctrl Pts',(-3.94732609124,-9.20815916043,-4.13359925186));
#82802=CARTESIAN_POINT('Ctrl Pts',(-3.90964076698,-9.15426319663,-4.0898484638));
#82803=CARTESIAN_POINT('Ctrl Pts',(-3.8820963349,-9.11520770945,-4.03001850758));
#82804=CARTESIAN_POINT('Ctrl Pts',(-3.86651403782,-9.0935734628,-3.96239691009));
#82805=CARTESIAN_POINT('Ctrl Pts',(-4.18747374061,-9.18016437508,-4.15542016568));
#82806=CARTESIAN_POINT('Ctrl Pts',(-4.12388018645,-9.13700016797,-4.15542016252));
#82807=CARTESIAN_POINT('Ctrl Pts',(-4.0602866323,-9.09383596087,-4.13249096908));
#82808=CARTESIAN_POINT('Ctrl Pts',(-4.00475631151,-9.05633061601,-4.08650843459));
#82809=CARTESIAN_POINT('Ctrl Pts',(-3.96503122609,-9.029900996,-4.02393293739));
#82810=CARTESIAN_POINT('Ctrl Pts',(-3.94373685893,-9.0162718551,-3.9537856064));
#82811=CARTESIAN_POINT('Ctrl Pts',(-4.26723541157,-8.98063713586,-4.15542016568));
#82812=CARTESIAN_POINT('Ctrl Pts',(-4.19077919927,-8.95915602901,-4.1554201683));
#82813=CARTESIAN_POINT('Ctrl Pts',(-4.11432298698,-8.93767492216,-4.13000304884));
#82814=CARTESIAN_POINT('Ctrl Pts',(-4.04869892936,-8.91937700045,-4.07900263159));
#82815=CARTESIAN_POINT('Ctrl Pts',(-4.00420277032,-8.90727654877,-4.01043652908));
#82816=CARTESIAN_POINT('Ctrl Pts',(-3.98361771521,-8.90210958415,-3.93506389031));
#82817=CARTESIAN_POINT('Ctrl Pts',(-4.28448738522,-8.88291546038,-4.15542016568));
#82818=CARTESIAN_POINT('Ctrl Pts',(-4.2038128468,-8.87211558957,-4.15542016079));
#82819=CARTESIAN_POINT('Ctrl Pts',(-4.12313830838,-8.86131571876,-4.12815293378));
#82820=CARTESIAN_POINT('Ctrl Pts',(-4.05474416619,-8.85231492765,-4.07341965826));
#82821=CARTESIAN_POINT('Ctrl Pts',(-4.01023278232,-8.84679291313,-4.00043036345));
#82822=CARTESIAN_POINT('Ctrl Pts',(-3.99224364397,-8.84501961539,-3.92126984866));
#82823=CARTESIAN_POINT('Ctrl Pts',(-4.2908008405,-8.79368075155,-4.15542016568));
#82824=CARTESIAN_POINT('Ctrl Pts',(-4.20683195096,-8.78806573108,-4.15542016568));
#82825=CARTESIAN_POINT('Ctrl Pts',(-4.12286306143,-8.78245071061,-4.12598423857));
#82826=CARTESIAN_POINT('Ctrl Pts',(-4.05279621082,-8.77777630692,-4.06686040464));
#82827=CARTESIAN_POINT('Ctrl Pts',(-4.00960658253,-8.77491887358,-3.98899545804));
#82828=CARTESIAN_POINT('Ctrl Pts',(-3.99540042025,-8.7740131878,-3.9061483086));
#82829=CARTESIAN_POINT('Ctrl Pts',(-4.29232317424,-8.70602837163,-4.15542016568));
#82830=CARTESIAN_POINT('Ctrl Pts',(-4.20764026079,-8.70455761115,-4.15542016568));
#82831=CARTESIAN_POINT('Ctrl Pts',(-4.12295734733,-8.70308685067,-4.12553116999));
#82832=CARTESIAN_POINT('Ctrl Pts',(-4.05251771609,-8.70186346543,-4.06549012145));
#82833=CARTESIAN_POINT('Ctrl Pts',(-4.00958636427,-8.70111783998,-3.98660378483));
#82834=CARTESIAN_POINT('Ctrl Pts',(-3.99616158712,-8.70088468041,-3.90297914754));
#82835=CARTESIAN_POINT('Ctrl Pts',(-3.99616160115866,-8.70088468065382,
-3.90297923498851));
#82836=CARTESIAN_POINT('Ctrl Pts',(-3.99604551141223,-8.71203767637363,
-3.9034625548241));
#82837=CARTESIAN_POINT('Ctrl Pts',(-3.99586488182614,-8.72292685065226,
-3.90426647885834));
#82838=CARTESIAN_POINT('Ctrl Pts',(-3.99560115130509,-8.73359011569891,
-3.90528436153708));
#82839=CARTESIAN_POINT('Ctrl Pts',(-3.99529801267143,-8.74584674638279,
-3.90645434202788));
#82840=CARTESIAN_POINT('Ctrl Pts',(-3.99488561757464,-8.75780627735821,
-3.90790775425564));
#82841=CARTESIAN_POINT('Ctrl Pts',(-3.99432792915694,-8.76955639086698,
-3.90954414641858));
#82842=CARTESIAN_POINT('Ctrl Pts',(-3.99368017119247,-8.78320420811978,
-3.91144482432923));
#82843=CARTESIAN_POINT('Ctrl Pts',(-3.99283783198393,-8.79657147264791,
-3.91359388993806));
#82844=CARTESIAN_POINT('Ctrl Pts',(-3.99171828615615,-8.80980380168097,
-3.91589197001634));
#82845=CARTESIAN_POINT('Ctrl Pts',(-3.99064600082351,-8.82247754132309,
-3.9180930389677));
#82846=CARTESIAN_POINT('Ctrl Pts',(-3.98932011806426,-8.83502840719307,
-3.92043291784419));
#82847=CARTESIAN_POINT('Ctrl Pts',(-3.98763067900264,-8.84756915200607,
-3.92284258058646));
#82848=CARTESIAN_POINT('Ctrl Pts',(-3.98684406614188,-8.85340819727119,
-3.92396453387038));
#82849=CARTESIAN_POINT('Ctrl Pts',(-3.98597803251126,-8.85924475074751,
-3.92510169021808));
#82850=CARTESIAN_POINT('Ctrl Pts',(-3.98501789856444,-8.86508845323168,
-3.92624698376165));
#82851=CARTESIAN_POINT('Ctrl Pts',(-3.98252059670421,-8.880287883616,-3.92922588447268));
#82852=CARTESIAN_POINT('Ctrl Pts',(-3.97939450198513,-8.89550115214628,
-3.93225214634863));
#82853=CARTESIAN_POINT('Ctrl Pts',(-3.97537936433567,-8.91066978033972,
-3.93515747744907));
#82854=CARTESIAN_POINT('Ctrl Pts',(-3.97262832208053,-8.92106283302081,
-3.93714811620677));
#82855=CARTESIAN_POINT('Ctrl Pts',(-3.96945852442506,-8.93143598728981,
-3.93908154714824));
#82856=CARTESIAN_POINT('Ctrl Pts',(-3.96577774861011,-8.941769529366,-3.94091664769336));
#82857=CARTESIAN_POINT('Ctrl Pts',(-3.96216893175439,-8.95190105127839,
-3.94271587212651));
#82858=CARTESIAN_POINT('Ctrl Pts',(-3.95807061154141,-8.96198653511246,
-3.94441767599072));
#82859=CARTESIAN_POINT('Ctrl Pts',(-3.95341373784437,-8.97197051163173,
-3.94600679205796));
#82860=CARTESIAN_POINT('Ctrl Pts',(-3.94932091006251,-8.9807452173957,-3.94740343255365));
#82861=CARTESIAN_POINT('Ctrl Pts',(-3.94479769632574,-8.98944092795093,
-3.94871261919628));
#82862=CARTESIAN_POINT('Ctrl Pts',(-3.93980261645734,-8.99801101188341,
-3.94995603040284));
#82863=CARTESIAN_POINT('Ctrl Pts',(-3.93763249450409,-9.00173430115467,
-3.95049623276745));
#82864=CARTESIAN_POINT('Ctrl Pts',(-3.93537324066519,-9.00543373618864,
-3.95102461961947));
#82865=CARTESIAN_POINT('Ctrl Pts',(-3.93302131928633,-9.00910465172099,
-3.95154035015494));
#82866=CARTESIAN_POINT('Ctrl Pts',(-3.93266333651296,-9.00966339681123,
-3.9516188488025));
#82867=CARTESIAN_POINT('Ctrl Pts',(-3.93230320820075,-9.01022147916087,
-3.95169705425756));
#82868=CARTESIAN_POINT('Ctrl Pts',(-3.93194092287047,-9.01077888093755,
-3.95177496369907));
#82869=CARTESIAN_POINT('Ctrl Pts',(-3.93176419291978,-9.01105079255052,
-3.95181296946581));
#82870=CARTESIAN_POINT('Ctrl Pts',(-3.93158234635872,-9.01132962742367,
-3.95185189524054));
#82871=CARTESIAN_POINT('Ctrl Pts',(-3.93139478338652,-9.01161613949368,
-3.95189183812612));
#82872=CARTESIAN_POINT('Ctrl Pts',(-3.93028310063817,-9.01331429196849,
-3.95212857897266));
#82873=CARTESIAN_POINT('Ctrl Pts',(-3.92899148176813,-9.0152425934793,-3.95239515355946));
#82874=CARTESIAN_POINT('Ctrl Pts',(-3.92785226325583,-9.01690526443413,
-3.95262308942227));
#82875=CARTESIAN_POINT('Ctrl Pts',(-3.92698904941135,-9.01816511104963,
-3.95279580202334));
#82876=CARTESIAN_POINT('Ctrl Pts',(-3.92621450008615,-9.01927362386826,
-3.95294664455499));
#82877=CARTESIAN_POINT('Ctrl Pts',(-3.92568436011083,-9.0200266935362,-3.95304883021392));
#82878=CARTESIAN_POINT('Ctrl Pts',(-3.9185903818677,-9.03010376768366,-3.95441621029272));
#82879=CARTESIAN_POINT('Ctrl Pts',(-3.91069606779733,-9.04001012485587,
-3.95571759994867));
#82880=CARTESIAN_POINT('Ctrl Pts',(-3.90191649924126,-9.04958397296082,
-3.95692033378577));
#82881=CARTESIAN_POINT('Ctrl Pts',(-3.89352540383185,-9.05873420310834,
-3.95806984976879));
#82882=CARTESIAN_POINT('Ctrl Pts',(-3.88432499148419,-9.06758068841357,
-3.9591292538823));
#82883=CARTESIAN_POINT('Ctrl Pts',(-3.87427212029623,-9.07594769332381,
-3.9600791735614));
#82884=CARTESIAN_POINT('Ctrl Pts',(-3.86461090920672,-9.08398871952552,
-3.9609920843474));
#82885=CARTESIAN_POINT('Ctrl Pts',(-3.85416187252658,-9.09158662465468,
-3.96180401029878));
#82886=CARTESIAN_POINT('Ctrl Pts',(-3.84292435692288,-9.09855486626783,
-3.96250537695381));
#82887=CARTESIAN_POINT('Ctrl Pts',(-3.84110078825937,-9.0996856381834,-3.96261919127886));
#82888=CARTESIAN_POINT('Ctrl Pts',(-3.83925654865879,-9.10079976768752,
-3.96273010799853));
#82889=CARTESIAN_POINT('Ctrl Pts',(-3.83739174650389,-9.10189638836945,
-3.96283810094468));
#82890=CARTESIAN_POINT('Ctrl Pts',(-3.82591638674565,-9.10864461997696,
-3.96350265289469));
#82891=CARTESIAN_POINT('Ctrl Pts',(-3.81364052793048,-9.11472436781836,
-3.96401517490357));
#82892=CARTESIAN_POINT('Ctrl Pts',(-3.80060602177208,-9.119932670966,-3.96441142708227));
#82893=CARTESIAN_POINT('Ctrl Pts',(-3.78769322884257,-9.12509234017344,
-3.96480397914901));
#82894=CARTESIAN_POINT('Ctrl Pts',(-3.77403546873179,-9.12939595950774,
-3.96508294623434));
#82895=CARTESIAN_POINT('Ctrl Pts',(-3.75971878916075,-9.13262369144836,
-3.96527859680989));
#82896=CARTESIAN_POINT('Ctrl Pts',(-3.7460532179828,-9.13570462934035,-3.96546534939123));
#82897=CARTESIAN_POINT('Ctrl Pts',(-3.73178737468922,-9.13780386141483,
-3.96557697803066));
#82898=CARTESIAN_POINT('Ctrl Pts',(-3.71703967484152,-9.13872606991317,
-3.9656262756991));
#82899=CARTESIAN_POINT('Ctrl Pts',(-3.71142639112646,-9.13907708179971,
-3.96564503942513));
#82900=CARTESIAN_POINT('Ctrl Pts',(-3.7057437580401,-9.13925764788124,-3.96565456535276));
#82901=CARTESIAN_POINT('Ctrl Pts',(-3.70000000003,-9.13925764692,-3.96565456539));
#82902=CARTESIAN_POINT('Ctrl Pts',(-3.7,-9.13925764782849,-3.96565456816803));
#82903=CARTESIAN_POINT('Ctrl Pts',(-3.7,-9.02827749416282,-3.68475377230609));
#82904=CARTESIAN_POINT('Ctrl Pts',(-3.7,-8.72799905369119,-3.65227747615864));
#82905=CARTESIAN_POINT('Ctrl Pts',(-3.95543192421952,-9.13925764782849,
-3.96565456816803));
#82906=CARTESIAN_POINT('Ctrl Pts',(-3.95543192421952,-9.02827749416282,
-3.68475377230609));
#82907=CARTESIAN_POINT('Ctrl Pts',(-3.95543192421952,-8.72799905369119,
-3.65227747615864));
#82908=CARTESIAN_POINT('Ctrl Pts',(-3.99616160122642,-8.90473423916573,
-4.05831163541388));
#82909=CARTESIAN_POINT('Ctrl Pts',(-3.99616160122642,-8.84972443093161,
-3.919076840698));
#82910=CARTESIAN_POINT('Ctrl Pts',(-3.99616160122642,-8.70088467101431,
-3.90297923437636));
#82911=CARTESIAN_POINT('',(-3.7,-8.7279990537,-3.65227747616));
#82912=CARTESIAN_POINT('Origin',(-3.7,-8.67423561284,-4.1493785649));
#82913=CARTESIAN_POINT('Origin',(-3.7,-8.69574098918,-3.9505381294));
#82914=CARTESIAN_POINT('Origin',(3.,-8.67423561284,-4.1493785649));
#82915=CARTESIAN_POINT('',(0.,-8.7279990537,-3.65227747616));
#82916=CARTESIAN_POINT('Origin',(0.,-9.17423561284,0.47366156039));
#82917=CARTESIAN_POINT('',(-3.7,-8.7279990537,4.59960059693));
#82918=CARTESIAN_POINT('',(3.,-8.7279990537,4.59960059693));
#82919=CARTESIAN_POINT('Origin',(-3.7,-9.17423561284,0.47366156039));
#82920=CARTESIAN_POINT('Origin',(3.,-8.67423561284,5.09670168568));
#82921=CARTESIAN_POINT('',(-3.7,-9.13925764671,4.9129776861));
#82922=CARTESIAN_POINT('',(3.225,-9.13925764673,4.91297768617));
#82923=CARTESIAN_POINT('Origin',(-3.7,-8.67423561284,5.09670168568));
#82924=CARTESIAN_POINT('Origin',(3.225,-9.41827086707,4.80274328646));
#82925=CARTESIAN_POINT('',(-3.69999999774,-9.41827086749,5.10274328646));
#82926=CARTESIAN_POINT('',(-3.,-9.41827086707,5.10274328646));
#82927=CARTESIAN_POINT('Origin',(-3.69999999763766,-9.41833116541154,4.80265462953655));
#82928=CARTESIAN_POINT('Origin',(0.,-8.08610163061,5.10274328646));
#82929=CARTESIAN_POINT('',(-4.29232279670749,-8.70602826446416,5.10274328645992));
#82930=CARTESIAN_POINT('Ctrl Pts',(-4.29232279844,-8.70602816471,5.10274328646));
#82931=CARTESIAN_POINT('Ctrl Pts',(-4.29367604164,-8.62810126572,5.10274328646));
#82932=CARTESIAN_POINT('Ctrl Pts',(-4.29515862692,-8.55000353482,5.10274328646));
#82933=CARTESIAN_POINT('Ctrl Pts',(-4.2966466112,-8.47169636018,5.10274328646));
#82934=CARTESIAN_POINT('Ctrl Pts',(-4.29796673138,-8.39314927373,5.10274328646));
#82935=CARTESIAN_POINT('Ctrl Pts',(-4.29889875178,-8.31430322211,5.10274328646));
#82936=CARTESIAN_POINT('Ctrl Pts',(-3.69999999774,-9.41827086749,5.10274328646));
#82937=CARTESIAN_POINT('Ctrl Pts',(-3.73058948857333,-9.41827087355667,
5.10274328646));
#82938=CARTESIAN_POINT('Ctrl Pts',(-3.76117302676985,-9.41574705670535,
5.10274328662896));
#82939=CARTESIAN_POINT('Ctrl Pts',(-3.79135695696247,-9.41074020445563,
5.10274328606016));
#82940=CARTESIAN_POINT('Ctrl Pts',(-3.8215408871551,-9.40573335220591,5.10274328549136));
#82941=CARTESIAN_POINT('Ctrl Pts',(-3.85132370712135,-9.39824319698092,
5.10274328437385));
#82942=CARTESIAN_POINT('Ctrl Pts',(-3.880310581398,-9.38836645220521,5.1027432782161));
#82943=CARTESIAN_POINT('Ctrl Pts',(-3.90707199290093,-9.37924799297674,
5.1027432725311));
#82944=CARTESIAN_POINT('Ctrl Pts',(-3.93315644396342,-9.36809987699747,
5.10274326252178));
#82945=CARTESIAN_POINT('Ctrl Pts',(-3.95827561771127,-9.35505208010836,
5.10274325269434));
#82946=CARTESIAN_POINT('Ctrl Pts',(-3.98223829836866,-9.34260500707664,
5.10274324331936));
#82947=CARTESIAN_POINT('Ctrl Pts',(-4.00532196797495,-9.32842939224294,
5.10274323477061));
#82948=CARTESIAN_POINT('Ctrl Pts',(-4.02730698337273,-9.31267452069528,
5.10274323470365));
#82949=CARTESIAN_POINT('Ctrl Pts',(-4.0342532243783,-9.30769671500346,5.1027432346825));
#82950=CARTESIAN_POINT('Ctrl Pts',(-4.04109006204254,-9.30256152719756,
5.10274323548998));
#82951=CARTESIAN_POINT('Ctrl Pts',(-4.04781138042469,-9.29727441845877,
5.10274323721421));
#82952=CARTESIAN_POINT('Ctrl Pts',(-4.06816544935236,-9.28126354535637,
5.10274324243566));
#82953=CARTESIAN_POINT('Ctrl Pts',(-4.08745353683921,-9.26386507535306,
5.10274325797042));
#82954=CARTESIAN_POINT('Ctrl Pts',(-4.1055168903408,-9.24523724841711,5.10274326872092));
#82955=CARTESIAN_POINT('Ctrl Pts',(-4.12268030159011,-9.22753748661184,
5.10274327893581));
#82956=CARTESIAN_POINT('Ctrl Pts',(-4.13873762061326,-9.20872790766285,
5.10274328434029));
#82957=CARTESIAN_POINT('Ctrl Pts',(-4.1535845819758,-9.18897826222551,5.10274328574875));
#82958=CARTESIAN_POINT('Ctrl Pts',(-4.16272152564545,-9.17682416594611,
5.10274328661553));
#82959=CARTESIAN_POINT('Ctrl Pts',(-4.17140072073273,-9.16431470638581,
5.10274328646));
#82960=CARTESIAN_POINT('Ctrl Pts',(-4.17960523291625,-9.15149611025241,
5.10274328646));
#82961=CARTESIAN_POINT('Ctrl Pts',(-4.18942766527051,-9.13614970201014,
5.10274328646));
#82962=CARTESIAN_POINT('Ctrl Pts',(-4.19857745049624,-9.12036311945856,
5.10274328646));
#82963=CARTESIAN_POINT('Ctrl Pts',(-4.20701878194007,-9.10419983822068,
5.10274328646));
#82964=CARTESIAN_POINT('Ctrl Pts',(-4.21621021747847,-9.08660027367622,
5.10274328646));
#82965=CARTESIAN_POINT('Ctrl Pts',(-4.22456152722091,-9.06855481897592,
5.10274328646));
#82966=CARTESIAN_POINT('Ctrl Pts',(-4.2320738661817,-9.05018712924208,5.10274328646));
#82967=CARTESIAN_POINT('Ctrl Pts',(-4.23525034335279,-9.04242063368992,
5.10274328646));
#82968=CARTESIAN_POINT('Ctrl Pts',(-4.23827738137825,-9.03459693600601,
5.10274328646));
#82969=CARTESIAN_POINT('Ctrl Pts',(-4.24115737109239,-9.02672676812149,
5.10274328646));
#82970=CARTESIAN_POINT('Ctrl Pts',(-4.24909569801083,-9.00503364704426,
5.10274328646));
#82971=CARTESIAN_POINT('Ctrl Pts',(-4.25591706153315,-8.98297603570749,
5.10274328646));
#82972=CARTESIAN_POINT('Ctrl Pts',(-4.26171659160653,-8.96076940630961,
5.10274328646));
#82973=CARTESIAN_POINT('Ctrl Pts',(-4.26455589904718,-8.94989758613051,
5.10274328646));
#82974=CARTESIAN_POINT('Ctrl Pts',(-4.26715114281098,-8.93899011197066,
5.10274328646));
#82975=CARTESIAN_POINT('Ctrl Pts',(-4.26951780859379,-8.92807096217797,
5.10274328646));
#82976=CARTESIAN_POINT('Ctrl Pts',(-4.27382084868247,-8.90821790999222,
5.10274328646));
#82977=CARTESIAN_POINT('Ctrl Pts',(-4.27736537389317,-8.88833607622953,
5.10274328652144));
#82978=CARTESIAN_POINT('Ctrl Pts',(-4.28025710062774,-8.868557900564,5.10274328639925));
#82979=CARTESIAN_POINT('Ctrl Pts',(-4.28203791090249,-8.85637791895645,
5.102743286324));
#82980=CARTESIAN_POINT('Ctrl Pts',(-4.2835716533847,-8.84423662612072,5.10274328620522));
#82981=CARTESIAN_POINT('Ctrl Pts',(-4.2848866086288,-8.83215545542406,5.10274328535497));
#82982=CARTESIAN_POINT('Ctrl Pts',(-4.28680275059482,-8.81455087285411,
5.102743284116));
#82983=CARTESIAN_POINT('Ctrl Pts',(-4.28827698219617,-8.79709218114212,
5.10274328404483));
#82984=CARTESIAN_POINT('Ctrl Pts',(-4.28939927179632,-8.77979151596189,
5.10274328478464));
#82985=CARTESIAN_POINT('Ctrl Pts',(-4.29044254900022,-8.76370886706949,
5.10274328547236));
#82986=CARTESIAN_POINT('Ctrl Pts',(-4.29118189695424,-8.74776302279939,
5.10274328622038));
#82987=CARTESIAN_POINT('Ctrl Pts',(-4.29168885063704,-8.73191886459746,
5.1027432863823));
#82988=CARTESIAN_POINT('Ctrl Pts',(-4.29196579590166,-8.72326331136879,
5.10274328647075));
#82989=CARTESIAN_POINT('Ctrl Pts',(-4.29217335586042,-8.71463728288328,
5.10274328645986));
#82990=CARTESIAN_POINT('Ctrl Pts',(-4.29232279496067,-8.70602836504273,
5.10274328645976));
#82991=CARTESIAN_POINT('Ctrl Pts',(-4.29232279844,-8.70602816471,5.10274328646));
#82992=CARTESIAN_POINT('Ctrl Pts',(-4.20763985549,-8.70455745139,5.10274332142));
#82993=CARTESIAN_POINT('Ctrl Pts',(-4.12295691253,-8.70308673807,5.07285428042));
#82994=CARTESIAN_POINT('Ctrl Pts',(-4.05251729593,-8.70186339274,5.01281309848));
#82995=CARTESIAN_POINT('Ctrl Pts',(-4.00958603902,-8.70111779311,4.93392659864));
#82996=CARTESIAN_POINT('Ctrl Pts',(-3.99616141568,-8.70088464377,4.85030182916));
#82997=CARTESIAN_POINT('Ctrl Pts',(-4.29367604164,-8.62810126572,5.10274328646));
#82998=CARTESIAN_POINT('Ctrl Pts',(-4.20813285855,-8.6265058463,5.10274333195));
#82999=CARTESIAN_POINT('Ctrl Pts',(-4.12258967546,-8.62491042687,5.07224568401));
#83000=CARTESIAN_POINT('Ctrl Pts',(-4.0517315901,-8.62358850977,5.01097248773));
#83001=CARTESIAN_POINT('Ctrl Pts',(-4.00919737959,-8.62279415849,4.93071397417));
#83002=CARTESIAN_POINT('Ctrl Pts',(-3.99683804383,-8.62256210931,4.84604483372));
#83003=CARTESIAN_POINT('Ctrl Pts',(-4.29515862692,-8.55000353482,5.10274328646));
#83004=CARTESIAN_POINT('Ctrl Pts',(-4.20858147867,-8.54835950303,5.10274332811));
#83005=CARTESIAN_POINT('Ctrl Pts',(-4.12200433041,-8.54671547124,5.07150754218));
#83006=CARTESIAN_POINT('Ctrl Pts',(-4.05065454881,-8.5453604781,5.00873951265));
#83007=CARTESIAN_POINT('Ctrl Pts',(-4.0086265191,-8.54456207669,4.92682955987));
#83008=CARTESIAN_POINT('Ctrl Pts',(-3.99757933996,-8.54435185028,4.84092376899));
#83009=CARTESIAN_POINT('Ctrl Pts',(-4.2966466112,-8.47169636018,5.10274328646));
#83010=CARTESIAN_POINT('Ctrl Pts',(-4.20886559395,-8.47010372313,5.10274328646));
#83011=CARTESIAN_POINT('Ctrl Pts',(-4.12108457671,-8.46851108607,5.0706369892));
#83012=CARTESIAN_POINT('Ctrl Pts',(-4.049181176,-8.4672075164,5.00610503411));
#83013=CARTESIAN_POINT('Ctrl Pts',(-4.00779063879,-8.46645935943,4.92226864646));
#83014=CARTESIAN_POINT('Ctrl Pts',(-3.99832332564,-8.46629167717,4.83495432364));
#83015=CARTESIAN_POINT('Ctrl Pts',(-4.29796673138,-8.39314927373,5.10274328646));
#83016=CARTESIAN_POINT('Ctrl Pts',(-4.20881731963,-8.39173518355,5.10274328646));
#83017=CARTESIAN_POINT('Ctrl Pts',(-4.11966790787,-8.39032109337,5.06963007213));
#83018=CARTESIAN_POINT('Ctrl Pts',(-4.04716501903,-8.3891735059,5.00305604873));
#83019=CARTESIAN_POINT('Ctrl Pts',(-4.00657458492,-8.38853640885,4.91702461127));
#83020=CARTESIAN_POINT('Ctrl Pts',(-3.99898336569,-8.38842527481,4.8281587616));
#83021=CARTESIAN_POINT('Ctrl Pts',(-4.29889875178,-8.31430322211,5.10274328646));
#83022=CARTESIAN_POINT('Ctrl Pts',(-4.20822334583,-8.31323136973,5.10274328646));
#83023=CARTESIAN_POINT('Ctrl Pts',(-4.11754793987,-8.31215951735,5.06848004433));
#83024=CARTESIAN_POINT('Ctrl Pts',(-4.04442178691,-8.31129511051,4.99957103487));
#83025=CARTESIAN_POINT('Ctrl Pts',(-4.00483540394,-8.3108271693,4.91108461112));
#83026=CARTESIAN_POINT('Ctrl Pts',(-3.99944937589,-8.31076350235,4.82056298519));
#83027=CARTESIAN_POINT('',(-3.9961616700265,-8.70088464035681,4.85030293837252));
#83028=CARTESIAN_POINT('Origin',(-4.2906912681792,-8.70600002892326,4.80465840215202));
#83029=CARTESIAN_POINT('',(-3.9994493766888,-8.31076354696256,4.82056300748371));
#83030=CARTESIAN_POINT('Origin',(-4.29696517402085,-8.31428035436309,4.80479513966836));
#83031=CARTESIAN_POINT('Ctrl Pts',(-3.9961615961339,-8.70088460680108,4.85030294889421));
#83032=CARTESIAN_POINT('Ctrl Pts',(-3.99678390426082,-8.62885486806307,
4.846388344858));
#83033=CARTESIAN_POINT('Ctrl Pts',(-3.99747548605133,-8.5569395249013,4.84159514513512));
#83034=CARTESIAN_POINT('Ctrl Pts',(-3.99810969192043,-8.48520158611709,
4.83595601816904));
#83035=CARTESIAN_POINT('Ctrl Pts',(-3.99862484060351,-8.42693075247652,
4.83137550421942));
#83036=CARTESIAN_POINT('Ctrl Pts',(-3.99910126161364,-8.36877776894241,
4.8262371302703));
#83037=CARTESIAN_POINT('Ctrl Pts',(-3.9994493766893,-8.31076354696257,4.82056300748368));
#83038=CARTESIAN_POINT('Ctrl Pts',(-3.69999999774,-9.41827086749,5.10274328646));
#83039=CARTESIAN_POINT('Ctrl Pts',(-3.69999999833,-9.34659890209,5.10274328646));
#83040=CARTESIAN_POINT('Ctrl Pts',(-3.69999999892,-9.2749269367,5.0813396589));
#83041=CARTESIAN_POINT('Ctrl Pts',(-3.69999999944,-9.21183540432,5.03842913842));
#83042=CARTESIAN_POINT('Ctrl Pts',(-3.69999999982,-9.16559336719,4.97963577235));
#83043=CARTESIAN_POINT('Ctrl Pts',(-3.70000000003,-9.13925764692,4.91297768617));
#83044=CARTESIAN_POINT('Ctrl Pts',(-3.81412909821,-9.41827089013,5.10274328646));
#83045=CARTESIAN_POINT('Ctrl Pts',(-3.79947056194,-9.34659892134,5.10274328643));
#83046=CARTESIAN_POINT('Ctrl Pts',(-3.78481202566,-9.27492695255,5.08133965881));
#83047=CARTESIAN_POINT('Ctrl Pts',(-3.77190837788,-9.21183541723,5.03842913824));
#83048=CARTESIAN_POINT('Ctrl Pts',(-3.76245084042,-9.16559337792,4.97963577207));
#83049=CARTESIAN_POINT('Ctrl Pts',(-3.75706459059,-9.13925765647,4.9129776858));
#83050=CARTESIAN_POINT('Ctrl Pts',(-3.92823594404,-9.38909765086,5.10274328646));
#83051=CARTESIAN_POINT('Ctrl Pts',(-3.89892199959,-9.32091627439,5.10274328539));
#83052=CARTESIAN_POINT('Ctrl Pts',(-3.86960805513,-9.25273489792,5.08118011966));
#83053=CARTESIAN_POINT('Ctrl Pts',(-3.84380320278,-9.19278171906,5.03794838538));
#83054=CARTESIAN_POINT('Ctrl Pts',(-3.82488943837,-9.14898176867,4.97875813986));
#83055=CARTESIAN_POINT('Ctrl Pts',(-3.81411802643,-9.12422889542,4.91173129034));
#83056=CARTESIAN_POINT('Ctrl Pts',(-4.03302804821,-9.33107957038,5.10274328646));
#83057=CARTESIAN_POINT('Ctrl Pts',(-3.99017706972,-9.2696193654,5.10274329028));
#83058=CARTESIAN_POINT('Ctrl Pts',(-3.94732609124,-9.20815916043,5.08092237264));
#83059=CARTESIAN_POINT('Ctrl Pts',(-3.90964076698,-9.15426319663,5.03717158458));
#83060=CARTESIAN_POINT('Ctrl Pts',(-3.8820963349,-9.11520770945,4.97734162836));
#83061=CARTESIAN_POINT('Ctrl Pts',(-3.86651403782,-9.0935734628,4.90972003087));
#83062=CARTESIAN_POINT('Ctrl Pts',(-4.18747374061,-9.18016437508,5.10274328646));
#83063=CARTESIAN_POINT('Ctrl Pts',(-4.12388018645,-9.13700016797,5.1027432833));
#83064=CARTESIAN_POINT('Ctrl Pts',(-4.0602866323,-9.09383596087,5.07981408986));
#83065=CARTESIAN_POINT('Ctrl Pts',(-4.00475631151,-9.05633061601,5.03383155537));
#83066=CARTESIAN_POINT('Ctrl Pts',(-3.96503122609,-9.029900996,4.97125605817));
#83067=CARTESIAN_POINT('Ctrl Pts',(-3.94373685893,-9.0162718551,4.90110872718));
#83068=CARTESIAN_POINT('Ctrl Pts',(-4.26723541157,-8.98063713586,5.10274328646));
#83069=CARTESIAN_POINT('Ctrl Pts',(-4.19077919927,-8.95915602901,5.10274328908));
#83070=CARTESIAN_POINT('Ctrl Pts',(-4.11432298698,-8.93767492216,5.07732616962));
#83071=CARTESIAN_POINT('Ctrl Pts',(-4.04869892936,-8.91937700045,5.02632575237));
#83072=CARTESIAN_POINT('Ctrl Pts',(-4.00420277032,-8.90727654877,4.95775964986));
#83073=CARTESIAN_POINT('Ctrl Pts',(-3.98361771521,-8.90210958415,4.88238701109));
#83074=CARTESIAN_POINT('Ctrl Pts',(-4.28448738522,-8.88291546038,5.10274328646));
#83075=CARTESIAN_POINT('Ctrl Pts',(-4.2038128468,-8.87211558957,5.10274328157));
#83076=CARTESIAN_POINT('Ctrl Pts',(-4.12313830838,-8.86131571876,5.07547605456));
#83077=CARTESIAN_POINT('Ctrl Pts',(-4.05474416619,-8.85231492765,5.02074277903));
#83078=CARTESIAN_POINT('Ctrl Pts',(-4.01023278232,-8.84679291313,4.94775348423));
#83079=CARTESIAN_POINT('Ctrl Pts',(-3.99224364397,-8.84501961539,4.86859296944));
#83080=CARTESIAN_POINT('Ctrl Pts',(-4.2908008405,-8.79368075155,5.10274328646));
#83081=CARTESIAN_POINT('Ctrl Pts',(-4.20683195096,-8.78806573108,5.10274328646));
#83082=CARTESIAN_POINT('Ctrl Pts',(-4.12286306143,-8.78245071061,5.07330735934));
#83083=CARTESIAN_POINT('Ctrl Pts',(-4.05279621082,-8.77777630692,5.01418352542));
#83084=CARTESIAN_POINT('Ctrl Pts',(-4.00960658253,-8.77491887358,4.93631857882));
#83085=CARTESIAN_POINT('Ctrl Pts',(-3.99540042025,-8.7740131878,4.85347142938));
#83086=CARTESIAN_POINT('Ctrl Pts',(-4.29232317424,-8.70602837163,5.10274328646));
#83087=CARTESIAN_POINT('Ctrl Pts',(-4.20764026079,-8.70455761115,5.10274328646));
#83088=CARTESIAN_POINT('Ctrl Pts',(-4.12295734733,-8.70308685067,5.07285429077));
#83089=CARTESIAN_POINT('Ctrl Pts',(-4.05251771609,-8.70186346543,5.01281324223));
#83090=CARTESIAN_POINT('Ctrl Pts',(-4.00958636427,-8.70111783998,4.93392690561));
#83091=CARTESIAN_POINT('Ctrl Pts',(-3.99616158712,-8.70088468041,4.85030226832));
#83092=CARTESIAN_POINT('Ctrl Pts',(-3.70000000003,-9.13925764692,4.91297768617));
#83093=CARTESIAN_POINT('Ctrl Pts',(-3.71529015207103,-9.13925764947887,
4.91297768607086));
#83094=CARTESIAN_POINT('Ctrl Pts',(-3.73014416026747,-9.13797639510877,
4.91291207427923));
#83095=CARTESIAN_POINT('Ctrl Pts',(-3.74442150434438,-9.1356118541454,4.91277684154045));
#83096=CARTESIAN_POINT('Ctrl Pts',(-3.75913917708147,-9.13317438819342,
4.91263743807842));
#83097=CARTESIAN_POINT('Ctrl Pts',(-3.77324400464638,-9.12958776148789,
4.91242293557063));
#83098=CARTESIAN_POINT('Ctrl Pts',(-3.78663328576126,-9.12507402641783,
4.91210731666113));
#83099=CARTESIAN_POINT('Ctrl Pts',(-3.8002070348353,-9.12049810432745,4.91178734937955));
#83100=CARTESIAN_POINT('Ctrl Pts',(-3.81304573279602,-9.11497046038793,
4.91136276950297));
#83101=CARTESIAN_POINT('Ctrl Pts',(-3.8250917003685,-9.10870418173369,4.91079849724977));
#83102=CARTESIAN_POINT('Ctrl Pts',(-3.8292814570418,-9.10652468202556,4.9106022354365));
#83103=CARTESIAN_POINT('Ctrl Pts',(-3.83337571956335,-9.10425559637984,
4.91038904836799));
#83104=CARTESIAN_POINT('Ctrl Pts',(-3.83737329592438,-9.10190509538605,
4.91015742089567));
#83105=CARTESIAN_POINT('Ctrl Pts',(-3.8488097273671,-9.09518068513249,4.90949477146307));
#83106=CARTESIAN_POINT('Ctrl Pts',(-3.8594617959262,-9.08779972523566,4.9087105172242));
#83107=CARTESIAN_POINT('Ctrl Pts',(-3.86933226327774,-9.07995068541308,
4.90782345834443));
#83108=CARTESIAN_POINT('Ctrl Pts',(-3.87578520446725,-9.07481927769292,
4.90724353253354));
#83109=CARTESIAN_POINT('Ctrl Pts',(-3.88190505349891,-9.06948713729174,
4.90661977297618));
#83110=CARTESIAN_POINT('Ctrl Pts',(-3.88770139233235,-9.0639990067157,4.90595898381691));
#83111=CARTESIAN_POINT('Ctrl Pts',(-3.89503262347501,-9.05705759853542,
4.90512321520462));
#83112=CARTESIAN_POINT('Ctrl Pts',(-3.90184468314376,-9.0498682586582,4.90422830374491));
#83113=CARTESIAN_POINT('Ctrl Pts',(-3.90816884420435,-9.04251720447913,
4.90330690801195));
#83114=CARTESIAN_POINT('Ctrl Pts',(-3.91133092473464,-9.0388416773896,4.90284621014547));
#83115=CARTESIAN_POINT('Ctrl Pts',(-3.91436903980901,-9.03512384425042,
4.90237127730828));
#83116=CARTESIAN_POINT('Ctrl Pts',(-3.9172869481511,-9.03137248254924,4.90188194411826));
#83117=CARTESIAN_POINT('Ctrl Pts',(-3.91874590232215,-9.02949680169865,
4.90163727752325));
#83118=CARTESIAN_POINT('Ctrl Pts',(-3.92017480408882,-9.02761274156667,
4.90138901495576));
#83119=CARTESIAN_POINT('Ctrl Pts',(-3.92157419015545,-9.02572141015965,
4.90113729933359));
#83120=CARTESIAN_POINT('Ctrl Pts',(-3.92238337566387,-9.0246277605924,4.90099174648113));
#83121=CARTESIAN_POINT('Ctrl Pts',(-3.92290954425151,-9.02390648865029,
4.90089521932563));
#83122=CARTESIAN_POINT('Ctrl Pts',(-3.92362915257453,-9.02291017871459,
4.90076221167712));
#83123=CARTESIAN_POINT('Ctrl Pts',(-3.92415401767594,-9.0221834940742,4.90066519907917));
#83124=CARTESIAN_POINT('Ctrl Pts',(-3.92478177136042,-9.0213104522166,4.90054877457427));
#83125=CARTESIAN_POINT('Ctrl Pts',(-3.9256856428377,-9.02002767016122,4.90037663508057));
#83126=CARTESIAN_POINT('Ctrl Pts',(-3.93076928149868,-9.01281292712051,
4.8994084720095));
#83127=CARTESIAN_POINT('Ctrl Pts',(-3.93546808728794,-9.0054636078729,4.89838345132082));
#83128=CARTESIAN_POINT('Ctrl Pts',(-3.93981071245734,-8.99801619371013,
4.89730809585987));
#83129=CARTESIAN_POINT('Ctrl Pts',(-3.94482881368225,-8.98941036735518,
4.89606547363361));
#83130=CARTESIAN_POINT('Ctrl Pts',(-3.9493701033765,-8.98067630776327,4.89475285872136));
#83131=CARTESIAN_POINT('Ctrl Pts',(-3.95347304747733,-8.9718716535676,4.8933511552548));
#83132=CARTESIAN_POINT('Ctrl Pts',(-3.95830199337999,-8.96150904619162,
4.89170142519629));
#83133=CARTESIAN_POINT('Ctrl Pts',(-3.9625243731347,-8.95104726054702,4.88992847546876));
#83134=CARTESIAN_POINT('Ctrl Pts',(-3.96622543769305,-8.94053252013442,
4.88804954732827));
#83135=CARTESIAN_POINT('Ctrl Pts',(-3.97105362982472,-8.92681560541267,
4.88559840768431));
#83136=CARTESIAN_POINT('Ctrl Pts',(-3.97499639173049,-8.91300578021216,
4.88296736034851));
#83137=CARTESIAN_POINT('Ctrl Pts',(-3.97825803337248,-8.89916845917825,
4.88026821014047));
#83138=CARTESIAN_POINT('Ctrl Pts',(-3.98093354530121,-8.8878177586564,4.87805410774305));
#83139=CARTESIAN_POINT('Ctrl Pts',(-3.98315132864282,-8.87644764305007,
4.87579638200634));
#83140=CARTESIAN_POINT('Ctrl Pts',(-3.98501607995159,-8.8650995212513,4.87357227374489));
#83141=CARTESIAN_POINT('Ctrl Pts',(-3.98704683592159,-8.85274116226647,
4.87115016999914));
#83142=CARTESIAN_POINT('Ctrl Pts',(-3.98865981875432,-8.84041605363061,
4.86876464610217));
#83143=CARTESIAN_POINT('Ctrl Pts',(-3.98998120246124,-8.82802685533874,
4.86648143874877));
#83144=CARTESIAN_POINT('Ctrl Pts',(-3.99138671146833,-8.81484890430245,
4.86405287202475));
#83145=CARTESIAN_POINT('Ctrl Pts',(-3.99246174015616,-8.80159798477713,
4.86173834904854));
#83146=CARTESIAN_POINT('Ctrl Pts',(-3.99330779305355,-8.78813311929187,
4.85962424523925));
#83147=CARTESIAN_POINT('Ctrl Pts',(-3.99408249088382,-8.77580386410155,
4.85768844236086));
#83148=CARTESIAN_POINT('Ctrl Pts',(-3.99466399994344,-8.76329376004554,
4.85591896163928));
#83149=CARTESIAN_POINT('Ctrl Pts',(-3.99510413495378,-8.75049000131564,
4.85441263397948));
#83150=CARTESIAN_POINT('Ctrl Pts',(-3.99546774267706,-8.73991246157952,
4.85316821497618));
#83151=CARTESIAN_POINT('Ctrl Pts',(-3.99573425864729,-8.72913360479011,
4.8521030453621));
#83152=CARTESIAN_POINT('Ctrl Pts',(-3.99592511106015,-8.71810107884211,
4.85130447744043));
#83153=CARTESIAN_POINT('Ctrl Pts',(-3.9960232071946,-8.71243047645101,4.85089402192122));
#83154=CARTESIAN_POINT('Ctrl Pts',(-3.99610122682654,-8.70669311547007,
4.85055459128874));
#83155=CARTESIAN_POINT('Ctrl Pts',(-3.99616169433912,-8.70088468227217,
4.8503029361967));
#83156=CARTESIAN_POINT('Ctrl Pts',(-3.7,-8.72799905369119,4.59960059693865));
#83157=CARTESIAN_POINT('Ctrl Pts',(-3.7,-9.02827749416229,4.63207689308604));
#83158=CARTESIAN_POINT('Ctrl Pts',(-3.7,-9.13925764782821,4.91297768894732));
#83159=CARTESIAN_POINT('Ctrl Pts',(-3.95543243018288,-8.72799905369119,
4.59960059693865));
#83160=CARTESIAN_POINT('Ctrl Pts',(-3.95543243018288,-9.02827749416229,
4.63207689308604));
#83161=CARTESIAN_POINT('Ctrl Pts',(-3.95543243018288,-9.13925764782821,
4.91297768894732));
#83162=CARTESIAN_POINT('Ctrl Pts',(-3.99616169476815,-8.70088460874173,
4.85030293093368));
#83163=CARTESIAN_POINT('Ctrl Pts',(-3.99616169476815,-8.84972402085523,
4.86640049963897));
#83164=CARTESIAN_POINT('Ctrl Pts',(-3.99616169476815,-8.90473370054448,
5.00563496899553));
#83165=CARTESIAN_POINT('Origin',(-3.7,-8.69574098918,4.89786125018));
#83166=CARTESIAN_POINT('Origin',(-3.7,-9.17423561284,0.47366156039));
#83167=CARTESIAN_POINT('',(-3.99951365747597,-8.00613534473186,4.74991749256093));
#83168=CARTESIAN_POINT('Ctrl Pts',(-3.99944937669,-8.31076354672,4.82056300746));
#83169=CARTESIAN_POINT('Ctrl Pts',(-3.99959839809,-8.28592729564,4.81813395331));
#83170=CARTESIAN_POINT('Ctrl Pts',(-3.99969341422,-8.26106714699,4.8150399126));
#83171=CARTESIAN_POINT('Ctrl Pts',(-3.99975395169,-8.23622932864,4.81128563568));
#83172=CARTESIAN_POINT('Ctrl Pts',(-3.99984876957,-8.17436353389,4.80027772376));
#83173=CARTESIAN_POINT('Ctrl Pts',(-3.99983052524,-8.11319387748,4.78525185918));
#83174=CARTESIAN_POINT('Ctrl Pts',(-3.99979379772,-8.07691196013,4.77482737361));
#83175=CARTESIAN_POINT('Ctrl Pts',(-3.99970844997,-8.04117830882,4.76303153489));
#83176=CARTESIAN_POINT('Ctrl Pts',(-3.99951367307,-8.00613533845,4.74991748836));
#83177=CARTESIAN_POINT('',(-4.,-6.41575007864,3.96554608849));
#83178=CARTESIAN_POINT('Ctrl Pts',(-3.99951362599666,-8.00613533213075,
4.74991748884671));
#83179=CARTESIAN_POINT('Ctrl Pts',(-3.99912775537927,-7.93670347374554,
4.72393400135952));
#83180=CARTESIAN_POINT('Ctrl Pts',(-3.99857222013012,-7.86774756468867,
4.69717811451172));
#83181=CARTESIAN_POINT('Ctrl Pts',(-3.99801113590394,-7.79918725181215,
4.66959751880907));
#83182=CARTESIAN_POINT('Ctrl Pts',(-3.99744761007927,-7.730328593788,4.64189690415447));
#83183=CARTESIAN_POINT('Ctrl Pts',(-3.99687800868216,-7.66186886095888,
4.61336445780402));
#83184=CARTESIAN_POINT('Ctrl Pts',(-3.99641199162889,-7.59372678110788,
4.58394586052179));
#83185=CARTESIAN_POINT('Ctrl Pts',(-3.99594125784065,-7.52489500947846,
4.55422950648306));
#83186=CARTESIAN_POINT('Ctrl Pts',(-3.995576066866,-7.45638723799201,4.52360898626897));
#83187=CARTESIAN_POINT('Ctrl Pts',(-3.99537650648205,-7.3881216373169,4.49202632379195));
#83188=CARTESIAN_POINT('Ctrl Pts',(-3.99518351319893,-7.32210250998592,
4.46148297846278));
#83189=CARTESIAN_POINT('Ctrl Pts',(-3.99514521891445,-7.25630980867474,
4.43003972020292));
#83190=CARTESIAN_POINT('Ctrl Pts',(-3.99526985343324,-7.19067264205082,
4.39764258740694));
#83191=CARTESIAN_POINT('Ctrl Pts',(-3.99539848691283,-7.12292947414796,
4.36420597642182));
#83192=CARTESIAN_POINT('Ctrl Pts',(-3.99570001270616,-7.05585580407319,
4.33000186128198));
#83193=CARTESIAN_POINT('Ctrl Pts',(-3.99612402104634,-6.98939603026552,
4.29503064588602));
#83194=CARTESIAN_POINT('Ctrl Pts',(-3.9965462561408,-6.92321419794775,4.26020568364672));
#83195=CARTESIAN_POINT('Ctrl Pts',(-3.99708992828748,-6.85764109095415,
4.22461998892733));
#83196=CARTESIAN_POINT('Ctrl Pts',(-3.99765401687659,-6.79262048515617,
4.18827520267667));
#83197=CARTESIAN_POINT('Ctrl Pts',(-3.99820754909831,-6.72881667653507,
4.1526105736279));
#83198=CARTESIAN_POINT('Ctrl Pts',(-3.998780787767,-6.66554485798596,4.11621493441839));
#83199=CARTESIAN_POINT('Ctrl Pts',(-3.99922880371063,-6.60275116879257,
4.07909177039002));
#83200=CARTESIAN_POINT('Ctrl Pts',(-3.99967681965425,-6.53995747959918,
4.04196860636165));
#83201=CARTESIAN_POINT('Ctrl Pts',(-4.,-6.47764191894906,4.00411781442964));
#83202=CARTESIAN_POINT('Ctrl Pts',(-4.,-6.41575007864,3.96554608849));
#83203=CARTESIAN_POINT('Origin',(-4.,-9.17423561284,0.47366156039));
#83204=CARTESIAN_POINT('Ctrl Pts',(-4.29889876134,-8.31430322282,5.1027434229));
#83205=CARTESIAN_POINT('Ctrl Pts',(-4.2082233452,-8.31323138881,5.10274342246));
#83206=CARTESIAN_POINT('Ctrl Pts',(-4.11754792907,-8.31215955225,5.0684801702));
#83207=CARTESIAN_POINT('Ctrl Pts',(-4.04442177042,-8.31129515513,4.99957114081));
#83208=CARTESIAN_POINT('Ctrl Pts',(-4.00483538997,-8.31082721545,4.91108469399));
#83209=CARTESIAN_POINT('Ctrl Pts',(-3.99944937087,-8.31076354298,4.8205630482));
#83210=CARTESIAN_POINT('Ctrl Pts',(-4.29964314059,-8.22434260602,5.1027436292));
#83211=CARTESIAN_POINT('Ctrl Pts',(-4.20780699632,-8.22403023518,5.10264720521));
#83212=CARTESIAN_POINT('Ctrl Pts',(-4.11597085206,-8.22680019636,5.06741723002));
#83213=CARTESIAN_POINT('Ctrl Pts',(-4.0423682592,-8.23275280902,4.99666339283));
#83214=CARTESIAN_POINT('Ctrl Pts',(-4.00353912359,-8.24059165767,4.90627699718));
#83215=CARTESIAN_POINT('Ctrl Pts',(-3.99982155439,-8.24873700866,4.81449657867));
#83216=CARTESIAN_POINT('Ctrl Pts',(-4.29971371834,-8.13469356333,5.09262744205));
#83217=CARTESIAN_POINT('Ctrl Pts',(-4.20724144925,-8.13466365636,5.09260573663));
#83218=CARTESIAN_POINT('Ctrl Pts',(-4.11476918016,-8.14098347585,5.05729879766));
#83219=CARTESIAN_POINT('Ctrl Pts',(-4.04093270982,-8.15373242653,4.98629044613));
#83220=CARTESIAN_POINT('Ctrl Pts',(-4.00258694952,-8.1700271987,4.89579754059));
#83221=CARTESIAN_POINT('Ctrl Pts',(-3.99985686503,-8.18656139935,4.80428277208));
#83222=CARTESIAN_POINT('Ctrl Pts',(-4.29971786827,-8.04665414995,5.07253279403));
#83223=CARTESIAN_POINT('Ctrl Pts',(-4.20720101416,-8.04666571693,5.07252348963));
#83224=CARTESIAN_POINT('Ctrl Pts',(-4.11468416006,-8.05626571803,5.0379315222));
#83225=CARTESIAN_POINT('Ctrl Pts',(-4.04083150668,-8.07556834767,4.96834669024));
#83226=CARTESIAN_POINT('Ctrl Pts',(-4.00251997495,-8.10013935979,4.87966809703));
#83227=CARTESIAN_POINT('Ctrl Pts',(-3.9998589855,-8.12494698597,4.78999433407));
#83228=CARTESIAN_POINT('Ctrl Pts',(-4.29967705707,-7.96150927709,5.0427549913));
#83229=CARTESIAN_POINT('Ctrl Pts',(-4.20771171282,-7.96176972051,5.0427867655));
#83230=CARTESIAN_POINT('Ctrl Pts',(-4.11574636857,-7.97452633141,5.00973042736));
#83231=CARTESIAN_POINT('Ctrl Pts',(-4.04209470673,-7.99987188278,4.94319135382));
#83232=CARTESIAN_POINT('Ctrl Pts',(-4.00335979512,-8.03206135592,4.85814590158));
#83233=CARTESIAN_POINT('Ctrl Pts',(-3.99983852853,-8.06458049923,4.77178934946));
#83234=CARTESIAN_POINT('Ctrl Pts',(-4.29902733552,-7.88049121843,5.00374669681));
#83235=CARTESIAN_POINT('Ctrl Pts',(-4.20814475196,-7.88133646016,5.00415366088));
#83236=CARTESIAN_POINT('Ctrl Pts',(-4.1172621684,-7.89711301226,4.97354912353));
#83237=CARTESIAN_POINT('Ctrl Pts',(-4.04405132352,-7.92782452293,4.91150502168));
#83238=CARTESIAN_POINT('Ctrl Pts',(-4.00460096887,-7.96672185729,4.83165611315));
#83239=CARTESIAN_POINT('Ctrl Pts',(-3.99951366776,-8.00613540701,4.74991741048));
#83240=CARTESIAN_POINT('Origin',(-4.29708374629736,-8.00976110076321,4.73530658527947));
#83241=CARTESIAN_POINT('Ctrl Pts',(-4.2990272509,-7.88049121843,5.00374669681));
#83242=CARTESIAN_POINT('Ctrl Pts',(-4.20814466399,-7.88133645067,5.00415365756));
#83243=CARTESIAN_POINT('Ctrl Pts',(-4.11726207707,-7.8971129981,4.97354910689));
#83244=CARTESIAN_POINT('Ctrl Pts',(-4.04405123536,-7.92782451085,4.91150498201));
#83245=CARTESIAN_POINT('Ctrl Pts',(-4.00460089543,-7.96672185122,4.83165605064));
#83246=CARTESIAN_POINT('Ctrl Pts',(-3.99951361632,-8.0061354071,4.74991733337));
#83247=CARTESIAN_POINT('Ctrl Pts',(-4.29534152276,-7.55873090479,4.8488266546));
#83248=CARTESIAN_POINT('Ctrl Pts',(-4.21089110293,-7.56075677108,4.84980205594));
#83249=CARTESIAN_POINT('Ctrl Pts',(-4.12644068311,-7.57560508753,4.82414594128));
#83250=CARTESIAN_POINT('Ctrl Pts',(-4.05583695285,-7.60300935451,4.77146524893));
#83251=CARTESIAN_POINT('Ctrl Pts',(-4.01210473647,-7.6379921895,4.70122601239));
#83252=CARTESIAN_POINT('Ctrl Pts',(-3.99767078695,-7.67454601586,4.62582683568));
#83253=CARTESIAN_POINT('Ctrl Pts',(-4.28495419985,-7.24223776902,4.69644263496));
#83254=CARTESIAN_POINT('Ctrl Pts',(-4.20364197507,-7.24265108624,4.69664162775));
#83255=CARTESIAN_POINT('Ctrl Pts',(-4.12232975028,-7.25504442659,4.67195877864));
#83256=CARTESIAN_POINT('Ctrl Pts',(-4.05372035815,-7.27955010958,4.62221233106));
#83257=CARTESIAN_POINT('Ctrl Pts',(-4.00967965098,-7.31194178404,4.55622127864));
#83258=CARTESIAN_POINT('Ctrl Pts',(-3.99247722227,-7.34677145748,4.48508959035));
#83259=CARTESIAN_POINT('Ctrl Pts',(-4.28719359971,-6.92729615453,4.54480563642));
#83260=CARTESIAN_POINT('Ctrl Pts',(-4.20516486744,-6.92619358841,4.54427477668));
#83261=CARTESIAN_POINT('Ctrl Pts',(-4.12313613516,-6.93728087775,4.51842626492));
#83262=CARTESIAN_POINT('Ctrl Pts',(-4.05411385932,-6.96067605503,4.46706057541));
#83263=CARTESIAN_POINT('Ctrl Pts',(-4.01020087277,-6.99204699421,4.39931666036));
#83264=CARTESIAN_POINT('Ctrl Pts',(-3.99359726714,-7.02607103842,4.32667666396));
#83265=CARTESIAN_POINT('Ctrl Pts',(-4.3,-6.60947733541,4.39178333134));
#83266=CARTESIAN_POINT('Ctrl Pts',(-4.21340350799,-6.60705721212,4.39061809876));
#83267=CARTESIAN_POINT('Ctrl Pts',(-4.12680701597,-6.61808600203,4.3615202213));
#83268=CARTESIAN_POINT('Ctrl Pts',(-4.0550389398,-6.64318599408,4.30449502667));
#83269=CARTESIAN_POINT('Ctrl Pts',(-4.01201861445,-6.67775474512,4.23026617343));
#83270=CARTESIAN_POINT('Ctrl Pts',(-4.,-6.71532134284,4.1522424388));
#83271=CARTESIAN_POINT('Ctrl Pts',(-4.3,-6.28560647753,4.2358471116));
#83272=CARTESIAN_POINT('Ctrl Pts',(-4.20575222039,-6.28560647753,4.2358471116));
#83273=CARTESIAN_POINT('Ctrl Pts',(-4.11150444078,-6.30166230076,4.20250005951));
#83274=CARTESIAN_POINT('Ctrl Pts',(-4.0370110165,-6.33397844241,4.13538123018));
#83275=CARTESIAN_POINT('Ctrl Pts',(-4.,-6.37486426052,4.05046365934));
#83276=CARTESIAN_POINT('Ctrl Pts',(-4.,-6.41575007864,3.96554608849));
#83277=CARTESIAN_POINT('Origin',(-4.29787865889067,-6.41482978920342,3.96745741146091));
#83278=CARTESIAN_POINT('Origin',(-4.3,-2.74845588872,2.19982997428));
#83279=CARTESIAN_POINT('',(-4.,-4.55379688725,3.06905931004));
#83280=CARTESIAN_POINT('Origin',(-4.,0.,0.));
#98285=UNCERTAINTY_MEASURE_WITH_UNIT(LENGTH_MEASURE(0.01),#98303,
'DISTANCE_ACCURACY_VALUE',
'Maximum model space distance between geometric entities at asserted c
onnectivities');
#98290=UNCERTAINTY_MEASURE_WITH_UNIT(LENGTH_MEASURE(0.01),#98303,
'DISTANCE_ACCURACY_VALUE',
'Maximum model space distance between geometric entities at asserted c
onnectivities');
#98297=(
GEOMETRIC_REPRESENTATION_CONTEXT(3)
GLOBAL_UNCERTAINTY_ASSIGNED_CONTEXT((#98285))
GLOBAL_UNIT_ASSIGNED_CONTEXT((#98303,#98305,#98306))
REPRESENTATION_CONTEXT('','3D')
);
#98302=(
GEOMETRIC_REPRESENTATION_CONTEXT(3)
GLOBAL_UNCERTAINTY_ASSIGNED_CONTEXT((#98290))
GLOBAL_UNIT_ASSIGNED_CONTEXT((#98303,#98305,#98306))
REPRESENTATION_CONTEXT('','3D')
);
#98303=(
LENGTH_UNIT()
NAMED_UNIT(*)
SI_UNIT(.MILLI.,.METRE.)
);
#98305=(
NAMED_UNIT(*)
PLANE_ANGLE_UNIT()
SI_UNIT($,.RADIAN.)
);
#98306=(
NAMED_UNIT(*)
SI_UNIT($,.STERADIAN.)
SOLID_ANGLE_UNIT()
);
#98313=SHAPE_DEFINITION_REPRESENTATION(#98324,#98345);
#98324=PRODUCT_DEFINITION_SHAPE('',$,#98357);
#98345=SHAPE_REPRESENTATION('',(#35726),#98297);
#98350=PRODUCT_DEFINITION_CONTEXT('part definition',#98385,'design');
#98357=PRODUCT_DEFINITION('Control Lever','Control Lever',#98368,#98350);
#98368=PRODUCT_DEFINITION_FORMATION('',$,#98393);
#98385=APPLICATION_CONTEXT(
'Core Data for Automotive Mechanical Design Process');
#98386=PRODUCT_CONTEXT('part definition',#98385,'mechanical');
#98393=PRODUCT('Control Lever','Control Lever',$,(#98386));
#98399=PRESENTATION_STYLE_ASSIGNMENT((#98401));
#98401=SURFACE_STYLE_USAGE(.BOTH.,#98403);
#98403=SURFACE_SIDE_STYLE('',(#98405));
#98405=SURFACE_STYLE_FILL_AREA(#98407);
#98407=FILL_AREA_STYLE('Opaque(202,209,238)',(#98409));
#98409=FILL_AREA_STYLE_COLOUR('Opaque(202,209,238)',#98411);
#98411=COLOUR_RGB('Opaque(202,209,238)', 0.31764706, 0.68627451, 0.89019608);
ENDSEC;
END-ISO-10303-21;
